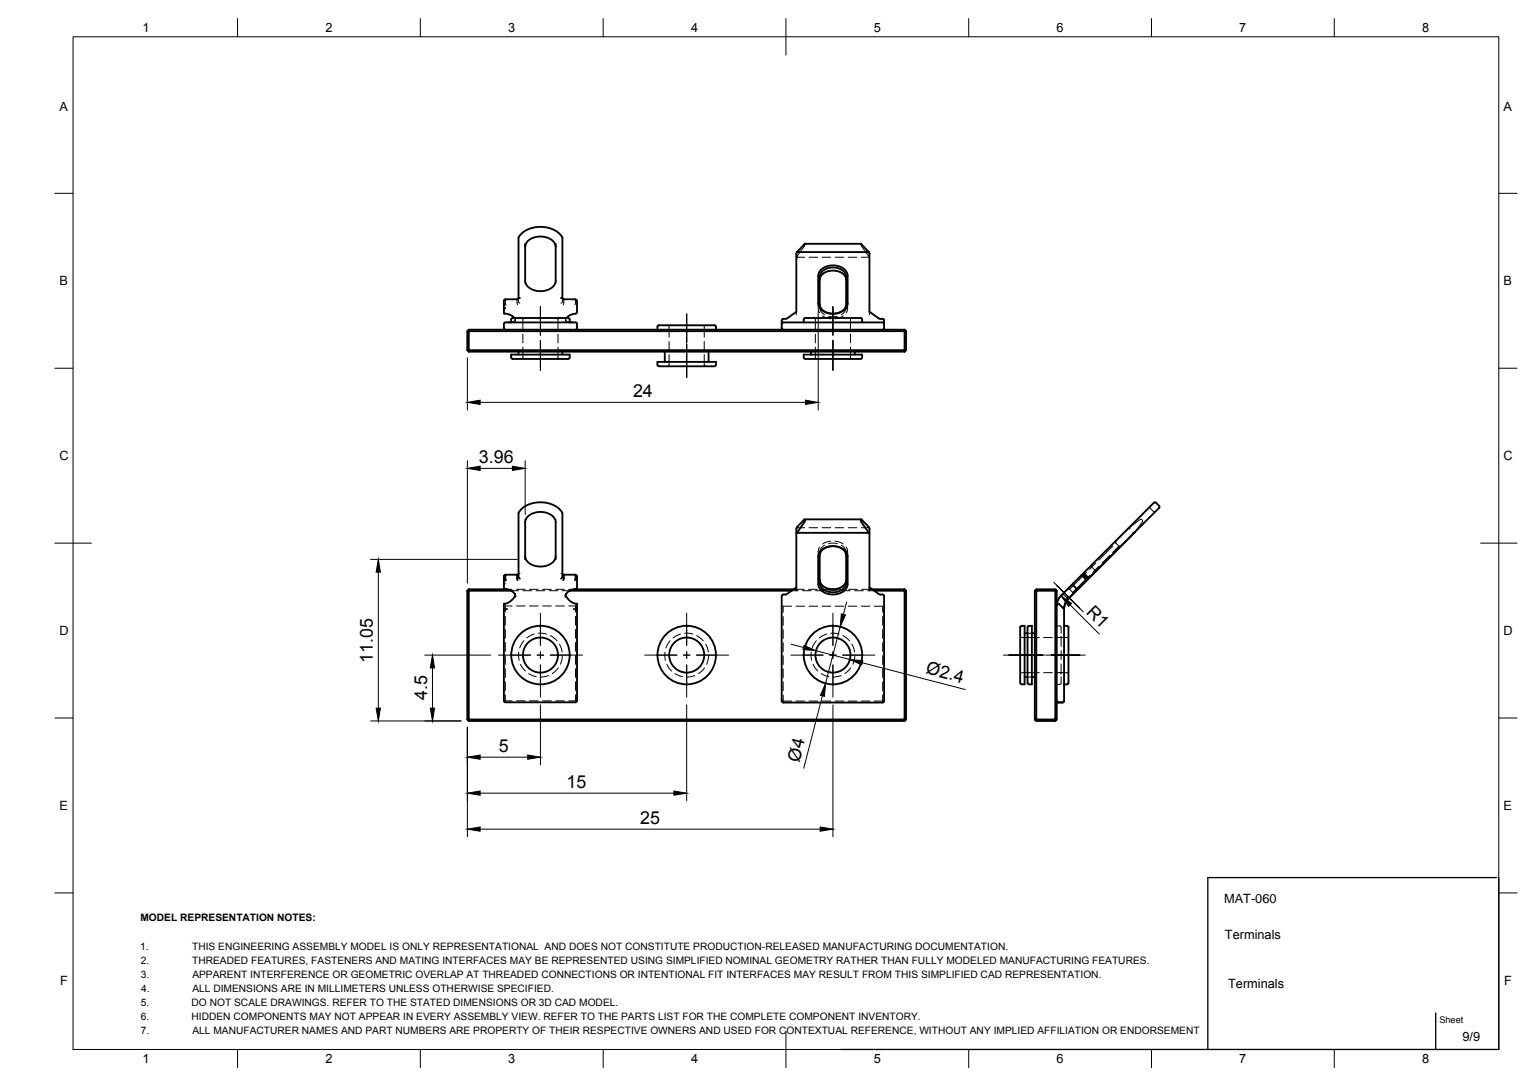
ISO-10303-21;
HEADER;
FILE_DESCRIPTION (('STEP AP214'),
    '1' );
FILE_NAME ('Terminals.step',
    '2026-10-29T23:46:56',
    ( '' ),
    ( '' ),
    'SwSTEP 2.0',
    'SolidWorks 2020',
    '' );
FILE_SCHEMA (( 'AUTOMOTIVE_DESIGN' ));
ENDSEC;

DATA;
#17=AXIS2_PLACEMENT_3D ( 'NONE', #6109, #14151, #26614 ) ;
#19=AXIS2_PLACEMENT_3D ( 'NONE', #29892, #26933, #14470 ) ;
#20=EDGE_LOOP ( 'NONE', ( #20639, #20304, #9074, #30153 ) ) ;
#22=DIRECTION ( 'NONE',  ( 7.588956326749211550E-18, -4.206627182996911684E-18, 1.000000000000000000 ) ) ;
#27=DIRECTION ( 'NONE',  ( 0.9612616959383206705, 0.2756373558169926130, 8.795445018804289444E-19 ) ) ;
#28=FACE_OUTER_BOUND ( 'NONE', #27332, .T. ) ;
#29=CARTESIAN_POINT ( 'NONE',  ( -42.41019933908752648, 14.71530103803245915, 55.14139656020049785 ) ) ;
#36=DIRECTION ( 'NONE',  ( 0.9612616959383191162, 0.2756373558169986082, 8.795445018805098335E-19 ) ) ;
#38=FACE_OUTER_BOUND ( 'NONE', #16032, .T. ) ;
#41=AXIS2_PLACEMENT_3D ( 'NONE', #1077, #13253, #30795 ) ;
#52=EDGE_LOOP ( 'NONE', ( #4319, #21732, #2975, #7082 ) ) ;
#54=CARTESIAN_POINT ( 'NONE',  ( -41.75126335834794133, 15.45321085637654690, 35.55750462089839203 ) ) ;
#56=ORIENTED_EDGE ( 'NONE', *, *, #16072, .T. ) ;
#57=CARTESIAN_POINT ( 'NONE',  ( -40.99628586177130529, 8.927770518203464789, 58.05249952744806308 ) ) ;
#66=ORIENTED_EDGE ( 'NONE', *, *, #7414, .F. ) ;
#68=FACE_OUTER_BOUND ( 'NONE', #23592, .T. ) ;
#69=CARTESIAN_POINT ( 'NONE',  ( -40.69193635511749108, 9.347952559758585522, 39.44930799450052206 ) ) ;
#72=CARTESIAN_POINT ( 'NONE',  ( -40.77849034781615956, 8.435947495041027366, 34.55508635502627612 ) ) ;
#75=CARTESIAN_POINT ( 'NONE',  ( -40.75848109938849717, 9.580021662090986823, 38.54930799450052348 ) ) ;
#76=DIRECTION ( 'NONE',  ( 0.4848096202463429982, 0.8746197071393925215, 9.920727850371698576E-18 ) ) ;
#77=ORIENTED_EDGE ( 'NONE', *, *, #10123, .F. ) ;
#82=CARTESIAN_POINT ( 'NONE',  ( -39.58809650894544774, 2.596771453999702661, 45.04930799450051637 ) ) ;
#90=VERTEX_POINT ( 'NONE', #16171 ) ;
#101=LINE ( 'NONE', #30305, #23466 ) ;
#103=ORIENTED_EDGE ( 'NONE', *, *, #27267, .F. ) ;
#108=DIRECTION ( 'NONE',  ( 0.9612616959383206705, 0.2756373558169926130, 8.795445018804289444E-19 ) ) ;
#110=VERTEX_POINT ( 'NONE', #16495 ) ;
#115=VECTOR ( 'NONE', #2052, 999.9999999999998863 ) ;
#118=SPHERICAL_SURFACE ( 'NONE', #22577, 0.1000000000000000056 ) ;
#123=EDGE_CURVE ( 'NONE', #13895, #2732, #897, .T. ) ;
#136=FACE_OUTER_BOUND ( 'NONE', #14776, .T. ) ;
#137=ORIENTED_EDGE ( 'NONE', *, *, #30547, .F. ) ;
#149=AXIS2_PLACEMENT_3D ( 'NONE', #13743, #23739, #24058 ) ;
#153=ORIENTED_EDGE ( 'NONE', *, *, #20856, .F. ) ;
#155=VERTEX_POINT ( 'NONE', #13728 ) ;
#156=CARTESIAN_POINT ( 'NONE',  ( -40.54018958231235814, 7.005332542891154368, 35.02307665165292150 ) ) ;
#158=CARTESIAN_POINT ( 'NONE',  ( -40.76199410932685652, 8.110698076655893374, 59.50788663826320146 ) ) ;
#168=VECTOR ( 'NONE', #18188, 1000.000000000000114 ) ;
#171=AXIS2_PLACEMENT_3D ( 'NONE', #9638, #108, #19631 ) ;
#175=DIRECTION ( 'NONE',  ( 0.3958453973320085195, 0.7141240004913234074, 0.5773502691896251759 ) ) ;
#179=EDGE_CURVE ( 'NONE', #22338, #15550, #10168, .T. ) ;
#180=VERTEX_POINT ( 'NONE', #22065 ) ;
#184=DIRECTION ( 'NONE',  ( 0.8746197071393858602, -0.4848096202463547666, 0.000000000000000000 ) ) ;
#187=ORIENTED_EDGE ( 'NONE', *, *, #28945, .F. ) ;
#188=AXIS2_PLACEMENT_3D ( 'NONE', #771, #25875, #3057 ) ;
#192=DIRECTION ( 'NONE',  ( -0.9612616959383207815, -0.2756373558169926685, -8.795445018804289444E-19 ) ) ;
#195=CARTESIAN_POINT ( 'NONE',  ( -42.67844523361456766, 15.18734573188464765, 35.55750462089839203 ) ) ;
#196=CIRCLE ( 'NONE', #709, 0.8928932188134561798 ) ;
#197=DIRECTION ( 'NONE',  ( -0.9612616959383183390, -0.2756373558170014948, -8.795445018805493151E-19 ) ) ;
#209=DIRECTION ( 'NONE',  ( 0.2756373558169961657, -0.9612616959383196713, -2.918609477355923238E-15 ) ) ;
#211=CARTESIAN_POINT ( 'NONE',  ( -43.29088418437023478, 1.073429008971243270, 39.44930799450052916 ) ) ;
#218=LINE ( 'NONE', #12381, #10663 ) ;
#225=ORIENTED_EDGE ( 'NONE', *, *, #23042, .T. ) ;
#229=VERTEX_POINT ( 'NONE', #19763 ) ;
#232=CARTESIAN_POINT ( 'NONE',  ( -40.60333149162104860, 7.557375771971046596, 56.04611646155296256 ) ) ;
#240=CARTESIAN_POINT ( 'NONE',  ( -40.59758774925371938, 7.567737757495682338, 34.64930799450051779 ) ) ;
#249=ORIENTED_EDGE ( 'NONE', *, *, #29875, .T. ) ;
#250=DIRECTION ( 'NONE',  ( -0.9612616959383205595, -0.2756373558169929461, 1.660411357259281952E-16 ) ) ;
#261=TOROIDAL_SURFACE ( 'NONE', #15443, 0.2000000000000000111, 0.1000000000000000056 ) ;
#271=DIRECTION ( 'NONE',  ( -0.2756373558170082672, 0.9612616959383162296, 0.000000000000000000 ) ) ;
#280=DIRECTION ( 'NONE',  ( -0.8746197071393927436, 0.4848096202463423876, 1.277302113040827440E-17 ) ) ;
#283=TOROIDAL_SURFACE ( 'NONE', #21230, 1.142135311067127068, 0.1000000000000000056 ) ;
#284=CARTESIAN_POINT ( 'NONE',  ( -40.04869510400508403, 6.988917179839018168, 35.05065200723174001 ) ) ;
#286=VERTEX_POINT ( 'NONE', #26777 ) ;
#289=ORIENTED_EDGE ( 'NONE', *, *, #14454, .T. ) ;
#290=VECTOR ( 'NONE', #23726, 1000.000000000000114 ) ;
#292=PLANE ( 'NONE',  #4320 ) ;
#301=ADVANCED_FACE ( 'NONE', ( #4126 ), #31709, .T. ) ;
#311=ORIENTED_EDGE ( 'NONE', *, *, #27048, .T. ) ;
#317=DIRECTION ( 'NONE',  ( 2.946248497964555786E-19, 3.001156285468303092E-19, 1.000000000000000000 ) ) ;
#318=CARTESIAN_POINT ( 'NONE',  ( -40.58856461370174884, 7.499380836222963254, 53.94930799450052206 ) ) ;
#328=CYLINDRICAL_SURFACE ( 'NONE', #6747, 0.1000000000000020595 ) ;
#342=DIRECTION ( 'NONE',  ( 0.4848096202463636484, 0.8746197071393810862, 0.000000000000000000 ) ) ;
#356=ORIENTED_EDGE ( 'NONE', *, *, #17245, .T. ) ;
#357=CYLINDRICAL_SURFACE ( 'NONE', #3440, 2.000000000000001776 ) ;
#361=LINE ( 'NONE', #25479, #15657 ) ;
#365=FACE_OUTER_BOUND ( 'NONE', #31359, .T. ) ;
#367=ORIENTED_EDGE ( 'NONE', *, *, #20650, .T. ) ;
#372=CYLINDRICAL_SURFACE ( 'NONE', #24107, 0.1000000000000012962 ) ;
#376=ORIENTED_EDGE ( 'NONE', *, *, #20856, .T. ) ;
#382=VERTEX_POINT ( 'NONE', #1667 ) ;
#383=LINE ( 'NONE', #20407, #27548 ) ;
#384=VECTOR ( 'NONE', #5115, 1000.000000000000114 ) ;
#390=ORIENTED_EDGE ( 'NONE', *, *, #15587, .T. ) ;
#395=CARTESIAN_POINT ( 'NONE',  ( -37.58300281841709989, 16.01180101885526597, 37.04930799450052348 ) ) ;
#400=CARTESIAN_POINT ( 'NONE',  ( -40.68422973805265030, 6.807290781432339344, 39.32248954417796227 ) ) ;
#407=EDGE_CURVE ( 'NONE', #2291, #14081, #6151, .T. ) ;
#411=ADVANCED_FACE ( 'NONE', ( #1587 ), #6674, .T. ) ;
#413=CARTESIAN_POINT ( 'NONE',  ( -40.08841711228579641, 7.575633567407562552, 60.54930799450051637 ) ) ;
#423=CARTESIAN_POINT ( 'NONE',  ( -40.11967773290336226, 9.763195579837789850, 38.54930799450052348 ) ) ;
#424=ORIENTED_EDGE ( 'NONE', *, *, #23042, .F. ) ;
#433=DIRECTION ( 'NONE',  ( -0.8746197071393805311, 0.4848096202463645921, 8.676864087101954631E-18 ) ) ;
#437=EDGE_CURVE ( 'NONE', #1880, #13059, #22878, .T. ) ;
#438=LINE ( 'NONE', #30167, #5287 ) ;
#451=CARTESIAN_POINT ( 'NONE',  ( -40.90015969217747482, 8.955334253785164123, 57.04930799450051637 ) ) ;
#452=VECTOR ( 'NONE', #29063, 1000.000000000000000 ) ;
#466=DIRECTION ( 'NONE',  ( 0.000000000000000000, 0.000000000000000000, -1.000000000000000000 ) ) ;
#471=ORIENTED_EDGE ( 'NONE', *, *, #842, .F. ) ;
#472=DIRECTION ( 'NONE',  ( -0.8746197071393926326, 0.4848096202463430537, 8.676864087101709653E-18 ) ) ;
#479=DIRECTION ( 'NONE',  ( -0.9612616959383175619, -0.2756373558170036597, -8.795445018805799373E-19 ) ) ;
#480=ORIENTED_EDGE ( 'NONE', *, *, #9764, .F. ) ;
#482=EDGE_CURVE ( 'NONE', #26626, #155, #15829, .T. ) ;
#491=AXIS2_PLACEMENT_3D ( 'NONE', #9371, #11504, #4285 ) ;
#493=ORIENTED_EDGE ( 'NONE', *, *, #32444, .F. ) ;
#495=ORIENTED_EDGE ( 'NONE', *, *, #28799, .T. ) ;
#497=CIRCLE ( 'NONE', #8889, 0.1000000000000018235 ) ;
#503=DIRECTION ( 'NONE',  ( 0.2756373558169932236, -0.9612616959383206705, 3.214564189377567398E-15 ) ) ;
#504=FACE_OUTER_BOUND ( 'NONE', #24476, .T. ) ;
#507=DIRECTION ( 'NONE',  ( -0.8746197071393926326, 0.4848096202463430537, 8.676864087101709653E-18 ) ) ;
#508=FACE_OUTER_BOUND ( 'NONE', #6579, .T. ) ;
#513=ORIENTED_EDGE ( 'NONE', *, *, #26307, .F. ) ;
#527=CARTESIAN_POINT ( 'NONE',  ( -40.19935072163752210, 7.013056605096603668, 39.22629476879045285 ) ) ;
#534=AXIS2_PLACEMENT_3D ( 'NONE', #12377, #29269, #2022 ) ;
#550=EDGE_CURVE ( 'NONE', #4992, #17225, #25775, .T. ) ;
#551=AXIS2_PLACEMENT_3D ( 'NONE', #843, #30240, #2664 ) ;
#557=CARTESIAN_POINT ( 'NONE',  ( -40.69574609830256406, 6.786514717574567257, 39.44982113259668211 ) ) ;
#560=FACE_OUTER_BOUND ( 'NONE', #13717, .T. ) ;
#561=AXIS2_PLACEMENT_3D ( 'NONE', #7178, #14738, #4059 ) ;
#563=CARTESIAN_POINT ( 'NONE',  ( -40.11286833322907341, 2.887657226147505973, 35.84930799450052064 ) ) ;
#564=DIRECTION ( 'NONE',  ( -2.779292025043186357E-18, 1.288349127009862211E-17, -1.000000000000000000 ) ) ;
#569=CARTESIAN_POINT ( 'NONE',  ( -40.29992972011127961, 7.980862958756435255, 40.07149053519532345 ) ) ;
#577=AXIS2_PLACEMENT_3D ( 'NONE', #24916, #30008, #25240 ) ;
#584=AXIS2_PLACEMENT_3D ( 'NONE', #31750, #4338, #1712 ) ;
#585=ADVANCED_FACE ( 'NONE', ( #17503 ), #25657, .T. ) ;
#586=CARTESIAN_POINT ( 'NONE',  ( -40.39697993529618714, 8.288924485351975235, 59.57859731638185963 ) ) ;
#589=EDGE_CURVE ( 'NONE', #28974, #110, #24896, .T. ) ;
#591=ORIENTED_EDGE ( 'NONE', *, *, #5712, .T. ) ;
#594=EDGE_CURVE ( 'NONE', #3250, #802, #20731, .T. ) ;
#596=CIRCLE ( 'NONE', #27333, 0.1000000000000016709 ) ;
#600=CIRCLE ( 'NONE', #24713, 1.199999999999999734 ) ;
#601=ORIENTED_EDGE ( 'NONE', *, *, #27122, .F. ) ;
#607=VERTEX_POINT ( 'NONE', #27519 ) ;
#614=CARTESIAN_POINT ( 'NONE',  ( -40.46704362897354201, 7.411062716778210380, 35.30013894732506685 ) ) ;
#615=ORIENTED_EDGE ( 'NONE', *, *, #10584, .T. ) ;
#626=EDGE_CURVE ( 'NONE', #32106, #27773, #16758, .T. ) ;
#640=DIRECTION ( 'NONE',  ( -2.779292025043186357E-18, 1.288349127009862211E-17, -1.000000000000000000 ) ) ;
#651=B_SPLINE_CURVE_WITH_KNOTS ( 'NONE', 3,
 ( #1890, #31770, #9282, #29302, #27005, #12076, #21904, #22069 ),
 .UNSPECIFIED., .F., .F.,
 ( 4, 2, 2, 4 ),
 ( 0.000000000000000000, 0.0005021167140330338053, 0.0007531750710495593816, 0.001004233428066084958 ),
 .UNSPECIFIED. ) ;
#652=DIRECTION ( 'NONE',  ( -0.9612616959383221138, -0.2756373558169876170, 0.000000000000000000 ) ) ;
#655=VERTEX_POINT ( 'NONE', #26463 ) ;
#656=DIRECTION ( 'NONE',  ( 7.588956326749211550E-18, -4.206627182996912454E-18, 1.000000000000000000 ) ) ;
#666=DIRECTION ( 'NONE',  ( 0.8746197071393925215, -0.4848096202463429982, -8.676864087101709653E-18 ) ) ;
#683=CARTESIAN_POINT ( 'NONE',  ( -43.64647580959332629, 1.256990871545142774, 53.54930799450051637 ) ) ;
#684=VECTOR ( 'NONE', #2246, 1000.000000000000000 ) ;
#685=CARTESIAN_POINT ( 'NONE',  ( -41.08785830660042393, 9.277514380576530328, 34.69072935073783981 ) ) ;
#688=CARTESIAN_POINT ( 'NONE',  ( -42.38687957179150345, 4.148162238788004608, 55.04930799450051637 ) ) ;
#697=LINE ( 'NONE', #20231, #30952 ) ;
#699=CARTESIAN_POINT ( 'NONE',  ( -43.38408989745150990, 1.111547985471239786, 60.54930799450051637 ) ) ;
#701=EDGE_LOOP ( 'NONE', ( #9890, #30769 ) ) ;
#707=EDGE_CURVE ( 'NONE', #18016, #21157, #8900, .T. ) ;
#709=AXIS2_PLACEMENT_3D ( 'NONE', #18125, #3351, #11077 ) ;
#718=DIRECTION ( 'NONE',  ( -0.1949050434465282311, 0.6797146636928673713, -0.7071067811865470176 ) ) ;
#720=DIRECTION ( 'NONE',  ( 0.000000000000000000, 0.000000000000000000, 1.000000000000000000 ) ) ;
#724=DIRECTION ( 'NONE',  ( -7.588956326749211550E-18, 4.206627182996912454E-18, -1.000000000000000000 ) ) ;
#725=ORIENTED_EDGE ( 'NONE', *, *, #20436, .T. ) ;
#728=DIRECTION ( 'NONE',  ( -0.4848096202463391680, -0.8746197071393946310, 0.000000000000000000 ) ) ;
#731=CARTESIAN_POINT ( 'NONE',  ( -40.56956524039852496, 6.944624558150293225, 39.15224832543683675 ) ) ;
#734=DIRECTION ( 'NONE',  ( -0.9612616959383221138, -0.2756373558169876170, 0.000000000000000000 ) ) ;
#743=EDGE_LOOP ( 'NONE', ( #3761, #27026, #1718, #13814 ) ) ;
#747=EDGE_CURVE ( 'NONE', #17034, #3050, #21468, .T. ) ;
#752=ADVANCED_FACE ( 'NONE', ( #26303 ), #3814, .T. ) ;
#753=AXIS2_PLACEMENT_3D ( 'NONE', #2967, #13000, #25623 ) ;
#754=ORIENTED_EDGE ( 'NONE', *, *, #20425, .F. ) ;
#771=CARTESIAN_POINT ( 'NONE',  ( -40.28779227465695811, 2.984619150196779813, 57.04930799450051637 ) ) ;
#773=FACE_OUTER_BOUND ( 'NONE', #16679, .T. ) ;
#776=EDGE_CURVE ( 'NONE', #22267, #18307, #27310, .T. ) ;
#777=VERTEX_POINT ( 'NONE', #26786 ) ;
#784=ADVANCED_FACE ( 'NONE', ( #24816 ), #9558, .T. ) ;
#786=ORIENTED_EDGE ( 'NONE', *, *, #27395, .F. ) ;
#789=ADVANCED_FACE ( 'NONE', ( #32368 ), #21852, .F. ) ;
#791=VECTOR ( 'NONE', #10665, 1000.000000000000114 ) ;
#793=DIRECTION ( 'NONE',  ( 0.000000000000000000, 0.000000000000000000, -1.000000000000000000 ) ) ;
#799=AXIS2_PLACEMENT_3D ( 'NONE', #9111, #29139, #16645 ) ;
#802=VERTEX_POINT ( 'NONE', #6762 ) ;
#804=CIRCLE ( 'NONE', #9739, 1.199999999999999734 ) ;
#805=CARTESIAN_POINT ( 'NONE',  ( -40.60722745863126448, 9.415333058485025219, 39.54930799450052348 ) ) ;
#809=EDGE_CURVE ( 'NONE', #2831, #29664, #6340, .T. ) ;
#811=CARTESIAN_POINT ( 'NONE',  ( -40.08841711228579641, 7.575633567407562552, 53.64930799450051779 ) ) ;
#813=ADVANCED_FACE ( 'NONE', ( #24319 ), #1838, .T. ) ;
#823=AXIS2_PLACEMENT_3D ( 'NONE', #3985, #9075, #29100 ) ;
#830=VECTOR ( 'NONE', #28891, 1000.000000000000000 ) ;
#831=ORIENTED_EDGE ( 'NONE', *, *, #27020, .F. ) ;
#833=CARTESIAN_POINT ( 'NONE',  ( -42.22510282758591416, 14.66434666503944051, 60.44930799450051495 ) ) ;
#839=DIRECTION ( 'NONE',  ( -0.9612616959383193382, -0.2756373558169973870, -8.795445018804928853E-19 ) ) ;
#841=CARTESIAN_POINT ( 'NONE',  ( -40.60722745863126448, 9.415333058485023443, 38.60788663826321709 ) ) ;
#842=EDGE_CURVE ( 'NONE', #16822, #14722, #27927, .T. ) ;
#843=CARTESIAN_POINT ( 'NONE',  ( -40.50720532202722524, 7.584939507552746818, 54.01510846932454513 ) ) ;
#848=EDGE_CURVE ( 'NONE', #30210, #4768, #22672, .T. ) ;
#854=DIRECTION ( 'NONE',  ( -0.2756373558170082672, 0.9612616959383162296, 0.000000000000000000 ) ) ;
#862=CARTESIAN_POINT ( 'NONE',  ( -39.58809650894544774, 2.596771453999702661, 45.54930799450051637 ) ) ;
#864=DIRECTION ( 'NONE',  ( -0.4848096202463430537, -0.8746197071393926326, -9.920727850371701658E-18 ) ) ;
#871=CARTESIAN_POINT ( 'NONE',  ( -41.07560527903737579, 9.385057823277964673, 38.64930799450052490 ) ) ;
#873=SPHERICAL_SURFACE ( 'NONE', #13622, 0.1000000000000000056 ) ;
#875=ORIENTED_EDGE ( 'NONE', *, *, #31987, .T. ) ;
#876=DIRECTION ( 'NONE',  ( 0.8746197071393926326, -0.4848096202463430537, -8.676864087101709653E-18 ) ) ;
#877=CARTESIAN_POINT ( 'NONE',  ( -39.67555847965937943, 2.645252416024337361, 45.14930799450051779 ) ) ;
#879=CARTESIAN_POINT ( 'NONE',  ( -40.13135354151336998, 6.899777549362540618, 34.56234534340313758 ) ) ;
#882=DIRECTION ( 'NONE',  ( -0.7141240004913198547, 0.3958453973320100738, -0.5773502691896283956 ) ) ;
#885=ORIENTED_EDGE ( 'NONE', *, *, #17568, .F. ) ;
#886=FACE_OUTER_BOUND ( 'NONE', #15333, .T. ) ;
#887=DIRECTION ( 'NONE',  ( 0.6184495258776567805, -0.3428121700606641120, -0.7071067811865474617 ) ) ;
#895=DIRECTION ( 'NONE',  ( -0.8746197071393926326, 0.4848096202463430537, 8.676864087101709653E-18 ) ) ;
#897=CIRCLE ( 'NONE', #5101, 0.09999999999999815981 ) ;
#898=ORIENTED_EDGE ( 'NONE', *, *, #17976, .F. ) ;
#899=AXIS2_PLACEMENT_3D ( 'NONE', #30878, #1312, #5929 ) ;
#907=ORIENTED_EDGE ( 'NONE', *, *, #16677, .T. ) ;
#909=DIRECTION ( 'NONE',  ( 2.779292025043186357E-18, -1.288349127009862211E-17, 1.000000000000000000 ) ) ;
#911=AXIS2_PLACEMENT_3D ( 'NONE', #20744, #10594, #20099 ) ;
#912=CARTESIAN_POINT ( 'NONE',  ( -40.63136629056263160, 9.462201496834364178, 35.46931185928404773 ) ) ;
#915=DIRECTION ( 'NONE',  ( -0.2756373558169954441, 0.9612616959383198934, -1.479773560108263451E-16 ) ) ;
#925=ORIENTED_EDGE ( 'NONE', *, *, #15668, .F. ) ;
#930=CYLINDRICAL_SURFACE ( 'NONE', #149, 0.1000000000000028644 ) ;
#931=EDGE_CURVE ( 'NONE', #23264, #20995, #14972, .T. ) ;
#933=EDGE_CURVE ( 'NONE', #14507, #21242, #22832, .T. ) ;
#937=AXIS2_PLACEMENT_3D ( 'NONE', #13718, #3858, #21243 ) ;
#944=DIRECTION ( 'NONE',  ( -0.3958453973319808195, -0.7141240004913296247, 0.5773502691896363892 ) ) ;
#945=ORIENTED_EDGE ( 'NONE', *, *, #16041, .F. ) ;
#948=CYLINDRICAL_SURFACE ( 'NONE', #21641, 0.1000000000000006301 ) ;
#954=DIRECTION ( 'NONE',  ( 1.188208965918165239E-16, 1.880121038077813132E-16, 1.000000000000000000 ) ) ;
#959=CARTESIAN_POINT ( 'NONE',  ( -43.64073206722599707, 1.267352857069778516, 34.64930799450052490 ) ) ;
#962=AXIS2_PLACEMENT_3D ( 'NONE', #395, #15181, #10105 ) ;
#964=DIRECTION ( 'NONE',  ( 0.9612616959383207815, 0.2756373558169926685, 8.795445018804289444E-19 ) ) ;
#967=FACE_BOUND ( 'NONE', #5368, .T. ) ;
#974=CARTESIAN_POINT ( 'NONE',  ( -41.77464577679392477, 3.808795504615564820, 61.94930799450052206 ) ) ;
#975=CARTESIAN_POINT ( 'NONE',  ( -40.59307404304409772, 7.534955414378393002, 53.83739922958098134 ) ) ;
#978=AXIS2_PLACEMENT_3D ( 'NONE', #23436, #30997, #9473 ) ;
#986=ADVANCED_FACE ( 'NONE', ( #5446, #504 ), #31042, .F. ) ;
#988=EDGE_LOOP ( 'NONE', ( #24346, #13936, #21488, #25413 ) ) ;
#990=DIRECTION ( 'NONE',  ( 0.2756373558169961657, -0.9612616959383196713, 1.479773560108262218E-16 ) ) ;
#993=ORIENTED_EDGE ( 'NONE', *, *, #1703, .F. ) ;
#998=EDGE_CURVE ( 'NONE', #28668, #3984, #20301, .T. ) ;
#1005=DIRECTION ( 'NONE',  ( -0.2756373558169945559, 0.9612616959383202264, 0.000000000000000000 ) ) ;
#1008=VECTOR ( 'NONE', #28478, 1000.000000000000000 ) ;
#1010=EDGE_LOOP ( 'NONE', ( #6505, #21848, #23375, #10940 ) ) ;
#1012=CARTESIAN_POINT ( 'NONE',  ( -40.07989290236489666, 6.890692649785590262, 39.18555621625623075 ) ) ;
#1014=CARTESIAN_POINT ( 'NONE',  ( -40.50792392543508669, 7.569031714560849444, 60.24719206080857958 ) ) ;
#1016=EDGE_CURVE ( 'NONE', #17357, #30739, #19231, .T. ) ;
#1021=ADVANCED_FACE ( 'NONE', ( #1151 ), #13482, .T. ) ;
#1022=CARTESIAN_POINT ( 'NONE',  ( -40.22018024869837660, 7.672350704644241404, 53.87859731638185679 ) ) ;
#1036=EDGE_CURVE ( 'NONE', #1567, #17902, #25780, .T. ) ;
#1041=ORIENTED_EDGE ( 'NONE', *, *, #21183, .F. ) ;
#1042=CIRCLE ( 'NONE', #18832, 1.500000000000001332 ) ;
#1043=CYLINDRICAL_SURFACE ( 'NONE', #25449, 1.199999999999999734 ) ;
#1045=CARTESIAN_POINT ( 'NONE',  ( -40.38481129770396194, 8.639635153120075017, 34.64781247685129273 ) ) ;
#1053=DIRECTION ( 'NONE',  ( 0.000000000000000000, 0.000000000000000000, 1.000000000000000000 ) ) ;
#1063=AXIS2_PLACEMENT_3D ( 'NONE', #8082, #7920, #27934 ) ;
#1067=FACE_OUTER_BOUND ( 'NONE', #17197, .T. ) ;
#1074=EDGE_CURVE ( 'NONE', #15332, #31848, #11178, .T. ) ;
#1077=CARTESIAN_POINT ( 'NONE',  ( -40.98031486389898248, 9.265261353013489298, 39.44930799450052206 ) ) ;
#1078=EDGE_LOOP ( 'NONE', ( #3257, #10108, #20186, #1551 ) ) ;
#1080=ORIENTED_EDGE ( 'NONE', *, *, #16476, .F. ) ;
#1083=EDGE_LOOP ( 'NONE', ( #28239, #21597, #8161, #3992, #26206 ) ) ;
#1085=AXIS2_PLACEMENT_3D ( 'NONE', #29474, #7145, #12406 ) ;
#1086=PLANE ( 'NONE',  #19421 ) ;
#1087=CARTESIAN_POINT ( 'NONE',  ( -41.52218637998914375, 11.15499190493234671, 37.04930799450052348 ) ) ;
#1090=VECTOR ( 'NONE', #2299, 1000.000000000000114 ) ;
#1094=VECTOR ( 'NONE', #21735, 1000.000000000000114 ) ;
#1101=AXIS2_PLACEMENT_3D ( 'NONE', #12283, #32466, #15389 ) ;
#1104=DIRECTION ( 'NONE',  ( -0.4848096202463424431, -0.8746197071393927436, 2.220446049250312588E-16 ) ) ;
#1110=EDGE_CURVE ( 'NONE', #4462, #25249, #21007, .T. ) ;
#1111=( BOUNDED_CURVE ( )  B_SPLINE_CURVE ( 3, ( #18107, #6123, #11062, #15965 ),
 .UNSPECIFIED., .F., .F. ) 
 B_SPLINE_CURVE_WITH_KNOTS ( ( 4, 4 ),
 ( 1.048273564425898918, 1.570796326794896558 ),
 .UNSPECIFIED. ) 
 CURVE ( )  GEOMETRIC_REPRESENTATION_ITEM ( )  RATIONAL_B_SPLINE_CURVE ( ( 1.000000000000000000, 0.9773766218976414066, 0.9773766218976414066, 1.000000000000000000 ) ) 
 REPRESENTATION_ITEM ( '' )  );
#1119=DIRECTION ( 'NONE',  ( -0.8746197071393858602, 0.4848096202463547666, 0.000000000000000000 ) ) ;
#1122=DIRECTION ( 'NONE',  ( -0.4848096202463636484, -0.8746197071393810862, 0.000000000000000000 ) ) ;
#1123=DIRECTION ( 'NONE',  ( -0.9612616959383205595, -0.2756373558169932236, 1.660411357259282445E-16 ) ) ;
#1125=CARTESIAN_POINT ( 'NONE',  ( -40.54828680531407770, 6.846271790121643441, 39.54930799450052348 ) ) ;
#1138=EDGE_CURVE ( 'NONE', #155, #26626, #23818, .T. ) ;
#1142=LINE ( 'NONE', #11172, #830 ) ;
#1150=ORIENTED_EDGE ( 'NONE', *, *, #15975, .T. ) ;
#1151=FACE_OUTER_BOUND ( 'NONE', #1860, .T. ) ;
#1155=CARTESIAN_POINT ( 'NONE',  ( -40.66789130039685318, 6.810915939861079238, 34.59928685681251181 ) ) ;
#1165=CARTESIAN_POINT ( 'NONE',  ( -40.23397449525940317, 6.794506605641760899, 39.54930799450052348 ) ) ;
#1170=CIRCLE ( 'NONE', #24754, 0.1000000000000011019 ) ;
#1179=DIRECTION ( 'NONE',  ( -1.431146867680865853E-17, -2.558717127065790464E-17, -1.000000000000000000 ) ) ;
#1180=ORIENTED_EDGE ( 'NONE', *, *, #4567, .T. ) ;
#1184=DIRECTION ( 'NONE',  ( 0.8746197071393926326, -0.4848096202463430537, -8.676864087101709653E-18 ) ) ;
#1187=VERTEX_POINT ( 'NONE', #1804 ) ;
#1188=DIRECTION ( 'NONE',  ( 0.8746197071393926326, -0.4848096202463430537, -8.676864087101709653E-18 ) ) ;
#1189=DIRECTION ( 'NONE',  ( 0.1949050434465272041, -0.6797146636928682595, 0.7071067811865464625 ) ) ;
#1195=CARTESIAN_POINT ( 'NONE',  ( -40.11708823821336267, 6.803395581744677401, 34.64878293746919979 ) ) ;
#1201=CARTESIAN_POINT ( 'NONE',  ( -40.13606231985500017, 7.635531802539802904, 53.64930799450051779 ) ) ;
#1202=EDGE_CURVE ( 'NONE', #5096, #18712, #24777, .T. ) ;
#1204=CARTESIAN_POINT ( 'NONE',  ( -40.02540636251513462, 2.839176264122873050, 37.04930799450052348 ) ) ;
#1213=TOROIDAL_SURFACE ( 'NONE', #10659, 0.2000000000000000111, 0.1000000000000000056 ) ;
#1216=EDGE_CURVE ( 'NONE', #21033, #23633, #1170, .T. ) ;
#1222=EDGE_LOOP ( 'NONE', ( #3505, #5373, #3575, #27729 ) ) ;
#1234=ORIENTED_EDGE ( 'NONE', *, *, #29026, .F. ) ;
#1236=DIRECTION ( 'NONE',  ( 0.7141240004913222972, -0.3958453973320028019, -0.5773502691896303940 ) ) ;
#1237=DIRECTION ( 'NONE',  ( 0.7936353835927094647, -0.4399192766786362285, -0.4202545751282172337 ) ) ;
#1238=DIRECTION ( 'NONE',  ( -0.9097384655268496711, -0.4151817967359032746, -2.820562191637069417E-18 ) ) ;
#1239=AXIS2_PLACEMENT_3D ( 'NONE', #3672, #18277, #16138 ) ;
#1244=CARTESIAN_POINT ( 'NONE',  ( -40.57119026524449623, 6.941393190192507667, 34.94194090914223949 ) ) ;
#1246=ORIENTED_EDGE ( 'NONE', *, *, #10469, .T. ) ;
#1255=AXIS2_PLACEMENT_3D ( 'NONE', #6118, #23513, #31074 ) ;
#1257=DIRECTION ( 'NONE',  ( 0.9612616959383206705, 0.2756373558169926130, 8.795445018804289444E-19 ) ) ;
#1260=CARTESIAN_POINT ( 'NONE',  ( -40.68422973805265030, 6.807290781432339344, 39.32248954417796227 ) ) ;
#1261=CARTESIAN_POINT ( 'NONE',  ( -40.50737503712689147, 7.561449354142130375, 53.83005649861389941 ) ) ;
#1265=VERTEX_POINT ( 'NONE', #20497 ) ;
#1270=CARTESIAN_POINT ( 'NONE',  ( -40.69571722278731585, 6.786566810383049209, 39.44930799450052206 ) ) ;
#1278=FACE_OUTER_BOUND ( 'NONE', #27742, .T. ) ;
#1279=DIRECTION ( 'NONE',  ( 2.779292025043186357E-18, -1.288349127009862211E-17, 1.000000000000000000 ) ) ;
#1283=AXIS2_PLACEMENT_3D ( 'NONE', #2957, #27434, #10201 ) ;
#1288=EDGE_LOOP ( 'NONE', ( #27758, #29000, #14380, #13174 ) ) ;
#1289=AXIS2_PLACEMENT_3D ( 'NONE', #1498, #12009, #32033 ) ;
#1293=EDGE_CURVE ( 'NONE', #25363, #13517, #18029, .T. ) ;
#1295=EDGE_CURVE ( 'NONE', #19780, #23334, #28946, .T. ) ;
#1298=( BOUNDED_CURVE ( )  B_SPLINE_CURVE ( 3, ( #6678, #1749, #21433, #31949 ),
 .UNSPECIFIED., .F., .F. ) 
 B_SPLINE_CURVE_WITH_KNOTS ( ( 4, 4 ),
 ( 2.001968580199905201, 2.533845118315130041 ),
 .UNSPECIFIED. ) 
 CURVE ( )  GEOMETRIC_REPRESENTATION_ITEM ( )  RATIONAL_B_SPLINE_CURVE ( ( 1.000000000000000000, 0.9765642231641245008, 0.9765642231641245008, 1.000000000000000000 ) ) 
 REPRESENTATION_ITEM ( '' )  );
#1302=CARTESIAN_POINT ( 'NONE',  ( -42.22138300640814634, 14.68176690255379491, 37.04930799450052348 ) ) ;
#1308=DIRECTION ( 'NONE',  ( -0.9612616959383200044, -0.2756373558169954996, 1.660411357259285896E-16 ) ) ;
#1310=CARTESIAN_POINT ( 'NONE',  ( -40.01185171578376298, 7.339011093366010208, 38.76026362135365844 ) ) ;
#1312=DIRECTION ( 'NONE',  ( 0.8746197071393928546, -0.4848096202463424431, -1.277302113040829905E-17 ) ) ;
#1315=CYLINDRICAL_SURFACE ( 'NONE', #22680, 0.1000000000000012962 ) ;
#1316=DIRECTION ( 'NONE',  ( 0.4848096202463429982, 0.8746197071393925215, 9.920727850371698576E-18 ) ) ;
#1317=PRESENTATION_STYLE_ASSIGNMENT (( #30729 ) ) ;
#1326=DIRECTION ( 'NONE',  ( 0.8746197071393925215, -0.4848096202463429982, -8.676864087101708112E-18 ) ) ;
#1328=VERTEX_POINT ( 'NONE', #10013 ) ;
#1329=CARTESIAN_POINT ( 'NONE',  ( -40.50735885958352611, 7.561537692508191633, 60.26824376325151889 ) ) ;
#1336=EDGE_CURVE ( 'NONE', #25136, #28530, #5568, .T. ) ;
#1345=EDGE_LOOP ( 'NONE', ( #24023, #10334, #14732, #11651 ) ) ;
#1346=DIRECTION ( 'NONE',  ( 0.9612616959383194493, 0.2756373558169974980, 8.795445018804946186E-19 ) ) ;
#1350=DIRECTION ( 'NONE',  ( 0.8746197071393926326, -0.4848096202463430537, -8.676864087101709653E-18 ) ) ;
#1351=DIRECTION ( 'NONE',  ( 0.7141240004913222972, -0.3958453973320028019, -0.5773502691896303940 ) ) ;
#1352=DIRECTION ( 'NONE',  ( -0.2756373558169932236, 0.9612616959383204485, -1.479773560108267395E-16 ) ) ;
#1354=DIRECTION ( 'NONE',  ( 0.000000000000000000, 0.000000000000000000, 1.000000000000000000 ) ) ;
#1357=CARTESIAN_POINT ( 'NONE',  ( -39.59792565122570096, 7.943629834091022524, 39.54930799450052348 ) ) ;
#1362=VECTOR ( 'NONE', #6802, 1000.000000000000114 ) ;
#1365=CARTESIAN_POINT ( 'NONE',  ( -41.40774006177731081, 10.72547736613775626, 57.28220823191252720 ) ) ;
#1368=ORIENTED_EDGE ( 'NONE', *, *, #22630, .F. ) ;
#1371=CARTESIAN_POINT ( 'NONE',  ( -40.47970302497625994, 7.463434137431150361, 53.64930799450051779 ) ) ;
#1379=ORIENTED_EDGE ( 'NONE', *, *, #26631, .F. ) ;
#1382=CARTESIAN_POINT ( 'NONE',  ( -40.75848109938849717, 9.580021662090986823, 38.54930799450052348 ) ) ;
#1386=ORIENTED_EDGE ( 'NONE', *, *, #2719, .F. ) ;
#1390=CARTESIAN_POINT ( 'NONE',  ( -40.50726676055796105, 7.559560307024983494, 60.29072935073781991 ) ) ;
#1393=EDGE_CURVE ( 'NONE', #7595, #2858, #1686, .T. ) ;
#1394=SPHERICAL_SURFACE ( 'NONE', #7627, 0.1000000000000000056 ) ;
#1396=DIRECTION ( 'NONE',  ( 0.000000000000000000, 0.000000000000000000, 1.000000000000000000 ) ) ;
#1402=DIRECTION ( 'NONE',  ( -0.8746197071393810862, 0.4848096202463637039, 8.676864087101942305E-18 ) ) ;
#1404=DIRECTION ( 'NONE',  ( -0.9612616959383207815, -0.2756373558169927795, 2.080984688351791594E-17 ) ) ;
#1409=DIRECTION ( 'NONE',  ( 0.000000000000000000, 0.000000000000000000, -1.000000000000000000 ) ) ;
#1422=EDGE_CURVE ( 'NONE', #90, #22267, #8822, .T. ) ;
#1425=DIRECTION ( 'NONE',  ( 0.4848096202463673676, 0.8746197071393789768, 0.000000000000000000 ) ) ;
#1435=CARTESIAN_POINT ( 'NONE',  ( -40.63900869798943205, 6.896661531574880044, 39.10715606024436397 ) ) ;
#1436=CARTESIAN_POINT ( 'NONE',  ( -42.47434154250544225, 4.196643200812637531, 57.04930799450051637 ) ) ;
#1441=ORIENTED_EDGE ( 'NONE', *, *, #179, .F. ) ;
#1443=ADVANCED_FACE ( 'NONE', ( #6369 ), #23288, .T. ) ;
#1446=CIRCLE ( 'NONE', #24577, 0.1000000000000018235 ) ;
#1447=CARTESIAN_POINT ( 'NONE',  ( -40.41647043964083252, 8.356895951721261540, 54.64930799450051069 ) ) ;
#1450=DIRECTION ( 'NONE',  ( 0.000000000000000000, 0.000000000000000000, -1.000000000000000000 ) ) ;
#1452=ORIENTED_EDGE ( 'NONE', *, *, #25684, .F. ) ;
#1453=DIRECTION ( 'NONE',  ( 0.2756373558169932236, -0.9612616959383205595, -1.211836997745615998E-14 ) ) ;
#1454=B_SPLINE_CURVE_WITH_KNOTS ( 'NONE', 3,
 ( #14906, #12614, #22766, #24749, #284, #20140, #30497, #30172 ),
 .UNSPECIFIED., .F., .F.,
 ( 4, 2, 2, 4 ),
 ( 4.148501517905142282E-16, 0.0002713365654423687142, 0.0005426731308843225042, 0.001085346261768216532 ),
 .UNSPECIFIED. ) ;
#1457=ORIENTED_EDGE ( 'NONE', *, *, #28527, .F. ) ;
#1458=ORIENTED_EDGE ( 'NONE', *, *, #25398, .T. ) ;
#1460=TOROIDAL_SURFACE ( 'NONE', #937, 1.299999999999999822, 0.1000000000000000056 ) ;
#1461=DIRECTION ( 'NONE',  ( 0.9612616959383198934, 0.2756373558169956106, 0.000000000000000000 ) ) ;
#1466=FACE_OUTER_BOUND ( 'NONE', #15993, .T. ) ;
#1467=VECTOR ( 'NONE', #28994, 1000.000000000000227 ) ;
#1468=CARTESIAN_POINT ( 'NONE',  ( -43.64073206722599707, 1.267352857069778960, 34.64930799450052490 ) ) ;
#1470=ORIENTED_EDGE ( 'NONE', *, *, #18966, .F. ) ;
#1472=ADVANCED_FACE ( 'NONE', ( #3419 ), #26855, .T. ) ;
#1475=CARTESIAN_POINT ( 'NONE',  ( -37.49824857498671093, 12.70128680827697387, 57.95249952744806166 ) ) ;
#1480=EDGE_LOOP ( 'NONE', ( #25592, #24123, #29450, #23747, #16266, #20918 ) ) ;
#1491=AXIS2_PLACEMENT_3D ( 'NONE', #13784, #18527, #23779 ) ;
#1493=AXIS2_PLACEMENT_3D ( 'NONE', #20507, #7402, #30208 ) ;
#1494=( BOUNDED_CURVE ( )  B_SPLINE_CURVE ( 3, ( #32024, #1823, #2317, #16914 ),
 .UNSPECIFIED., .F., .F. ) 
 B_SPLINE_CURVE_WITH_KNOTS ( ( 4, 4 ),
 ( 4.712388980384723425, 5.497787143782102426 ),
 .UNSPECIFIED. ) 
 CURVE ( )  GEOMETRIC_REPRESENTATION_ITEM ( )  RATIONAL_B_SPLINE_CURVE ( ( 1.000000000000000000, 0.9492530216742000038, 0.9492530216742000038, 1.000000000000000000 ) ) 
 REPRESENTATION_ITEM ( '' )  );
#1498=CARTESIAN_POINT ( 'NONE',  ( -39.64148344771002286, 7.657122216028890982, 61.94930799450052206 ) ) ;
#1500=CARTESIAN_POINT ( 'NONE',  ( -40.67014616567488616, 6.832698218566654269, 34.86215755014509909 ) ) ;
#1512=EDGE_CURVE ( 'NONE', #14722, #4736, #3326, .T. ) ;
#1513=ADVANCED_FACE ( 'NONE', ( #9149 ), #11780, .T. ) ;
#1521=VECTOR ( 'NONE', #32016, 1000.000000000000000 ) ;
#1529=CARTESIAN_POINT ( 'NONE',  ( -40.46271621608484281, 3.081581074246049212, 57.04930799450051637 ) ) ;
#1542=DIRECTION ( 'NONE',  ( 0.8746197071393926326, -0.4848096202463430537, -8.676864087101709653E-18 ) ) ;
#1544=DIRECTION ( 'NONE',  ( 0.4848096202463424431, 0.8746197071393927436, -2.220446049250312588E-16 ) ) ;
#1546=VERTEX_POINT ( 'NONE', #29669 ) ;
#1550=EDGE_CURVE ( 'NONE', #1830, #10311, #6857, .T. ) ;
#1551=ORIENTED_EDGE ( 'NONE', *, *, #30547, .T. ) ;
#1554=CARTESIAN_POINT ( 'NONE',  ( -40.41647043964083252, 8.356895951721259763, 54.44930799450051495 ) ) ;
#1555=( NAMED_UNIT ( * ) PLANE_ANGLE_UNIT ( ) SI_UNIT ( $, .RADIAN. ) );
#1557=AXIS2_PLACEMENT_3D ( 'NONE', #8265, #28289, #5810 ) ;
#1558=ORIENTED_EDGE ( 'NONE', *, *, #7947, .T. ) ;
#1565=CARTESIAN_POINT ( 'NONE',  ( -40.18126594841540822, 7.055686659393786364, 34.94323797956834454 ) ) ;
#1567=VERTEX_POINT ( 'NONE', #7175 ) ;
#1576=AXIS2_PLACEMENT_3D ( 'NONE', #20462, #28021, #8318 ) ;
#1577=TOROIDAL_SURFACE ( 'NONE', #26742, 1.524998423334081643, 0.1000000000000000056 ) ;
#1581=AXIS2_PLACEMENT_3D ( 'NONE', #4798, #14977, #16932 ) ;
#1582=EDGE_CURVE ( 'NONE', #18712, #25136, #9969, .T. ) ;
#1584=CIRCLE ( 'NONE', #16870, 0.09999999999999978351 ) ;
#1586=VERTEX_POINT ( 'NONE', #22759 ) ;
#1587=FACE_OUTER_BOUND ( 'NONE', #8169, .T. ) ;
#1588=CARTESIAN_POINT ( 'NONE',  ( -40.69193635511749108, 9.347952559758583746, 39.44930799450052206 ) ) ;
#1602=CARTESIAN_POINT ( 'NONE',  ( -40.68074350590692490, 6.811995273159344499, 39.41969944873108744 ) ) ;
#1609=DIRECTION ( 'NONE',  ( 0.9612616959383205595, 0.2756373558169931681, -1.660411357259282445E-16 ) ) ;
#1610=DIRECTION ( 'NONE',  ( -0.8746197071393926326, 0.4848096202463430537, 8.676864087101709653E-18 ) ) ;
#1611=VECTOR ( 'NONE', #3459, 1000.000000000000114 ) ;
#1614=CARTESIAN_POINT ( 'NONE',  ( -40.51565501380215295, 9.065589196111961456, 56.04611646155296256 ) ) ;
#1615=ORIENTED_EDGE ( 'NONE', *, *, #25392, .F. ) ;
#1617=EDGE_CURVE ( 'NONE', #26367, #2133, #27487, .T. ) ;
#1622=EDGE_LOOP ( 'NONE', ( #2552, #10221, #21109 ) ) ;
#1626=EDGE_CURVE ( 'NONE', #3661, #31739, #30026, .T. ) ;
#1630=FACE_OUTER_BOUND ( 'NONE', #22733, .T. ) ;
#1631=DIRECTION ( 'NONE',  ( -0.3958453973319808195, -0.7141240004913296247, -0.5773502691896363892 ) ) ;
#1634=CARTESIAN_POINT ( 'NONE',  ( -43.90780810587784089, -0.03953120679776400692, 62.04930799450052348 ) ) ;
#1635=CARTESIAN_POINT ( 'NONE',  ( -40.57861772207635198, 7.624524047285945905, 60.14124254659545699 ) ) ;
#1639=VERTEX_POINT ( 'NONE', #5206 ) ;
#1641=LINE ( 'NONE', #1475, #10773 ) ;
#1643=CIRCLE ( 'NONE', #21059, 0.1000000000000007688 ) ;
#1644=DIRECTION ( 'NONE',  ( 0.9612616959383194493, 0.2756373558169974980, 8.795445018804946186E-19 ) ) ;
#1648=EDGE_LOOP ( 'NONE', ( #4268, #16046, #1915, #601, #20806, #11239, #20230, #2720, #2294, #16738, #10326, #17722, #18135, #11663 ) ) ;
#1651=CYLINDRICAL_SURFACE ( 'NONE', #17206, 1.199999999999999734 ) ;
#1653=ORIENTED_EDGE ( 'NONE', *, *, #13052, .F. ) ;
#1662=EDGE_CURVE ( 'NONE', #14460, #7845, #17435, .T. ) ;
#1666=CIRCLE ( 'NONE', #5885, 0.1000000000000018235 ) ;
#1667=CARTESIAN_POINT ( 'NONE',  ( -41.23380787120766655, 11.23768311167744294, 38.09144330556765112 ) ) ;
#1668=DIRECTION ( 'NONE',  ( -0.6184495258776567805, 0.3428121700606641120, 0.7071067811865474617 ) ) ;
#1669=CARTESIAN_POINT ( 'NONE',  ( -40.61197514715824752, 6.966360136513624290, 35.08795977352291118 ) ) ;
#1673=LINE ( 'NONE', #8899, #26101 ) ;
#1676=DIRECTION ( 'NONE',  ( 0.1949050434465325055, -0.6797146636928671493, 0.7071067811865460184 ) ) ;
#1677=DIRECTION ( 'NONE',  ( 0.8746197071393926326, -0.4848096202463430537, -8.676864087101709653E-18 ) ) ;
#1678=FACE_BOUND ( 'NONE', #7087, .T. ) ;
#1685=DIRECTION ( 'NONE',  ( 0.9612616959383221138, 0.2756373558169876170, 0.000000000000000000 ) ) ;
#1686=CIRCLE ( 'NONE', #17409, 0.09999999999999795164 ) ;
#1688=CARTESIAN_POINT ( 'NONE',  ( -41.07644103349281295, 9.237697617431788188, 34.64930799450051779 ) ) ;
#1693=CARTESIAN_POINT ( 'NONE',  ( -42.22138300640814634, 14.68176690255379313, 36.00717268343339583 ) ) ;
#1698=LINE ( 'NONE', #6468, #5751 ) ;
#1703=EDGE_CURVE ( 'NONE', #22782, #13582, #17947, .T. ) ;
#1710=AXIS2_PLACEMENT_3D ( 'NONE', #9678, #29704, #7209 ) ;
#1712=DIRECTION ( 'NONE',  ( -0.2756373558170082672, 0.9612616959383162296, 0.000000000000000000 ) ) ;
#1715=DIRECTION ( 'NONE',  ( -0.1949050434465267878, 0.6797146636928665941, -0.7071067811865480168 ) ) ;
#1718=ORIENTED_EDGE ( 'NONE', *, *, #12170, .T. ) ;
#1720=ORIENTED_EDGE ( 'NONE', *, *, #11473, .F. ) ;
#1722=CARTESIAN_POINT ( 'NONE',  ( -40.23971823762673239, 6.784144620117122493, 53.54930799450051637 ) ) ;
#1724=DIRECTION ( 'NONE',  ( 0.8746197071393925215, -0.4848096202463429982, -8.676864087101708112E-18 ) ) ;
#1726=( NAMED_UNIT ( * ) SI_UNIT ( $, .STERADIAN. ) SOLID_ANGLE_UNIT ( ) );
#1736=ORIENTED_EDGE ( 'NONE', *, *, #28675, .T. ) ;
#1742=VECTOR ( 'NONE', #28385, 1000.000000000000000 ) ;
#1743=ORIENTED_EDGE ( 'NONE', *, *, #5029, .F. ) ;
#1745=EDGE_CURVE ( 'NONE', #2754, #8819, #23410, .T. ) ;
#1747=TOROIDAL_SURFACE ( 'NONE', #3839, 1.100000000000000089, 0.1000000000000000056 ) ;
#1749=CARTESIAN_POINT ( 'NONE',  ( -41.91799733298572761, 13.87669230940966969, 54.58433102282629079 ) ) ;
#1761=CARTESIAN_POINT ( 'NONE',  ( -42.12525683681430877, 14.70933063813549424, 37.04930799450052348 ) ) ;
#1764=VERTEX_POINT ( 'NONE', #15694 ) ;
#1767=FACE_OUTER_BOUND ( 'NONE', #3133, .T. ) ;
#1774=VERTEX_POINT ( 'NONE', #18309 ) ;
#1777=EDGE_CURVE ( 'NONE', #29734, #15549, #28017, .T. ) ;
#1789=VECTOR ( 'NONE', #16656, 1000.000000000000000 ) ;
#1792=ORIENTED_EDGE ( 'NONE', *, *, #16762, .F. ) ;
#1797=VECTOR ( 'NONE', #18419, 1000.000000000000114 ) ;
#1799=CARTESIAN_POINT ( 'NONE',  ( -43.68921302925062378, 1.179890886355840163, 39.54930799450052348 ) ) ;
#1802=ORIENTED_EDGE ( 'NONE', *, *, #6040, .T. ) ;
#1803=VERTEX_POINT ( 'NONE', #28179 ) ;
#1804=CARTESIAN_POINT ( 'NONE',  ( -40.61178118339597631, 9.038025460530262123, 56.14611646155296398 ) ) ;
#1805=ORIENTED_EDGE ( 'NONE', *, *, #30808, .T. ) ;
#1812=VERTEX_POINT ( 'NONE', #5865 ) ;
#1814=FACE_OUTER_BOUND ( 'NONE', #2795, .T. ) ;
#1823=CARTESIAN_POINT ( 'NONE',  ( -40.61463551858321352, 9.441168033762322054, 39.41901908761455786 ) ) ;
#1824=DIRECTION ( 'NONE',  ( -0.1949050434465283144, 0.6797146636928674823, 0.7071067811865467956 ) ) ;
#1826=AXIS2_PLACEMENT_3D ( 'NONE', #16899, #16723, #19189 ) ;
#1829=AXIS2_PLACEMENT_3D ( 'NONE', #31153, #1104, #26213 ) ;
#1830=VERTEX_POINT ( 'NONE', #15865 ) ;
#1833=CARTESIAN_POINT ( 'NONE',  ( -40.18454328187963398, 7.548069831825862330, 60.44930799450051495 ) ) ;
#1838=PLANE ( 'NONE',  #31511 ) ;
#1843=CARTESIAN_POINT ( 'NONE',  ( -41.13768170161382898, 11.26524684725914227, 37.04930799450052348 ) ) ;
#1853=AXIS2_PLACEMENT_3D ( 'NONE', #9106, #4179, #24201 ) ;
#1854=MANIFOLD_SOLID_BREP ( 'Stock-MAT-060-1', #25227 ) ;
#1855=CARTESIAN_POINT ( 'NONE',  ( -36.76418579970419387, 10.14130568307076352, 57.04930799450051637 ) ) ;
#1858=DIRECTION ( 'NONE',  ( -0.9612616959383200044, -0.2756373558169954996, 1.660411357259285896E-16 ) ) ;
#1860=EDGE_LOOP ( 'NONE', ( #4335, #9255, #17864, #29112 ) ) ;
#1862=DIRECTION ( 'NONE',  ( 0.8746197071393926326, -0.4848096202463430537, -8.676864087101709653E-18 ) ) ;
#1865=CARTESIAN_POINT ( 'NONE',  ( -42.66751614955960292, 15.14923148629343430, 38.44930799450052206 ) ) ;
#1871=CIRCLE ( 'NONE', #823, 1.300000000000002487 ) ;
#1872=CIRCLE ( 'NONE', #30188, 1.003191532947552256 ) ;
#1876=DIRECTION ( 'NONE',  ( -0.2530443915477144645, 0.8824706660164548522, 0.3965022818682404915 ) ) ;
#1879=DIRECTION ( 'NONE',  ( 0.9612616959383221138, 0.2756373558169876170, 0.000000000000000000 ) ) ;
#1880=VERTEX_POINT ( 'NONE', #21406 ) ;
#1883=CARTESIAN_POINT ( 'NONE',  ( -40.66881382964710667, 6.810455744988438198, 39.49839327164657732 ) ) ;
#1884=VERTEX_POINT ( 'NONE', #9113 ) ;
#1889=DIRECTION ( 'NONE',  ( 0.2756373558169954441, -0.9612616959383198934, 1.479773560108263451E-16 ) ) ;
#1890=CARTESIAN_POINT ( 'NONE',  ( -40.16503835899720087, 7.510440877657817538, 35.29832907986742185 ) ) ;
#1895=CARTESIAN_POINT ( 'NONE',  ( -40.23847961986563604, 6.935107571023904960, 34.63435542749680707 ) ) ;
#1897=EDGE_LOOP ( 'NONE', ( #19194, #19505 ) ) ;
#1898=DIRECTION ( 'NONE',  ( -0.8746197071393858602, 0.4848096202463547666, 0.000000000000000000 ) ) ;
#1899=VECTOR ( 'NONE', #10554, 1000.000000000000114 ) ;
#1903=ORIENTED_EDGE ( 'NONE', *, *, #12814, .T. ) ;
#1905=VERTEX_POINT ( 'NONE', #29472 ) ;
#1906=PLANE ( 'NONE',  #19818 ) ;
#1908=ORIENTED_EDGE ( 'NONE', *, *, #6557, .F. ) ;
#1909=ORIENTED_EDGE ( 'NONE', *, *, #24067, .T. ) ;
#1913=PLANE ( 'NONE',  #3302 ) ;
#1915=ORIENTED_EDGE ( 'NONE', *, *, #16110, .T. ) ;
#1925=DIRECTION ( 'NONE',  ( -0.4848096202463645921, -0.8746197071393805311, 0.000000000000000000 ) ) ;
#1926=EDGE_CURVE ( 'NONE', #18455, #2485, #10046, .T. ) ;
#1929=EDGE_CURVE ( 'NONE', #26389, #3234, #9006, .T. ) ;
#1932=EDGE_CURVE ( 'NONE', #24691, #28859, #24532, .T. ) ;
#1936=CARTESIAN_POINT ( 'NONE',  ( -36.59542768321662720, 12.56771722797891400, 37.04930799450052348 ) ) ;
#1943=AXIS2_PLACEMENT_3D ( 'NONE', #31975, #9495, #19493 ) ;
#1944=ORIENTED_EDGE ( 'NONE', *, *, #2599, .T. ) ;
#1950=DIRECTION ( 'NONE',  ( 0.000000000000000000, 0.000000000000000000, -1.000000000000000000 ) ) ;
#1953=VECTOR ( 'NONE', #28095, 999.9999999999998863 ) ;
#1968=EDGE_CURVE ( 'NONE', #4559, #29013, #12874, .T. ) ;
#1970=ORIENTED_EDGE ( 'NONE', *, *, #13537, .F. ) ;
#1973=CARTESIAN_POINT ( 'NONE',  ( -40.90015969217747482, 8.955334253785164123, 57.04930799450051637 ) ) ;
#1974=LINE ( 'NONE', #9699, #15157 ) ;
#1978=ORIENTED_EDGE ( 'NONE', *, *, #18415, .F. ) ;
#1982=ADVANCED_FACE ( 'NONE', ( #11582 ), #9775, .F. ) ;
#1983=CIRCLE ( 'NONE', #27669, 0.1000000000000006301 ) ;
#1988=VECTOR ( 'NONE', #29349, 1000.000000000000114 ) ;
#1990=CARTESIAN_POINT ( 'NONE',  ( -43.86882709718853590, -0.1754741395363378920, 32.14930799450051779 ) ) ;
#1993=EDGE_CURVE ( 'NONE', #12799, #21428, #12734, .T. ) ;
#1994=CIRCLE ( 'NONE', #8809, 0.1000000000000028644 ) ;
#1998=CARTESIAN_POINT ( 'NONE',  ( -43.69495677161796010, 1.169528900831203311, 60.44930799450051495 ) ) ;
#2002=CARTESIAN_POINT ( 'NONE',  ( -43.68921302925062378, 1.179890886355840163, 39.54930799450052348 ) ) ;
#2011=CARTESIAN_POINT ( 'NONE',  ( -40.41702379479729501, 8.543002789739318814, 34.55838508629864947 ) ) ;
#2017=DIRECTION ( 'NONE',  ( 0.4848096202463484938, 0.8746197071393896350, -2.220446049250314067E-16 ) ) ;
#2022=DIRECTION ( 'NONE',  ( 0.000000000000000000, 0.000000000000000000, -1.000000000000000000 ) ) ;
#2024=CARTESIAN_POINT ( 'NONE',  ( -39.58809650894544774, 2.596771453999702661, 47.04930799450051637 ) ) ;
#2030=ADVANCED_FACE ( 'NONE', ( #10267 ), #15024, .T. ) ;
#2033=DIRECTION ( 'NONE',  ( -0.2756373558169947779, 0.9612616959383200044, 0.000000000000000000 ) ) ;
#2034=EDGE_CURVE ( 'NONE', #8765, #30210, #25027, .T. ) ;
#2051=CARTESIAN_POINT ( 'NONE',  ( -41.04685960816998147, 9.497330455345890599, 38.54930799450052348 ) ) ;
#2052=DIRECTION ( 'NONE',  ( -0.9097384655268497822, -0.4151817967359032191, -2.820562191637069417E-18 ) ) ;
#2056=ORIENTED_EDGE ( 'NONE', *, *, #22974, .T. ) ;
#2059=ORIENTED_EDGE ( 'NONE', *, *, #18153, .T. ) ;
#2063=PLANE ( 'NONE',  #31594 ) ;
#2065=ORIENTED_EDGE ( 'NONE', *, *, #19663, .T. ) ;
#2069=AXIS2_PLACEMENT_3D ( 'NONE', #26157, #11550, #15989 ) ;
#2077=CARTESIAN_POINT ( 'NONE',  ( -40.13606231985500017, 7.635531802539802015, 60.54930799450051637 ) ) ;
#2081=CARTESIAN_POINT ( 'NONE',  ( -36.21250238186772208, 8.895094119121829124, 53.80788663826320573 ) ) ;
#2084=ORIENTED_EDGE ( 'NONE', *, *, #28084, .T. ) ;
#2087=DIRECTION ( 'NONE',  ( 0.9612616959383127879, 0.2756373558170205351, 1.210030619774134952E-14 ) ) ;
#2092=DIRECTION ( 'NONE',  ( 0.8746197071393925215, -0.4848096202463429982, -8.676864087101708112E-18 ) ) ;
#2098=CIRCLE ( 'NONE', #24716, 0.1000000000000014905 ) ;
#2099=DIRECTION ( 'NONE',  ( 0.2756373558170082672, -0.9612616959383162296, 0.000000000000000000 ) ) ;
#2102=LINE ( 'NONE', #14423, #15595 ) ;
#2106=ORIENTED_EDGE ( 'NONE', *, *, #1295, .F. ) ;
#2114=ADVANCED_FACE ( 'NONE', ( #560 ), #23211, .F. ) ;
#2116=TOROIDAL_SURFACE ( 'NONE', #10523, 1.524998423334081643, 0.1000000000000000056 ) ;
#2132=CIRCLE ( 'NONE', #31519, 1.042135311067126979 ) ;
#2133=VERTEX_POINT ( 'NONE', #20742 ) ;
#2134=CARTESIAN_POINT ( 'NONE',  ( -40.49360782792987123, 7.147293204394357780, 35.15590551817737008 ) ) ;
#2135=FACE_OUTER_BOUND ( 'NONE', #26216, .T. ) ;
#2143=DIRECTION ( 'NONE',  ( 0.000000000000000000, 0.000000000000000000, -1.000000000000000000 ) ) ;
#2148=CIRCLE ( 'NONE', #28885, 0.1000000000000006301 ) ;
#2153=AXIS2_PLACEMENT_3D ( 'NONE', #11898, #18942, #21895 ) ;
#2160=ORIENTED_EDGE ( 'NONE', *, *, #31987, .F. ) ;
#2161=ADVANCED_FACE ( 'NONE', ( #28145 ), #8119, .T. ) ;
#2170=VECTOR ( 'NONE', #280, 1000.000000000000227 ) ;
#2179=ORIENTED_EDGE ( 'NONE', *, *, #10545, .T. ) ;
#2180=DIRECTION ( 'NONE',  ( 0.000000000000000000, 0.000000000000000000, -1.000000000000000000 ) ) ;
#2181=CARTESIAN_POINT ( 'NONE',  ( -40.40343367063677249, 8.556671693759611230, 34.56793150177820451 ) ) ;
#2185=VERTEX_POINT ( 'NONE', #23370 ) ;
#2191=CARTESIAN_POINT ( 'NONE',  ( -40.11096502192367552, 6.858424625636979854, 39.50614098478442315 ) ) ;
#2202=ADVANCED_FACE ( 'NONE', ( #5648 ), #21568, .T. ) ;
#2209=ORIENTED_EDGE ( 'NONE', *, *, #15227, .F. ) ;
#2212=DIRECTION ( 'NONE',  ( 2.779292025043186357E-18, -1.288349127009862211E-17, 1.000000000000000000 ) ) ;
#2213=AXIS2_PLACEMENT_3D ( 'NONE', #15394, #27549, #23100 ) ;
#2214=EDGE_CURVE ( 'NONE', #31154, #24996, #28410, .T. ) ;
#2216=CARTESIAN_POINT ( 'NONE',  ( -40.68134976037170247, 6.801398876102698665, 39.48202140826487039 ) ) ;
#2220=CARTESIAN_POINT ( 'NONE',  ( -42.21195563036362586, 4.051200314738734320, 57.04930799450051637 ) ) ;
#2230=EDGE_CURVE ( 'NONE', #2858, #3439, #19942, .T. ) ;
#2231=AXIS2_PLACEMENT_3D ( 'NONE', #13331, #839, #8554 ) ;
#2235=AXIS2_PLACEMENT_3D ( 'NONE', #7426, #28093, #26096 ) ;
#2236=AXIS2_PLACEMENT_3D ( 'NONE', #31647, #8988, #24078 ) ;
#2246=DIRECTION ( 'NONE',  ( 0.2756373558169973870, -0.9612616959383193382, -1.315048337272770280E-17 ) ) ;
#2248=EDGE_CURVE ( 'NONE', #4768, #9952, #1584, .T. ) ;
#2255=EDGE_LOOP ( 'NONE', ( #24827, #13187, #8431, #1234 ) ) ;
#2257=DIRECTION ( 'NONE',  ( 1.188208965918165239E-16, 1.880121038077813132E-16, 1.000000000000000000 ) ) ;
#2260=CARTESIAN_POINT ( 'NONE',  ( -40.59783130604490253, 7.538194345349022996, 60.10545738969978657 ) ) ;
#2265=CARTESIAN_POINT ( 'NONE',  ( -41.94956971822180947, 3.905757428664828890, 48.94930799450051495 ) ) ;
#2271=EDGE_CURVE ( 'NONE', #6626, #25934, #27412, .T. ) ;
#2274=ORIENTED_EDGE ( 'NONE', *, *, #22337, .T. ) ;
#2284=CARTESIAN_POINT ( 'NONE',  ( -40.69193635511749108, 9.347952559758585522, 39.44930799450052206 ) ) ;
#2285=DIRECTION ( 'NONE',  ( 0.9612616959383207815, 0.2756373558169926685, 8.795445018804289444E-19 ) ) ;
#2291=VERTEX_POINT ( 'NONE', #15100 ) ;
#2294=ORIENTED_EDGE ( 'NONE', *, *, #13052, .T. ) ;
#2295=CARTESIAN_POINT ( 'NONE',  ( -40.50410981870283678, 7.604537000166496696, 35.33853321918559232 ) ) ;
#2296=DIRECTION ( 'NONE',  ( -0.2756373558169973870, 0.9612616959383193382, 1.315048337272770435E-17 ) ) ;
#2297=CARTESIAN_POINT ( 'NONE',  ( -40.69423955692155204, 6.789232590171223158, 34.67341590623290415 ) ) ;
#2299=DIRECTION ( 'NONE',  ( -0.9612616959383205595, -0.2756373558169931681, 1.660411357259282445E-16 ) ) ;
#2304=CARTESIAN_POINT ( 'NONE',  ( -42.33363892739273382, 14.73725438281773847, 58.96402370174222085 ) ) ;
#2305=LINE ( 'NONE', #9697, #452 ) ;
#2310=EDGE_CURVE ( 'NONE', #12604, #19419, #3241, .T. ) ;
#2317=CARTESIAN_POINT ( 'NONE',  ( -40.63136629056263160, 9.462201496834369507, 39.42930412971698217 ) ) ;
#2319=VERTEX_POINT ( 'NONE', #5069 ) ;
#2323=CARTESIAN_POINT ( 'NONE',  ( -41.08785830660042393, 9.277514380576530328, 34.69072935073783981 ) ) ;
#2327=VECTOR ( 'NONE', #6599, 1000.000000000000114 ) ;
#2331=ADVANCED_FACE ( 'NONE', ( #5088 ), #8204, .T. ) ;
#2332=CARTESIAN_POINT ( 'NONE',  ( -42.73182147790732444, -0.8057266458565844891, 61.94930799450052206 ) ) ;
#2333=DIRECTION ( 'NONE',  ( -0.4848096202463673121, -0.8746197071393789768, 0.000000000000000000 ) ) ;
#2335=DIRECTION ( 'NONE',  ( -0.9097384655268497822, -0.4151817967359032191, -2.820562191637069803E-18 ) ) ;
#2339=CARTESIAN_POINT ( 'NONE',  ( -40.58388821705207761, 6.836049376365832764, 39.54676951983897482 ) ) ;
#2341=EDGE_LOOP ( 'NONE', ( #4125, #591, #7956, #5863 ) ) ;
#2352=DIRECTION ( 'NONE',  ( -0.4848096202463432203, -0.8746197071393924105, -9.920727850371698576E-18 ) ) ;
#2356=DIRECTION ( 'NONE',  ( 0.8746197071393925215, -0.4848096202463429982, -8.676864087101708112E-18 ) ) ;
#2358=EDGE_CURVE ( 'NONE', #19852, #10175, #31112, .T. ) ;
#2361=AXIS2_PLACEMENT_3D ( 'NONE', #2640, #32194, #175 ) ;
#2364=CIRCLE ( 'NONE', #2885, 0.09999999999999795164 ) ;
#2368=DIRECTION ( 'NONE',  ( 0.2756373558169961102, -0.9612616959383197823, 0.000000000000000000 ) ) ;
#2369=ORIENTED_EDGE ( 'NONE', *, *, #31211, .T. ) ;
#2371=( BOUNDED_CURVE ( )  B_SPLINE_CURVE ( 3, ( #7988, #13550, #13400, #3525 ),
 .UNSPECIFIED., .F., .F. ) 
 B_SPLINE_CURVE_WITH_KNOTS ( ( 4, 4 ),
 ( 4.712388980384693227, 6.283185307179583567 ),
 .UNSPECIFIED. ) 
 CURVE ( )  GEOMETRIC_REPRESENTATION_ITEM ( )  RATIONAL_B_SPLINE_CURVE ( ( 1.000000000000000000, 0.8047378541243658256, 0.8047378541243658256, 1.000000000000000000 ) ) 
 REPRESENTATION_ITEM ( '' )  );
#2373=DIRECTION ( 'NONE',  ( 0.9612616959383198934, 0.2756373558169958327, 1.367252280957423978E-15 ) ) ;
#2374=CIRCLE ( 'NONE', #7609, 1.142135311067127512 ) ;
#2375=ADVANCED_FACE ( 'NONE', ( #3584 ), #9623, .T. ) ;
#2376=AXIS2_PLACEMENT_3D ( 'NONE', #32094, #11579, #21574 ) ;
#2378=CIRCLE ( 'NONE', #28592, 1.199999999999999734 ) ;
#2379=EDGE_LOOP ( 'NONE', ( #32400, #27308 ) ) ;
#2380=CARTESIAN_POINT ( 'NONE',  ( -40.74365851677129768, 8.439942589813739460, 34.54930799450052348 ) ) ;
#2391=ORIENTED_EDGE ( 'NONE', *, *, #4341, .T. ) ;
#2405=AXIS2_PLACEMENT_3D ( 'NONE', #30954, #8619, #21237 ) ;
#2408=EDGE_CURVE ( 'NONE', #23152, #30572, #16379, .T. ) ;
#2410=VERTEX_POINT ( 'NONE', #31491 ) ;
#2412=LINE ( 'NONE', #12429, #29320 ) ;
#2414=LINE ( 'NONE', #22260, #684 ) ;
#2417=DIRECTION ( 'NONE',  ( -0.9612616959383194493, -0.2756373558169974980, -8.795445018804946186E-19 ) ) ;
#2421=DIRECTION ( 'NONE',  ( 0.1949050434465355863, -0.6797146636928657060, 0.7071067811865464625 ) ) ;
#2422=PRODUCT_DEFINITION_FORMATION_WITH_SPECIFIED_SOURCE ( 'ANY', '', #14546, .NOT_KNOWN. ) ;
#2423=ORIENTED_EDGE ( 'NONE', *, *, #7011, .F. ) ;
#2425=DIRECTION ( 'NONE',  ( 0.1949050434465264547, -0.6797146636928678154, 0.7071067811865470176 ) ) ;
#2431=VERTEX_POINT ( 'NONE', #1125 ) ;
#2442=EDGE_CURVE ( 'NONE', #22267, #8364, #13818, .T. ) ;
#2451=VERTEX_POINT ( 'NONE', #23452 ) ;
#2454=LINE ( 'NONE', #32490, #18082 ) ;
#2456=ORIENTED_EDGE ( 'NONE', *, *, #11933, .T. ) ;
#2464=DIRECTION ( 'NONE',  ( 0.2756373558170082672, -0.9612616959383162296, 0.000000000000000000 ) ) ;
#2471=CARTESIAN_POINT ( 'NONE',  ( -41.93344242462055149, 13.82826554927147988, 59.53596428539564300 ) ) ;
#2477=CYLINDRICAL_SURFACE ( 'NONE', #20687, 0.1000000000000008243 ) ;
#2478=ORIENTED_EDGE ( 'NONE', *, *, #16762, .T. ) ;
#2479=VERTEX_POINT ( 'NONE', #18513 ) ;
#2485=VERTEX_POINT ( 'NONE', #18673 ) ;
#2487=CIRCLE ( 'NONE', #911, 1.300000000000002487 ) ;
#2488=DIRECTION ( 'NONE',  ( 0.8746197071393926326, -0.4848096202463430537, -8.676864087101709653E-18 ) ) ;
#2492=CARTESIAN_POINT ( 'NONE',  ( -42.60588768478345401, 14.57151196022700113, 37.04930799450052348 ) ) ;
#2493=CYLINDRICAL_SURFACE ( 'NONE', #10685, 0.1000000000000018235 ) ;
#2499=VERTEX_POINT ( 'NONE', #11306 ) ;
#2502=DIRECTION ( 'NONE',  ( 0.3428121700606596156, 0.6184495258776487869, 0.7071067811865566766 ) ) ;
#2503=CARTESIAN_POINT ( 'NONE',  ( -43.90780810587784089, -0.03953120679776574165, 32.14930799450051779 ) ) ;
#2517=AXIS2_PLACEMENT_3D ( 'NONE', #16868, #29187, #24258 ) ;
#2529=AXIS2_PLACEMENT_3D ( 'NONE', #19130, #19467, #9299 ) ;
#2544=ORIENTED_EDGE ( 'NONE', *, *, #17977, .F. ) ;
#2552=ORIENTED_EDGE ( 'NONE', *, *, #25358, .T. ) ;
#2555=VECTOR ( 'NONE', #21564, 1000.000000000000114 ) ;
#2558=CIRCLE ( 'NONE', #16691, 1.899999999999999023 ) ;
#2562=ADVANCED_FACE ( 'NONE', ( #24090 ), #6868, .F. ) ;
#2572=EDGE_LOOP ( 'NONE', ( #24176, #17970, #898, #18395 ) ) ;
#2574=DIRECTION ( 'NONE',  ( -0.8746197071393926326, 0.4848096202463430537, 8.676864087101709653E-18 ) ) ;
#2575=VECTOR ( 'NONE', #21813, 1000.000000000000227 ) ;
#2576=EDGE_LOOP ( 'NONE', ( #56, #9669, #26047, #25845 ) ) ;
#2577=CARTESIAN_POINT ( 'NONE',  ( -41.01929587258828747, 9.401204285752058354, 35.44930799450052206 ) ) ;
#2582=CARTESIAN_POINT ( 'NONE',  ( -40.90015969217747482, 8.955334253785162346, 57.95249952744806166 ) ) ;
#2584=DIRECTION ( 'NONE',  ( -0.8746197071393925215, 0.4848096202463429982, 1.121857559391816958E-19 ) ) ;
#2585=CARTESIAN_POINT ( 'NONE',  ( -40.64500813507293486, 6.819128862114092193, 39.51928662074344345 ) ) ;
#2586=EDGE_CURVE ( 'NONE', #655, #6754, #17979, .T. ) ;
#2587=ORIENTED_EDGE ( 'NONE', *, *, #29280, .T. ) ;
#2590=ORIENTED_EDGE ( 'NONE', *, *, #22060, .T. ) ;
#2597=DIRECTION ( 'NONE',  ( -0.4848096202463430537, -0.8746197071393926326, -9.920727850371701658E-18 ) ) ;
#2599=EDGE_CURVE ( 'NONE', #17105, #11324, #6696, .T. ) ;
#2606=AXIS2_PLACEMENT_3D ( 'NONE', #26812, #21379, #26644 ) ;
#2620=CARTESIAN_POINT ( 'NONE',  ( -39.50554051497144314, 7.696103224718195968, 62.04930799450052348 ) ) ;
#2624=SHAPE_DEFINITION_REPRESENTATION ( #25040, #28161 ) ;
#2627=CARTESIAN_POINT ( 'NONE',  ( -42.70758099689500398, -0.7619956604996156457, 32.09930799450052064 ) ) ;
#2640=CARTESIAN_POINT ( 'NONE',  ( -36.18493864628602807, 8.798967949527998655, 53.84930799450051353 ) ) ;
#2641=EDGE_CURVE ( 'NONE', #13496, #21395, #7024, .T. ) ;
#2642=CIRCLE ( 'NONE', #23062, 1.000000000000002220 ) ;
#2643=CIRCLE ( 'NONE', #17, 1.300000000000002487 ) ;
#2645=VERTEX_POINT ( 'NONE', #32144 ) ;
#2648=CARTESIAN_POINT ( 'NONE',  ( -41.74033427429298371, 15.41509661078533355, 38.54930799450052348 ) ) ;
#2659=CYLINDRICAL_SURFACE ( 'NONE', #29429, 0.1000000000000028644 ) ;
#2661=AXIS2_PLACEMENT_3D ( 'NONE', #11338, #26104, #23330 ) ;
#2663=EDGE_CURVE ( 'NONE', #1880, #18016, #6540, .T. ) ;
#2664=DIRECTION ( 'NONE',  ( -0.7141240004913222972, 0.3958453973320028019, -0.5773502691896303940 ) ) ;
#2668=DIRECTION ( 'NONE',  ( 0.000000000000000000, 0.000000000000000000, -1.000000000000000000 ) ) ;
#2669=CIRCLE ( 'NONE', #23099, 0.1000000000000018235 ) ;
#2678=ORIENTED_EDGE ( 'NONE', *, *, #2248, .F. ) ;
#2679=CARTESIAN_POINT ( 'NONE',  ( -40.65762574042817334, 9.591092754368338191, 35.59072935073783128 ) ) ;
#2682=FACE_OUTER_BOUND ( 'NONE', #28319, .T. ) ;
#2687=CIRCLE ( 'NONE', #21013, 0.9999999999999978906 ) ;
#2692=LINE ( 'NONE', #10251, #6619 ) ;
#2693=CARTESIAN_POINT ( 'NONE',  ( -42.50976151518962354, 14.59907569580870224, 38.19144330556764544 ) ) ;
#2694=AXIS2_PLACEMENT_3D ( 'NONE', #20538, #32372, #7590 ) ;
#2695=ORIENTED_EDGE ( 'NONE', *, *, #16677, .F. ) ;
#2696=CARTESIAN_POINT ( 'NONE',  ( -40.80566404189690388, 8.441333990788717045, 34.56793150177820451 ) ) ;
#2697=VERTEX_POINT ( 'NONE', #2585 ) ;
#2700=CARTESIAN_POINT ( 'NONE',  ( -39.52978099598376360, 7.652372239361226569, 32.09930799450052064 ) ) ;
#2701=CARTESIAN_POINT ( 'NONE',  ( -39.67555847965937943, 2.645252416024337361, 47.04930799450051637 ) ) ;
#2704=DIRECTION ( 'NONE',  ( 0.2072038891212098777, -0.4540212254542328463, -0.8665629089512670857 ) ) ;
#2719=EDGE_CURVE ( 'NONE', #26808, #16648, #7355, .T. ) ;
#2720=ORIENTED_EDGE ( 'NONE', *, *, #10034, .F. ) ;
#2722=CARTESIAN_POINT ( 'NONE',  ( -40.46271621608484281, 3.081581074246044327, 32.14930799450051779 ) ) ;
#2723=ORIENTED_EDGE ( 'NONE', *, *, #27198, .F. ) ;
#2725=CIRCLE ( 'NONE', #15306, 0.1000000000000014905 ) ;
#2729=DIRECTION ( 'NONE',  ( -0.4848096202463430537, -0.8746197071393926326, -9.920727850371701658E-18 ) ) ;
#2731=ORIENTED_EDGE ( 'NONE', *, *, #27073, .F. ) ;
#2732=VERTEX_POINT ( 'NONE', #19810 ) ;
#2740=ORIENTED_EDGE ( 'NONE', *, *, #4168, .F. ) ;
#2746=DIRECTION ( 'NONE',  ( -0.2743622330404226206, 0.9568148143496237878, 0.09607692814702083195 ) ) ;
#2748=CARTESIAN_POINT ( 'NONE',  ( -40.52669582637187773, 7.652910973922034010, 53.94439779120588696 ) ) ;
#2753=CARTESIAN_POINT ( 'NONE',  ( -40.13606231985500017, 7.635531802539801127, 60.29072935073781991 ) ) ;
#2754=VERTEX_POINT ( 'NONE', #2753 ) ;
#2758=CARTESIAN_POINT ( 'NONE',  ( -40.80097511801616150, 8.246641009394465982, 59.64930799450051779 ) ) ;
#2762=ORIENTED_EDGE ( 'NONE', *, *, #1929, .F. ) ;
#2770=EDGE_CURVE ( 'NONE', #7874, #11316, #29009, .T. ) ;
#2771=ORIENTED_EDGE ( 'NONE', *, *, #6793, .F. ) ;
#2777=ADVANCED_FACE ( 'NONE', ( #12782 ), #28025, .T. ) ;
#2781=ORIENTED_EDGE ( 'NONE', *, *, #809, .F. ) ;
#2788=ORIENTED_EDGE ( 'NONE', *, *, #19743, .T. ) ;
#2789=VERTEX_POINT ( 'NONE', #27696 ) ;
#2795=EDGE_LOOP ( 'NONE', ( #424, #16242, #2877, #20423 ) ) ;
#2796=FACE_OUTER_BOUND ( 'NONE', #7289, .T. ) ;
#2798=DIRECTION ( 'NONE',  ( 0.9612616959383193382, 0.2756373558169973870, 8.795445018804928853E-19 ) ) ;
#2804=FACE_OUTER_BOUND ( 'NONE', #22909, .T. ) ;
#2805=CARTESIAN_POINT ( 'NONE',  ( -42.47434154250543514, 4.196643200812633978, 35.14930799450051779 ) ) ;
#2807=ORIENTED_EDGE ( 'NONE', *, *, #22162, .F. ) ;
#2808=DIRECTION ( 'NONE',  ( -0.2756373558169956106, 0.9612616959383197823, 0.000000000000000000 ) ) ;
#2809=FACE_OUTER_BOUND ( 'NONE', #30576, .T. ) ;
#2810=CARTESIAN_POINT ( 'NONE',  ( -41.96544240928614755, 13.75880317176705603, 54.54930799450051637 ) ) ;
#2819=VECTOR ( 'NONE', #3476, 1000.000000000000000 ) ;
#2820=DIRECTION ( 'NONE',  ( -2.779292025043186357E-18, 1.288349127009862211E-17, -1.000000000000000000 ) ) ;
#2828=CARTESIAN_POINT ( 'NONE',  ( -39.67555847965937943, 2.645252416024337361, 47.04930799450051637 ) ) ;
#2831=VERTEX_POINT ( 'NONE', #22605 ) ;
#2832=CARTESIAN_POINT ( 'NONE',  ( -42.38263560350583248, 14.61917486843862868, 53.54930799450051637 ) ) ;
#2835=DIRECTION ( 'NONE',  ( -2.779292025043186357E-18, 1.288349127009862211E-17, -1.000000000000000000 ) ) ;
#2842=ADVANCED_FACE ( 'NONE', ( #8323 ), #11567, .T. ) ;
#2844=DIRECTION ( 'NONE',  ( 2.779292025043186357E-18, -1.288349127009862057E-17, 1.000000000000000000 ) ) ;
#2845=DIRECTION ( 'NONE',  ( -0.2756373558169932236, 0.9612616959383205595, -1.479773560108267395E-16 ) ) ;
#2847=EDGE_LOOP ( 'NONE', ( #18759, #30686 ) ) ;
#2848=CARTESIAN_POINT ( 'NONE',  ( -40.85259535153578270, 8.476421318711492958, 34.61707255558062002 ) ) ;
#2850=EDGE_CURVE ( 'NONE', #1764, #2499, #23259, .T. ) ;
#2852=DIRECTION ( 'NONE',  ( 0.000000000000000000, 0.000000000000000000, -1.000000000000000000 ) ) ;
#2858=VERTEX_POINT ( 'NONE', #5699 ) ;
#2862=AXIS2_PLACEMENT_3D ( 'NONE', #4608, #7241, #12334 ) ;
#2864=CARTESIAN_POINT ( 'NONE',  ( -40.47970302497625994, 7.463434137431151250, 53.54930799450051637 ) ) ;
#2865=VECTOR ( 'NONE', #14637, 1000.000000000000114 ) ;
#2866=DIRECTION ( 'NONE',  ( -0.8746197071393926326, 0.4848096202463430537, 8.676864087101709653E-18 ) ) ;
#2869=FACE_OUTER_BOUND ( 'NONE', #1078, .T. ) ;
#2877=ORIENTED_EDGE ( 'NONE', *, *, #19461, .F. ) ;
#2885=AXIS2_PLACEMENT_3D ( 'NONE', #29205, #24766, #14765 ) ;
#2889=VERTEX_POINT ( 'NONE', #23261 ) ;
#2891=ADVANCED_FACE ( 'NONE', ( #773 ), #3548, .T. ) ;
#2896=EDGE_LOOP ( 'NONE', ( #10191, #14250, #4824, #25229 ) ) ;
#2900=CARTESIAN_POINT ( 'NONE',  ( -41.13156850465621517, 9.429949956619452678, 35.64930799450052490 ) ) ;
#2901=EDGE_LOOP ( 'NONE', ( #29208, #11999, #12158, #28052 ) ) ;
#2904=DIRECTION ( 'NONE',  ( -2.779292025043186357E-18, 1.288349127009862211E-17, -1.000000000000000000 ) ) ;
#2906=AXIS2_PLACEMENT_3D ( 'NONE', #9143, #13758, #18812 ) ;
#2907=CARTESIAN_POINT ( 'NONE',  ( -40.06561427811386267, 7.496110634155836117, 54.64930799450051779 ) ) ;
#2914=DIRECTION ( 'NONE',  ( -0.2756373558170082672, 0.9612616959383162296, 0.000000000000000000 ) ) ;
#2916=ORIENTED_EDGE ( 'NONE', *, *, #5389, .T. ) ;
#2921=CARTESIAN_POINT ( 'NONE',  ( -38.41701585771487260, 6.978388747684010518, 62.04930799450052348 ) ) ;
#2922=AXIS2_PLACEMENT_3D ( 'NONE', #22353, #24663, #2180 ) ;
#2944=DIRECTION ( 'NONE',  ( 0.1949050434465264547, -0.6797146636928678154, 0.7071067811865470176 ) ) ;
#2947=EDGE_LOOP ( 'NONE', ( #22043, #26815, #24946, #6905 ) ) ;
#2948=CARTESIAN_POINT ( 'NONE',  ( -40.20068974435373121, 7.604379238274955100, 53.94930799450051495 ) ) ;
#2951=ORIENTED_EDGE ( 'NONE', *, *, #24151, .F. ) ;
#2955=ORIENTED_EDGE ( 'NONE', *, *, #21589, .F. ) ;
#2957=CARTESIAN_POINT ( 'NONE',  ( -42.38687957179150345, 4.148162238788003719, 57.04930799450051637 ) ) ;
#2963=DIRECTION ( 'NONE',  ( -0.9612616959383205595, -0.2756373558169931681, 1.660411357259282445E-16 ) ) ;
#2965=VECTOR ( 'NONE', #31329, 1000.000000000000000 ) ;
#2967=CARTESIAN_POINT ( 'NONE',  ( -40.70484894842233103, 8.274204744976163539, 54.44930799450051495 ) ) ;
#2968=DIRECTION ( 'NONE',  ( 0.000000000000000000, 1.517883041479704827E-15, -1.000000000000000000 ) ) ;
#2969=CARTESIAN_POINT ( 'NONE',  ( -40.57832943677391313, 7.446916543903029151, 60.23803160207061325 ) ) ;
#2971=CARTESIAN_POINT ( 'NONE',  ( -39.59300248568538194, 7.744584186742829779, 32.04930799450052348 ) ) ;
#2973=CARTESIAN_POINT ( 'NONE',  ( -42.37913764077812573, 15.23192269303853053, 38.44930799450052206 ) ) ;
#2975=ORIENTED_EDGE ( 'NONE', *, *, #14761, .F. ) ;
#2976=LINE ( 'NONE', #11187, #1899 ) ;
#2981=CARTESIAN_POINT ( 'NONE',  ( -41.23380787120766655, 11.23768311167744294, 35.90717268343339441 ) ) ;
#2983=CARTESIAN_POINT ( 'NONE',  ( -40.00476266209339116, 7.314288625133150035, 38.76830122587732319 ) ) ;
#2990=EDGE_CURVE ( 'NONE', #4508, #8640, #27007, .T. ) ;
#3002=ADVANCED_FACE ( 'NONE', ( #32105 ), #6663, .T. ) ;
#3004=DIRECTION ( 'NONE',  ( -0.8746197071393926326, 0.4848096202463430537, 8.676864087101709653E-18 ) ) ;
#3031=EDGE_CURVE ( 'NONE', #16525, #8364, #3873, .T. ) ;
#3033=EDGE_CURVE ( 'NONE', #23532, #9452, #20647, .T. ) ;
#3034=VECTOR ( 'NONE', #6705, 1000.000000000000114 ) ;
#3039=DIRECTION ( 'NONE',  ( 0.4848096202463430537, 0.8746197071393926326, 9.920727850371700117E-18 ) ) ;
#3050=VERTEX_POINT ( 'NONE', #8962 ) ;
#3054=CARTESIAN_POINT ( 'NONE',  ( -40.18454328187963398, 7.548069831825862330, 53.64930799450051779 ) ) ;
#3056=CARTESIAN_POINT ( 'NONE',  ( -44.16550389150962985, 1.558238629217584492, 34.54930799450052348 ) ) ;
#3057=DIRECTION ( 'NONE',  ( 0.000000000000000000, 0.000000000000000000, -1.000000000000000000 ) ) ;
#3062=CARTESIAN_POINT ( 'NONE',  ( -40.90015969217747482, 8.955334253785164123, 57.04930799450051637 ) ) ;
#3071=CIRCLE ( 'NONE', #6753, 1.300000000000002487 ) ;
#3072=ORIENTED_EDGE ( 'NONE', *, *, #16965, .F. ) ;
#3073=EDGE_CURVE ( 'NONE', #9700, #17034, #4934, .T. ) ;
#3079=AXIS2_PLACEMENT_3D ( 'NONE', #16869, #3916, #19495 ) ;
#3081=CYLINDRICAL_SURFACE ( 'NONE', #23837, 1.500000000000001332 ) ;
#3082=FACE_OUTER_BOUND ( 'NONE', #52, .T. ) ;
#3093=DIRECTION ( 'NONE',  ( 0.2756373558170013283, -0.9612616959383183390, 0.000000000000000000 ) ) ;
#3095=ORIENTED_EDGE ( 'NONE', *, *, #26603, .T. ) ;
#3098=CARTESIAN_POINT ( 'NONE',  ( -37.42114908093812176, 11.86897798031838391, 60.54930799450051637 ) ) ;
#3103=AXIS2_PLACEMENT_3D ( 'NONE', #14838, #26969, #4490 ) ;
#3104=EDGE_CURVE ( 'NONE', #7358, #18405, #20104, .T. ) ;
#3106=VERTEX_POINT ( 'NONE', #5347 ) ;
#3116=VECTOR ( 'NONE', #20424, 1000.000000000000114 ) ;
#3121=CARTESIAN_POINT ( 'NONE',  ( -40.73091736380679606, 9.483895492497158131, 39.44930799450052206 ) ) ;
#3127=DIRECTION ( 'NONE',  ( 1.431146867680865853E-17, 2.558717127065790464E-17, 1.000000000000000000 ) ) ;
#3130=PLANE ( 'NONE',  #9431 ) ;
#3132=ORIENTED_EDGE ( 'NONE', *, *, #13461, .T. ) ;
#3133=EDGE_LOOP ( 'NONE', ( #16009, #187, #22875, #25955 ) ) ;
#3141=CARTESIAN_POINT ( 'NONE',  ( -40.02667234278160890, 7.000595883235202876, 39.42620813939996793 ) ) ;
#3151=ADVANCED_FACE ( 'NONE', ( #27335 ), #21146, .T. ) ;
#3153=ORIENTED_EDGE ( 'NONE', *, *, #29232, .T. ) ;
#3156=AXIS2_PLACEMENT_3D ( 'NONE', #31133, #8483, #18478 ) ;
#3157=AXIS2_PLACEMENT_3D ( 'NONE', #31995, #2729, #25374 ) ;
#3159=AXIS2_PLACEMENT_3D ( 'NONE', #32179, #14457, #32009 ) ;
#3163=DIRECTION ( 'NONE',  ( -0.7141240004913222972, 0.3958453973320028019, 0.5773502691896303940 ) ) ;
#3165=ADVANCED_FACE ( 'NONE', ( #2869 ), #29802, .F. ) ;
#3171=ORIENTED_EDGE ( 'NONE', *, *, #28400, .T. ) ;
#3173=CARTESIAN_POINT ( 'NONE',  ( -37.58300281841709989, 16.01180101885526597, 38.09144330556765112 ) ) ;
#3179=ORIENTED_EDGE ( 'NONE', *, *, #18966, .T. ) ;
#3180=DIRECTION ( 'NONE',  ( -0.9612616959383205595, -0.2756373558169932236, 1.660411357259282445E-16 ) ) ;
#3182=FACE_OUTER_BOUND ( 'NONE', #27297, .T. ) ;
#3183=EDGE_LOOP ( 'NONE', ( #25096, #32071, #16042, #7853 ) ) ;
#3193=ORIENTED_EDGE ( 'NONE', *, *, #14864, .T. ) ;
#3204=EDGE_CURVE ( 'NONE', #14460, #10889, #6476, .T. ) ;
#3208=AXIS2_PLACEMENT_3D ( 'NONE', #29141, #31767, #3868 ) ;
#3234=VERTEX_POINT ( 'NONE', #20907 ) ;
#3236=CARTESIAN_POINT ( 'NONE',  ( -40.20380355051744914, 8.008426694338135476, 40.07149053519532345 ) ) ;
#3237=ORIENTED_EDGE ( 'NONE', *, *, #20116, .T. ) ;
#3241=CIRCLE ( 'NONE', #15827, 2.000000000000001776 ) ;
#3246=ADVANCED_FACE ( 'NONE', ( #3182 ), #13226, .F. ) ;
#3247=CARTESIAN_POINT ( 'NONE',  ( -40.59758774925371938, 7.567737757495683226, 39.54930799450052348 ) ) ;
#3250=VERTEX_POINT ( 'NONE', #1201 ) ;
#3251=AXIS2_PLACEMENT_3D ( 'NONE', #32371, #36, #14975 ) ;
#3256=EDGE_LOOP ( 'NONE', ( #10233, #3596, #9853, #1908 ) ) ;
#3257=ORIENTED_EDGE ( 'NONE', *, *, #933, .F. ) ;
#3264=CARTESIAN_POINT ( 'NONE',  ( -40.15599670534037102, 7.478908884098773413, 38.70582007960419446 ) ) ;
#3269=ORIENTED_EDGE ( 'NONE', *, *, #2230, .T. ) ;
#3280=AXIS2_PLACEMENT_3D ( 'NONE', #27857, #20132, #12438 ) ;
#3282=VECTOR ( 'NONE', #14060, 1000.000000000000114 ) ;
#3284=DIRECTION ( 'NONE',  ( -0.8746197071393858602, 0.4848096202463547666, 0.000000000000000000 ) ) ;
#3287=VERTEX_POINT ( 'NONE', #5828 ) ;
#3298=EDGE_CURVE ( 'NONE', #26367, #19002, #23535, .T. ) ;
#3302=AXIS2_PLACEMENT_3D ( 'NONE', #32289, #11932, #29504 ) ;
#3305=ORIENTED_EDGE ( 'NONE', *, *, #32444, .T. ) ;
#3307=FACE_OUTER_BOUND ( 'NONE', #6013, .T. ) ;
#3314=CARTESIAN_POINT ( 'NONE',  ( -40.75848109938849717, 9.580021662090986823, 35.54930799450052348 ) ) ;
#3322=EDGE_CURVE ( 'NONE', #21428, #30206, #196, .T. ) ;
#3324=EDGE_LOOP ( 'NONE', ( #390, #19888, #25132, #6051 ) ) ;
#3326=CIRCLE ( 'NONE', #11684, 0.1000000000000006301 ) ;
#3331=CARTESIAN_POINT ( 'NONE',  ( -40.76967387488526384, 8.530668925462080665, 39.44930799450052206 ) ) ;
#3332=ORIENTED_EDGE ( 'NONE', *, *, #6264, .T. ) ;
#3334=CARTESIAN_POINT ( 'NONE',  ( -40.59783212598352264, 7.538197204814764518, 53.99316187147203294 ) ) ;
#3337=EDGE_CURVE ( 'NONE', #25278, #286, #24298, .T. ) ;
#3346=CARTESIAN_POINT ( 'NONE',  ( -40.11669538345027064, 6.804256812083823824, 34.64773285490134214 ) ) ;
#3348=ORIENTED_EDGE ( 'NONE', *, *, #30107, .F. ) ;
#3351=DIRECTION ( 'NONE',  ( 0.9612616959383205595, 0.2756373558169932236, -1.660411357259282445E-16 ) ) ;
#3353=DIRECTION ( 'NONE',  ( 0.4848096202463430537, 0.8746197071393926326, 9.920727850371700117E-18 ) ) ;
#3355=CARTESIAN_POINT ( 'NONE',  ( -43.64073206722599707, 1.267352857069780736, 39.54930799450052348 ) ) ;
#3359=ORIENTED_EDGE ( 'NONE', *, *, #32430, .T. ) ;
#3362=EDGE_CURVE ( 'NONE', #777, #16797, #18442, .T. ) ;
#3363=AXIS2_PLACEMENT_3D ( 'NONE', #26945, #4463, #9061 ) ;
#3364=CARTESIAN_POINT ( 'NONE',  ( -36.76418579970419387, 10.14130568307076352, 56.14611646155296398 ) ) ;
#3368=AXIS2_PLACEMENT_3D ( 'NONE', #21853, #6447, #16448 ) ;
#3371=CIRCLE ( 'NONE', #19084, 0.09999999999999795164 ) ;
#3375=ADVANCED_FACE ( 'NONE', ( #23378 ), #25677, .T. ) ;
#3377=CARTESIAN_POINT ( 'NONE',  ( -40.45528000798979917, 8.522633796558835684, 34.54930799450052348 ) ) ;
#3384=CARTESIAN_POINT ( 'NONE',  ( -43.95628906790246759, -0.1269931775117038586, 32.04930799450052348 ) ) ;
#3387=VERTEX_POINT ( 'NONE', #11229 ) ;
#3392=VERTEX_POINT ( 'NONE', #5503 ) ;
#3397=VECTOR ( 'NONE', #7915, 1000.000000000000000 ) ;
#3398=AXIS2_PLACEMENT_3D ( 'NONE', #26704, #11778, #9309 ) ;
#3401=AXIS2_PLACEMENT_3D ( 'NONE', #3445, #13629, #5759 ) ;
#3402=ORIENTED_EDGE ( 'NONE', *, *, #8220, .T. ) ;
#3404=EDGE_CURVE ( 'NONE', #6754, #6409, #29438, .T. ) ;
#3411=( BOUNDED_CURVE ( )  B_SPLINE_CURVE ( 3, ( #31654, #4238, #26715, #9317 ),
 .UNSPECIFIED., .F., .F. ) 
 B_SPLINE_CURVE_WITH_KNOTS ( ( 4, 4 ),
 ( 1.570796326794888342, 1.630650672327995210 ),
 .UNSPECIFIED. ) 
 CURVE ( )  GEOMETRIC_REPRESENTATION_ITEM ( )  RATIONAL_B_SPLINE_CURVE ( ( 1.000000000000000000, 0.9997014770583808607, 0.9997014770583808607, 1.000000000000000000 ) ) 
 REPRESENTATION_ITEM ( '' )  );
#3412=DIRECTION ( 'NONE',  ( 0.9612616959383205595, 0.2756373558169932236, -1.660411357259282445E-16 ) ) ;
#3417=ORIENTED_EDGE ( 'NONE', *, *, #24032, .T. ) ;
#3418=ORIENTED_EDGE ( 'NONE', *, *, #4412, .T. ) ;
#3419=FACE_OUTER_BOUND ( 'NONE', #19613, .T. ) ;
#3422=CARTESIAN_POINT ( 'NONE',  ( -43.37834615508418068, 1.121909970995877082, 39.44930799450052916 ) ) ;
#3434=ORIENTED_EDGE ( 'NONE', *, *, #5360, .T. ) ;
#3435=FACE_OUTER_BOUND ( 'NONE', #7203, .T. ) ;
#3436=CARTESIAN_POINT ( 'NONE',  ( -40.50726676055793973, 7.559560307024990600, 53.80788663826320573 ) ) ;
#3439=VERTEX_POINT ( 'NONE', #31738 ) ;
#3440=AXIS2_PLACEMENT_3D ( 'NONE', #29927, #10380, #12364 ) ;
#3442=EDGE_CURVE ( 'NONE', #3984, #15332, #16746, .T. ) ;
#3445=CARTESIAN_POINT ( 'NONE',  ( -40.41018466243807694, 8.365367637131765122, 40.47149053519531492 ) ) ;
#3448=CIRCLE ( 'NONE', #12899, 0.1000000000000004774 ) ;
#3456=CARTESIAN_POINT ( 'NONE',  ( -43.29088418437023478, 1.073429008971242382, 34.64930799450052490 ) ) ;
#3459=DIRECTION ( 'NONE',  ( 0.2756373558169932236, -0.9612616959383204485, 1.479773560108267395E-16 ) ) ;
#3461=FILL_AREA_STYLE_COLOUR ( '', #24962 ) ;
#3462=EDGE_LOOP ( 'NONE', ( #11825, #22006, #19417, #25704 ) ) ;
#3470=CARTESIAN_POINT ( 'NONE',  ( -42.12525683681430877, 14.70933063813549424, 35.90717268343339441 ) ) ;
#3473=LINE ( 'NONE', #13344, #15733 ) ;
#3475=AXIS2_PLACEMENT_3D ( 'NONE', #22053, #1542, #21886 ) ;
#3476=DIRECTION ( 'NONE',  ( -0.6184495258776654403, 0.3428121700606547861, -0.7071067811865443531 ) ) ;
#3477=EDGE_CURVE ( 'NONE', #18541, #2754, #20404, .T. ) ;
#3485=CARTESIAN_POINT ( 'NONE',  ( -41.94956971822180947, 3.905757428664828890, 47.04930799450051637 ) ) ;
#3490=CARTESIAN_POINT ( 'NONE',  ( -42.28301147118429526, 15.25948642862022986, 38.44930799450052206 ) ) ;
#3498=CARTESIAN_POINT ( 'NONE',  ( -40.38492706200820948, 8.640065911210484728, 34.64831079233957212 ) ) ;
#3499=FACE_OUTER_BOUND ( 'NONE', #11549, .T. ) ;
#3505=ORIENTED_EDGE ( 'NONE', *, *, #24683, .T. ) ;
#3506=DIRECTION ( 'NONE',  ( 0.8746197071393926326, -0.4848096202463430537, -8.676864087101709653E-18 ) ) ;
#3507=DIRECTION ( 'NONE',  ( 0.9612616959383205595, 0.2756373558169932236, -1.660411357259282445E-16 ) ) ;
#3509=LINE ( 'NONE', #23539, #16210 ) ;
#3512=CARTESIAN_POINT ( 'NONE',  ( -40.58856461370174173, 7.499380836222960589, 60.14930799450051779 ) ) ;
#3514=B_SPLINE_CURVE_WITH_KNOTS ( 'NONE', 3,
 ( #400, #8604, #28151, #10600, #30616, #31095, #8128, #10759 ),
 .UNSPECIFIED., .F., .F.,
 ( 4, 2, 2, 4 ),
 ( 0.000000000000000000, 0.0002680696438040274616, 0.0005361392876080549232, 0.001072278575216109846 ),
 .UNSPECIFIED. ) ;
#3519=EDGE_CURVE ( 'NONE', #13529, #23253, #4154, .T. ) ;
#3521=VECTOR ( 'NONE', #18862, 1000.000000000000114 ) ;
#3525=CARTESIAN_POINT ( 'NONE',  ( -40.70335362822509495, 9.387769322903324110, 34.54930799450052348 ) ) ;
#3526=VECTOR ( 'NONE', #1326, 1000.000000000000114 ) ;
#3528=CARTESIAN_POINT ( 'NONE',  ( -43.29088418437023478, 1.073429008971243492, 39.54930799450052348 ) ) ;
#3538=CARTESIAN_POINT ( 'NONE',  ( -43.38408989745150990, 1.111547985471239786, 60.44930799450051495 ) ) ;
#3541=CARTESIAN_POINT ( 'NONE',  ( -42.38687957179149635, 4.148162238787999279, 38.94930799450052206 ) ) ;
#3542=DIRECTION ( 'NONE',  ( 0.9612616959383164517, 0.2756373558170082116, -1.660411357259305371E-16 ) ) ;
#3548=CYLINDRICAL_SURFACE ( 'NONE', #13332, 0.1000000000000018235 ) ;
#3549=VERTEX_POINT ( 'NONE', #22696 ) ;
#3558=CIRCLE ( 'NONE', #21366, 0.09999999999999939493 ) ;
#3560=AXIS2_PLACEMENT_3D ( 'NONE', #9657, #24583, #9496 ) ;
#3562=CIRCLE ( 'NONE', #29798, 0.1000000000000027811 ) ;
#3574=DIRECTION ( 'NONE',  ( 0.4848096202463427762, 0.8746197071393925215, -2.220446049250312588E-16 ) ) ;
#3575=ORIENTED_EDGE ( 'NONE', *, *, #17900, .F. ) ;
#3576=EDGE_CURVE ( 'NONE', #286, #16387, #9579, .T. ) ;
#3578=CARTESIAN_POINT ( 'NONE',  ( -40.56500720768295309, 7.149487417332511363, 38.92324275860853078 ) ) ;
#3579=CARTESIAN_POINT ( 'NONE',  ( -40.68422973805265030, 6.807290781432339344, 39.32248954417796227 ) ) ;
#3584=FACE_OUTER_BOUND ( 'NONE', #23361, .T. ) ;
#3590=LINE ( 'NONE', #6218, #24504 ) ;
#3596=ORIENTED_EDGE ( 'NONE', *, *, #25354, .T. ) ;
#3600=EDGE_CURVE ( 'NONE', #28668, #15332, #31965, .T. ) ;
#3601=AXIS2_PLACEMENT_3D ( 'NONE', #32164, #24117, #9676 ) ;
#3606=CYLINDRICAL_SURFACE ( 'NONE', #7617, 0.1000000000000006301 ) ;
#3610=ORIENTED_EDGE ( 'NONE', *, *, #1336, .F. ) ;
#3614=EDGE_CURVE ( 'NONE', #7068, #14556, #5138, .T. ) ;
#3619=CARTESIAN_POINT ( 'NONE',  ( -39.58809650894544774, 2.596771453999702661, 48.94930799450051495 ) ) ;
#3621=DIRECTION ( 'NONE',  ( 0.000000000000000000, 0.000000000000000000, -1.000000000000000000 ) ) ;
#3622=SPHERICAL_SURFACE ( 'NONE', #17842, 0.1000000000000000056 ) ;
#3625=APPLICATION_CONTEXT ( 'automotive_design' ) ;
#3630=AXIS2_PLACEMENT_3D ( 'NONE', #19080, #3507, #13857 ) ;
#3631=EDGE_CURVE ( 'NONE', #13895, #27622, #17605, .T. ) ;
#3637=CARTESIAN_POINT ( 'NONE',  ( -40.61463551858322063, 9.441168033762318501, 34.67959690138647488 ) ) ;
#3644=SPHERICAL_SURFACE ( 'NONE', #7897, 0.1000000000000000056 ) ;
#3652=TOROIDAL_SURFACE ( 'NONE', #15709, 1.299999999999999822, 0.1000000000000000056 ) ;
#3661=VERTEX_POINT ( 'NONE', #22361 ) ;
#3667=CARTESIAN_POINT ( 'NONE',  ( -40.28779227465695101, 2.984619150196775372, 35.04930799450051637 ) ) ;
#3668=DIRECTION ( 'NONE',  ( 0.8746197071393926326, -0.4848096202463430537, -8.676864087101709653E-18 ) ) ;
#3670=CYLINDRICAL_SURFACE ( 'NONE', #10858, 0.1000000000000028644 ) ;
#3672=CARTESIAN_POINT ( 'NONE',  ( -41.74593813222361405, 15.43463958587387808, 35.54930799450051637 ) ) ;
#3674=DIRECTION ( 'NONE',  ( 0.2756373558170093774, -0.9612616959383158965, 3.469446951953606616E-14 ) ) ;
#3676=LINE ( 'NONE', #3355, #31966 ) ;
#3678=ORIENTED_EDGE ( 'NONE', *, *, #30035, .T. ) ;
#3679=VERTEX_POINT ( 'NONE', #23179 ) ;
#3682=VERTEX_POINT ( 'NONE', #23340 ) ;
#3685=AXIS2_PLACEMENT_3D ( 'NONE', #26675, #26190, #1237 ) ;
#3693=LINE ( 'NONE', #3528, #6700 ) ;
#3700=CARTESIAN_POINT ( 'NONE',  ( -39.81647664150466426, 8.705807714305638711, 34.54930799450052348 ) ) ;
#3701=CARTESIAN_POINT ( 'NONE',  ( -40.13606231985500017, 7.635531802539802015, 60.54930799450051637 ) ) ;
#3702=ORIENTED_EDGE ( 'NONE', *, *, #29908, .T. ) ;
#3704=ADVANCED_FACE ( 'NONE', ( #15619 ), #3652, .T. ) ;
#3713=ORIENTED_EDGE ( 'NONE', *, *, #8139, .F. ) ;
#3722=DIRECTION ( 'NONE',  ( 2.779292025043186357E-18, -1.288349127009862211E-17, 1.000000000000000000 ) ) ;
#3728=ORIENTED_EDGE ( 'NONE', *, *, #31274, .F. ) ;
#3730=FACE_OUTER_BOUND ( 'NONE', #28754, .T. ) ;
#3739=DIRECTION ( 'NONE',  ( 0.4848096202463430537, 0.8746197071393926326, -1.125439520643636483E-16 ) ) ;
#3741=ORIENTED_EDGE ( 'NONE', *, *, #18376, .T. ) ;
#3742=CARTESIAN_POINT ( 'NONE',  ( -41.01929587258828036, 9.401204285752060130, 34.64930799450051779 ) ) ;
#3743=CARTESIAN_POINT ( 'NONE',  ( -40.57119026524328831, 6.941393190194602880, 39.15667507985590845 ) ) ;
#3744=LINE ( 'NONE', #23763, #27015 ) ;
#3747=ADVANCED_FACE ( 'NONE', ( #365 ), #12829, .T. ) ;
#3750=ADVANCED_FACE ( 'NONE', ( #11839 ), #8723, .T. ) ;
#3754=DIRECTION ( 'NONE',  ( -0.2756373558169954441, 0.9612616959383198934, -1.479773560108263204E-16 ) ) ;
#3755=VECTOR ( 'NONE', #19603, 1000.000000000000114 ) ;
#3759=CARTESIAN_POINT ( 'NONE',  ( -40.02540636251513462, 2.839176264122873050, 37.04930799450052348 ) ) ;
#3761=ORIENTED_EDGE ( 'NONE', *, *, #13645, .T. ) ;
#3764=VERTEX_POINT ( 'NONE', #16910 ) ;
#3767=ADVANCED_FACE ( 'NONE', ( #26930 ), #18710, .F. ) ;
#3779=CARTESIAN_POINT ( 'NONE',  ( -40.17244512953781310, 6.931285263614340053, 34.54930799450052348 ) ) ;
#3781=CARTESIAN_POINT ( 'NONE',  ( -40.41647043964083252, 8.356895951721259763, 59.64930799450051779 ) ) ;
#3783=FILL_AREA_STYLE ('',( #3461 ) ) ;
#3786=DIRECTION ( 'NONE',  ( 0.8746197071393925215, -0.4848096202463429982, -8.676864087101708112E-18 ) ) ;
#3789=TOROIDAL_SURFACE ( 'NONE', #16359, 0.2000000000000000111, 0.1000000000000000056 ) ;
#3790=ORIENTED_EDGE ( 'NONE', *, *, #5673, .F. ) ;
#3794=CARTESIAN_POINT ( 'NONE',  ( -36.38930206846553261, 9.511667899829566508, 59.64930799450051779 ) ) ;
#3801=ORIENTED_EDGE ( 'NONE', *, *, #29455, .F. ) ;
#3804=EDGE_CURVE ( 'NONE', #27622, #26389, #6424, .T. ) ;
#3814=SPHERICAL_SURFACE ( 'NONE', #25683, 0.1000000000000000056 ) ;
#3817=CARTESIAN_POINT ( 'NONE',  ( -40.58856461370174173, 7.499380836222961477, 53.94930799450051495 ) ) ;
#3830=EDGE_LOOP ( 'NONE', ( #3332, #16596, #29855, #32387, #24060, #13101 ) ) ;
#3832=CARTESIAN_POINT ( 'NONE',  ( -40.38516919650994197, 8.640923867788874446, 34.64930799450051779 ) ) ;
#3834=ORIENTED_EDGE ( 'NONE', *, *, #14912, .T. ) ;
#3837=DIRECTION ( 'NONE',  ( -0.8746197071393790878, 0.4848096202463673676, 1.277302113040196197E-17 ) ) ;
#3839=AXIS2_PLACEMENT_3D ( 'NONE', #30325, #2904, #12934 ) ;
#3847=ORIENTED_EDGE ( 'NONE', *, *, #6040, .F. ) ;
#3853=DIRECTION ( 'NONE',  ( 0.8746197071393926326, -0.4848096202463430537, -8.676864087101709653E-18 ) ) ;
#3858=DIRECTION ( 'NONE',  ( 0.8746197071393926326, -0.4848096202463430537, -8.676864087101709653E-18 ) ) ;
#3862=CARTESIAN_POINT ( 'NONE',  ( -40.54828680531408480, 6.846271790121642553, 34.54930799450052348 ) ) ;
#3868=DIRECTION ( 'NONE',  ( -0.9612616959383198934, -0.2756373558169956106, 0.000000000000000000 ) ) ;
#3873=CIRCLE ( 'NONE', #22212, 1.899999999999999023 ) ;
#3874=CARTESIAN_POINT ( 'NONE',  ( -42.36334586133935431, 13.70277685985800709, 54.62588685591540383 ) ) ;
#3876=CARTESIAN_POINT ( 'NONE',  ( -40.02353495526242710, 6.996741961792352527, 34.54930799450051637 ) ) ;
#3877=CARTESIAN_POINT ( 'NONE',  ( -40.56083369918835047, 7.405617721157512712, 35.30738027510436439 ) ) ;
#3885=CIRCLE ( 'NONE', #22223, 0.09999999999999774347 ) ;
#3888=AXIS2_PLACEMENT_3D ( 'NONE', #4950, #30225, #27593 ) ;
#3889=EDGE_CURVE ( 'NONE', #6416, #13529, #21989, .T. ) ;
#3890=ORIENTED_EDGE ( 'NONE', *, *, #848, .F. ) ;
#3893=DIRECTION ( 'NONE',  ( 0.000000000000000000, 1.517883041479704827E-15, -1.000000000000000000 ) ) ;
#3895=DIRECTION ( 'NONE',  ( 0.9612616959383206705, 0.2756373558169927240, 2.454997878969170293E-14 ) ) ;
#3896=DIRECTION ( 'NONE',  ( 0.1949050434465267878, -0.6797146636928667052, 0.7071067811865480168 ) ) ;
#3898=ORIENTED_EDGE ( 'NONE', *, *, #19488, .T. ) ;
#3899=ORIENTED_EDGE ( 'NONE', *, *, #18068, .T. ) ;
#3903=CARTESIAN_POINT ( 'NONE',  ( -40.59758774925372649, 7.567737757495682338, 38.66054537865625917 ) ) ;
#3907=AXIS2_PLACEMENT_3D ( 'NONE', #833, #30875, #17909 ) ;
#3909=FACE_OUTER_BOUND ( 'NONE', #20286, .T. ) ;
#3910=DIRECTION ( 'NONE',  ( 0.8746197071393926326, -0.4848096202463430537, -8.676864087101709653E-18 ) ) ;
#3914=FACE_BOUND ( 'NONE', #701, .T. ) ;
#3916=DIRECTION ( 'NONE',  ( 0.9612616959383205595, 0.2756373558169932236, -1.660411357259282445E-16 ) ) ;
#3923=ORIENTED_EDGE ( 'NONE', *, *, #32133, .F. ) ;
#3929=ADVANCED_FACE ( 'NONE', ( #15570 ), #17880, .T. ) ;
#3932=ORIENTED_EDGE ( 'NONE', *, *, #25696, .F. ) ;
#3933=EDGE_CURVE ( 'NONE', #17034, #31739, #10335, .T. ) ;
#3934=CIRCLE ( 'NONE', #21203, 0.09999999999999795164 ) ;
#3935=EDGE_CURVE ( 'NONE', #27622, #30194, #9457, .T. ) ;
#3948=ORIENTED_EDGE ( 'NONE', *, *, #29480, .F. ) ;
#3956=VECTOR ( 'NONE', #9637, 1000.000000000000114 ) ;
#3957=ORIENTED_EDGE ( 'NONE', *, *, #19251, .F. ) ;
#3961=CARTESIAN_POINT ( 'NONE',  ( -40.50726676055796105, 7.559560307024983494, 60.27956441091988182 ) ) ;
#3963=EDGE_CURVE ( 'NONE', #4744, #17141, #18339, .T. ) ;
#3971=DIRECTION ( 'NONE',  ( -0.7848668881104262640, -0.2250569586005336520, -0.5773502691896258421 ) ) ;
#3975=DIRECTION ( 'NONE',  ( 0.000000000000000000, 0.000000000000000000, 1.000000000000000000 ) ) ;
#3977=VECTOR ( 'NONE', #3786, 1000.000000000000114 ) ;
#3984=VERTEX_POINT ( 'NONE', #7878 ) ;
#3985=CARTESIAN_POINT ( 'NONE',  ( -39.58809650894544774, 2.596771453999702661, 47.04930799450051637 ) ) ;
#3992=ORIENTED_EDGE ( 'NONE', *, *, #3477, .T. ) ;
#3994=CARTESIAN_POINT ( 'NONE',  ( -40.23847960489091236, 6.935107575317838169, 39.54930799450052348 ) ) ;
#4004=CARTESIAN_POINT ( 'NONE',  ( -40.60330327974818232, 7.565477138576673255, 60.21714911875709220 ) ) ;
#4005=ORIENTED_EDGE ( 'NONE', *, *, #24067, .F. ) ;
#4006=AXIS2_PLACEMENT_3D ( 'NONE', #5579, #20826, #5740 ) ;
#4008=ORIENTED_EDGE ( 'NONE', *, *, #32492, .T. ) ;
#4016=ORIENTED_EDGE ( 'NONE', *, *, #3073, .T. ) ;
#4024=AXIS2_PLACEMENT_3D ( 'NONE', #24331, #19573, #11545 ) ;
#4026=ORIENTED_EDGE ( 'NONE', *, *, #14312, .F. ) ;
#4030=CARTESIAN_POINT ( 'NONE',  ( -40.69193635511749108, 9.347952559758585522, 39.54930799450052348 ) ) ;
#4039=FACE_OUTER_BOUND ( 'NONE', #9124, .T. ) ;
#4046=CARTESIAN_POINT ( 'NONE',  ( -40.91899271407989858, 10.13979218557001616, 37.04930799450052348 ) ) ;
#4051=DIRECTION ( 'NONE',  ( -0.9612616959383194493, -0.2756373558169974980, -8.795445018804946186E-19 ) ) ;
#4052=ADVANCED_FACE ( 'NONE', ( #14253 ), #21292, .T. ) ;
#4055=ORIENTED_EDGE ( 'NONE', *, *, #10445, .T. ) ;
#4059=DIRECTION ( 'NONE',  ( 0.000000000000000000, 0.000000000000000000, -1.000000000000000000 ) ) ;
#4060=DIRECTION ( 'NONE',  ( -2.779292025043186357E-18, 1.288349127009862211E-17, -1.000000000000000000 ) ) ;
#4066=ORIENTED_EDGE ( 'NONE', *, *, #26002, .F. ) ;
#4068=CARTESIAN_POINT ( 'NONE',  ( -43.64647580959332629, 1.256990871545142330, 60.44930799450051495 ) ) ;
#4069=AXIS2_PLACEMENT_3D ( 'NONE', #11640, #31502, #6552 ) ;
#4070=CARTESIAN_POINT ( 'NONE',  ( -40.11286833322908052, 2.887657226147511302, 57.04930799450051637 ) ) ;
#4071=AXIS2_PLACEMENT_3D ( 'NONE', #21137, #25916, #31175 ) ;
#4078=ORIENTED_EDGE ( 'NONE', *, *, #1662, .F. ) ;
#4087=CARTESIAN_POINT ( 'NONE',  ( -40.61685141166179136, 7.997713659873190828, 39.96793714460204683 ) ) ;
#4089=ORIENTED_EDGE ( 'NONE', *, *, #10087, .F. ) ;
#4091=LINE ( 'NONE', #9351, #15643 ) ;
#4094=ORIENTED_EDGE ( 'NONE', *, *, #14875, .F. ) ;
#4103=ORIENTED_EDGE ( 'NONE', *, *, #30107, .T. ) ;
#4105=DIRECTION ( 'NONE',  ( 0.8746197071393925215, -0.4848096202463429982, -8.676864087101708112E-18 ) ) ;
#4111=VERTEX_POINT ( 'NONE', #26713 ) ;
#4114=ADVANCED_FACE ( 'NONE', ( #6534 ), #23065, .T. ) ;
#4117=EDGE_CURVE ( 'NONE', #18405, #4732, #25187, .T. ) ;
#4123=AXIS2_PLACEMENT_3D ( 'NONE', #22239, #9455, #21910 ) ;
#4125=ORIENTED_EDGE ( 'NONE', *, *, #29280, .F. ) ;
#4126=FACE_OUTER_BOUND ( 'NONE', #31906, .T. ) ;
#4127=DIRECTION ( 'NONE',  ( 0.9612616959383145643, 0.2756373558170139848, 8.795445018807193747E-19 ) ) ;
#4128=DIRECTION ( 'NONE',  ( 0.8746197071393926326, -0.4848096202463430537, -8.676864087101709653E-18 ) ) ;
#4134=CARTESIAN_POINT ( 'NONE',  ( -40.18454328187963398, 7.548069831825862330, 53.64930799450051779 ) ) ;
#4139=LINE ( 'NONE', #27768, #25246 ) ;
#4140=DIRECTION ( 'NONE',  ( -0.8746197071393925215, 0.4848096202463429982, 8.676864087101708112E-18 ) ) ;
#4150=ORIENTED_EDGE ( 'NONE', *, *, #18011, .F. ) ;
#4154=LINE ( 'NONE', #7764, #6798 ) ;
#4155=ORIENTED_EDGE ( 'NONE', *, *, #11166, .F. ) ;
#4166=ORIENTED_EDGE ( 'NONE', *, *, #27096, .T. ) ;
#4168=EDGE_CURVE ( 'NONE', #10736, #16068, #7347, .T. ) ;
#4170=AXIS2_PLACEMENT_3D ( 'NONE', #1371, #11553, #9088 ) ;
#4179=DIRECTION ( 'NONE',  ( 0.2756373558170404081, -0.9612616959383071258, 1.479773560108186044E-16 ) ) ;
#4189=B_SPLINE_CURVE_WITH_KNOTS ( 'NONE', 3,
 ( #1270, #23925, #18670, #16057, #8681, #11453, #18823, #4237, #31806, #23609, #9316, #26714, #3579 ),
 .UNSPECIFIED., .F., .F.,
 ( 4, 3, 3, 3, 4 ),
 ( 0.000000000000000000, 3.644429809543512820E-05, 7.713354915361920658E-05, 0.0001101572536102696351, 0.0001291034991527052127 ),
 .UNSPECIFIED. ) ;
#4192=ORIENTED_EDGE ( 'NONE', *, *, #12171, .T. ) ;
#4193=CARTESIAN_POINT ( 'NONE',  ( -40.99628586177130529, 8.927770518203464789, 57.04930799450051637 ) ) ;
#4195=DIRECTION ( 'NONE',  ( 2.946248497964555786E-19, 3.001156285468303092E-19, 1.000000000000000000 ) ) ;
#4199=FACE_OUTER_BOUND ( 'NONE', #17319, .T. ) ;
#4200=DIRECTION ( 'NONE',  ( 0.9612616959383221138, 0.2756373558169876170, 0.000000000000000000 ) ) ;
#4204=AXIS2_PLACEMENT_3D ( 'NONE', #11785, #4060, #1122 ) ;
#4205=CIRCLE ( 'NONE', #26199, 0.1000000000000014905 ) ;
#4212=ORIENTED_EDGE ( 'NONE', *, *, #21642, .T. ) ;
#4216=CYLINDRICAL_SURFACE ( 'NONE', #2529, 0.1000000000000014905 ) ;
#4218=CIRCLE ( 'NONE', #15242, 0.1000000000000006301 ) ;
#4227=AXIS2_PLACEMENT_3D ( 'NONE', #5372, #15374, #7995 ) ;
#4230=DIRECTION ( 'NONE',  ( 0.2756373558169959437, -0.9612616959383197823, 0.000000000000000000 ) ) ;
#4237=CARTESIAN_POINT ( 'NONE',  ( -40.68879370032178144, 6.799057175545572207, 39.36235710484030648 ) ) ;
#4238=CARTESIAN_POINT ( 'NONE',  ( -40.52064562223811350, 7.631811404637807605, 60.17616806781843763 ) ) ;
#4247=DIRECTION ( 'NONE',  ( 2.779292025043186357E-18, -1.288349127009862211E-17, 1.000000000000000000 ) ) ;
#4249=FACE_OUTER_BOUND ( 'NONE', #4675, .T. ) ;
#4255=CIRCLE ( 'NONE', #6355, 0.09999999999999795164 ) ;
#4257=ADVANCED_FACE ( 'NONE', ( #9811 ), #19805, .F. ) ;
#4266=CARTESIAN_POINT ( 'NONE',  ( -38.41701585771487260, 6.978388747684010518, 62.04930799450052348 ) ) ;
#4268=ORIENTED_EDGE ( 'NONE', *, *, #7759, .T. ) ;
#4281=CARTESIAN_POINT ( 'NONE',  ( -42.38687957179150345, 4.148162238788003719, 58.94930799450051495 ) ) ;
#4285=DIRECTION ( 'NONE',  ( 0.4848096202463637039, 0.8746197071393810862, 0.000000000000000000 ) ) ;
#4289=VECTOR ( 'NONE', #25715, 1000.000000000000114 ) ;
#4290=DIRECTION ( 'NONE',  ( -0.2756373558169974980, 0.9612616959383193382, 1.315048337272770589E-17 ) ) ;
#4292=AXIS2_PLACEMENT_3D ( 'NONE', #30765, #18115, #27978 ) ;
#4296=CARTESIAN_POINT ( 'NONE',  ( -40.65065394966018175, 6.870367549600009838, 34.94083608680406172 ) ) ;
#4309=DIRECTION ( 'NONE',  ( 0.2756373558169973870, -0.9612616959383193382, -1.315048337272770280E-17 ) ) ;
#4311=CARTESIAN_POINT ( 'NONE',  ( -40.56598700578888383, 6.841196339308488028, 39.54930799450052348 ) ) ;
#4317=CARTESIAN_POINT ( 'NONE',  ( -40.15611298324447631, 6.923081382651430360, 34.55058768090939481 ) ) ;
#4319=ORIENTED_EDGE ( 'NONE', *, *, #13621, .T. ) ;
#4320=AXIS2_PLACEMENT_3D ( 'NONE', #30014, #25080, #22611 ) ;
#4323=DIRECTION ( 'NONE',  ( -0.4848096202463636484, -0.8746197071393810862, 0.000000000000000000 ) ) ;
#4324=ORIENTED_EDGE ( 'NONE', *, *, #14231, .F. ) ;
#4326=CARTESIAN_POINT ( 'NONE',  ( -40.11708823821248160, 6.803395581744264398, 39.44983305153184716 ) ) ;
#4330=DIRECTION ( 'NONE',  ( -0.9612616959383194493, -0.2756373558169972759, -8.795445018804905742E-19 ) ) ;
#4335=ORIENTED_EDGE ( 'NONE', *, *, #14948, .T. ) ;
#4338=DIRECTION ( 'NONE',  ( 0.9612616959383167847, 0.2756373558170070459, -6.299214802459322763E-15 ) ) ;
#4341=EDGE_CURVE ( 'NONE', #2499, #28788, #438, .T. ) ;
#4343=CYLINDRICAL_SURFACE ( 'NONE', #3475, 1.199999999999999734 ) ;
#4348=FACE_OUTER_BOUND ( 'NONE', #22661, .T. ) ;
#4349=VERTEX_POINT ( 'NONE', #5379 ) ;
#4352=CARTESIAN_POINT ( 'NONE',  ( -41.01929587258828747, 9.401204285752060130, 39.44930799450052206 ) ) ;
#4359=VECTOR ( 'NONE', #6059, 1000.000000000000114 ) ;
#4363=CIRCLE ( 'NONE', #8557, 0.09999999999999815981 ) ;
#4374=DIRECTION ( 'NONE',  ( 0.2756373558169926685, -0.9612616959383207815, -1.315048337272770743E-17 ) ) ;
#4376=ORIENTED_EDGE ( 'NONE', *, *, #29908, .F. ) ;
#4379=CARTESIAN_POINT ( 'NONE',  ( -39.67555847965937943, 2.645252416024336028, 45.84930799450051353 ) ) ;
#4380=CIRCLE ( 'NONE', #19038, 0.1000000000000018235 ) ;
#4382=DIRECTION ( 'NONE',  ( 0.000000000000000000, 0.000000000000000000, -1.000000000000000000 ) ) ;
#4385=CARTESIAN_POINT ( 'NONE',  ( -40.21210701746133509, 7.644196001419694575, 60.29072935073781991 ) ) ;
#4388=ORIENTED_EDGE ( 'NONE', *, *, #18409, .F. ) ;
#4390=DIRECTION ( 'NONE',  ( 0.000000000000000000, 0.000000000000000000, -1.000000000000000000 ) ) ;
#4393=CARTESIAN_POINT ( 'NONE',  ( -43.37834615508418068, 1.121909970995877082, 39.44930799450052916 ) ) ;
#4401=DIRECTION ( 'NONE',  ( -0.9612616959383198934, -0.2756373558169956106, 0.000000000000000000 ) ) ;
#4403=ADVANCED_FACE ( 'NONE', ( #20942 ), #16500, .T. ) ;
#4412=EDGE_CURVE ( 'NONE', #2185, #21311, #4218, .T. ) ;
#4421=ORIENTED_EDGE ( 'NONE', *, *, #10351, .T. ) ;
#4437=ADVANCED_FACE ( 'NONE', ( #29144 ), #8422, .T. ) ;
#4441=DIRECTION ( 'NONE',  ( -0.2756373558169956106, 0.9612616959383197823, 0.000000000000000000 ) ) ;
#4448=FACE_OUTER_BOUND ( 'NONE', #2255, .T. ) ;
#4455=VECTOR ( 'NONE', #27324, 1000.000000000000000 ) ;
#4462=VERTEX_POINT ( 'NONE', #23891 ) ;
#4463=DIRECTION ( 'NONE',  ( 0.9612616959383205595, 0.2756373558169932236, -1.660411357259282445E-16 ) ) ;
#4464=DIRECTION ( 'NONE',  ( 0.2756373558169954441, -0.9612616959383198934, 1.479773560108263204E-16 ) ) ;
#4465=CARTESIAN_POINT ( 'NONE',  ( -40.11286833322908052, 2.887657226147511302, 57.04930799450051637 ) ) ;
#4471=( BOUNDED_CURVE ( )  B_SPLINE_CURVE ( 3, ( #7914, #5770, #18388, #22992 ),
 .UNSPECIFIED., .F., .F. ) 
 B_SPLINE_CURVE_WITH_KNOTS ( ( 4, 4 ),
 ( 1.570796326794896558, 2.093319089163915070 ),
 .UNSPECIFIED. ) 
 CURVE ( )  GEOMETRIC_REPRESENTATION_ITEM ( )  RATIONAL_B_SPLINE_CURVE ( ( 1.000000000000000000, 0.9773766218976396303, 0.9773766218976396303, 1.000000000000000000 ) ) 
 REPRESENTATION_ITEM ( '' )  );
#4476=CIRCLE ( 'NONE', #2376, 1.500000000000001332 ) ;
#4477=B_SPLINE_CURVE_WITH_KNOTS ( 'NONE', 3,
 ( #27117, #26953, #32050, #17429, #2339, #4311, #12524 ),
 .UNSPECIFIED., .F., .F.,
 ( 4, 3, 4 ),
 ( 0.000000000000000000, 5.088378629326043544E-05, 0.0001059921926251528864 ),
 .UNSPECIFIED. ) ;
#4490=DIRECTION ( 'NONE',  ( -0.9612616959383221138, -0.2756373558169876170, 0.000000000000000000 ) ) ;
#4493=CIRCLE ( 'NONE', #28620, 1.042135311067126979 ) ;
#4494=ADVANCED_FACE ( 'NONE', ( #21409 ), #1086, .T. ) ;
#4498=ORIENTED_EDGE ( 'NONE', *, *, #5015, .T. ) ;
#4500=CIRCLE ( 'NONE', #2922, 1.300000000000002487 ) ;
#4506=EDGE_LOOP ( 'NONE', ( #3741, #1457, #31664, #1452 ) ) ;
#4508=VERTEX_POINT ( 'NONE', #11113 ) ;
#4511=CARTESIAN_POINT ( 'NONE',  ( -40.68921029693431279, 6.794170072703461294, 39.46947734395037344 ) ) ;
#4512=ORIENTED_EDGE ( 'NONE', *, *, #10803, .T. ) ;
#4521=CARTESIAN_POINT ( 'NONE',  ( -40.05987053574653345, 7.506472619680465641, 35.39279590939684539 ) ) ;
#4526=ADVANCED_FACE ( 'NONE', ( #6020 ), #13733, .T. ) ;
#4527=CARTESIAN_POINT ( 'NONE',  ( -40.90015969217747482, 8.955334253785164123, 56.14611646155296398 ) ) ;
#4532=ADVANCED_FACE ( 'NONE', ( #24534 ), #6820, .T. ) ;
#4535=ORIENTED_EDGE ( 'NONE', *, *, #1036, .T. ) ;
#4540=CARTESIAN_POINT ( 'NONE',  ( -42.32583647289406770, 13.67174551105522617, 59.52414500118048579 ) ) ;
#4541=DIRECTION ( 'NONE',  ( 0.8746197071393928546, -0.4848096202463424986, -1.277302113040826515E-17 ) ) ;
#4543=CARTESIAN_POINT ( 'NONE',  ( -40.02540636251513462, 2.839176264122873050, 37.04930799450052348 ) ) ;
#4551=CARTESIAN_POINT ( 'NONE',  ( -42.66751614955960292, 15.14923148629343430, 35.64930799450052490 ) ) ;
#4553=CARTESIAN_POINT ( 'NONE',  ( -41.08785830660041682, 9.277514380576530328, 39.54930799450052348 ) ) ;
#4559=VERTEX_POINT ( 'NONE', #32099 ) ;
#4567=EDGE_CURVE ( 'NONE', #27545, #27140, #11558, .T. ) ;
#4571=EDGE_CURVE ( 'NONE', #12082, #2410, #16796, .T. ) ;
#4572=DIRECTION ( 'NONE',  ( -0.2756373558169932236, 0.9612616959383205595, -1.479773560108267395E-16 ) ) ;
#4574=CARTESIAN_POINT ( 'NONE',  ( -48.34557642001920641, 3.861744873591483440, 60.44930799450051495 ) ) ;
#4583=DIRECTION ( 'NONE',  ( -0.8746197071393890798, 0.4848096202463489934, 8.676864087100840673E-18 ) ) ;
#4597=CARTESIAN_POINT ( 'NONE',  ( -42.28651568955962858, 14.71554561121750559, 58.98666529074791498 ) ) ;
#4599=AXIS2_PLACEMENT_3D ( 'NONE', #29951, #15487, #15329 ) ;
#4608=CARTESIAN_POINT ( 'NONE',  ( -42.36153388572594736, 13.68895619636815653, 60.54930799450051637 ) ) ;
#4609=TOROIDAL_SURFACE ( 'NONE', #13021, 0.8928932188134564019, 0.1000000000000000056 ) ;
#4616=CARTESIAN_POINT ( 'NONE',  ( -43.90780810587784089, -0.03953120679776400692, 62.04930799450052348 ) ) ;
#4628=DIRECTION ( 'NONE',  ( -0.7848668881104203798, -0.2250569586005539691, 0.5773502691896258421 ) ) ;
#4635=FACE_OUTER_BOUND ( 'NONE', #8262, .T. ) ;
#4640=CIRCLE ( 'NONE', #1491, 0.1000000000000008243 ) ;
#4646=DIRECTION ( 'NONE',  ( -0.4848096202463627602, -0.8746197071393815303, 0.000000000000000000 ) ) ;
#4647=CONICAL_SURFACE ( 'NONE', #9352, 0.9031915329475502796, 0.7853981633974456145 ) ;
#4651=CYLINDRICAL_SURFACE ( 'NONE', #16230, 1.500000000000001332 ) ;
#4659=CARTESIAN_POINT ( 'NONE',  ( -41.91739890389096956, 13.90674392281399818, 54.59993297551692848 ) ) ;
#4671=ORIENTED_EDGE ( 'NONE', *, *, #28166, .T. ) ;
#4672=DIRECTION ( 'NONE',  ( 0.8746197071393960742, -0.4848096202463368365, -1.277302113040707570E-17 ) ) ;
#4674=LINE ( 'NONE', #24528, #4455 ) ;
#4675=EDGE_LOOP ( 'NONE', ( #7524, #2544, #13091, #3923 ) ) ;
#4685=ORIENTED_EDGE ( 'NONE', *, *, #6793, .T. ) ;
#4686=B_SPLINE_CURVE_WITH_KNOTS ( 'NONE', 3,
 ( #3994, #6463, #16462, #11546, #26481, #22030, #20068, #30096 ),
 .UNSPECIFIED., .F., .F.,
 ( 4, 2, 2, 4 ),
 ( 0.000000000000000000, 0.0002558676349343736952, 0.0005117352698687473904, 0.001023470539737489360 ),
 .UNSPECIFIED. ) ;
#4688=B_SPLINE_CURVE_WITH_KNOTS ( 'NONE', 3,
 ( #26148, #28465, #3498, #1045, #11071, #11376, #21367, #21054, #32223, #24169, #22024, #2181, #6775, #2011, #9241, #27121, #12027, #26956, #16777 ),
 .UNSPECIFIED., .F., .F.,
 ( 4, 3, 3, 3, 3, 3, 4 ),
 ( -2.006352434653661683E-06, 0.000000000000000000, 4.188863878082995122E-05, 9.359854324831489748E-05, 0.0001315996560788412501, 0.0001581967873567794803, 0.0001850264499128575937 ),
 .UNSPECIFIED. ) ;
#4697=VECTOR ( 'NONE', #27385, 1000.000000000000000 ) ;
#4705=EDGE_CURVE ( 'NONE', #29664, #27773, #15343, .T. ) ;
#4706=EDGE_CURVE ( 'NONE', #26371, #23543, #30768, .T. ) ;
#4710=FACE_OUTER_BOUND ( 'NONE', #28962, .T. ) ;
#4718=CARTESIAN_POINT ( 'NONE',  ( -40.73091736380679606, 9.483895492497154578, 34.64930799450051779 ) ) ;
#4719=DIRECTION ( 'NONE',  ( -0.4848096202463424986, -0.8746197071393928546, 2.220446049250312834E-16 ) ) ;
#4726=DIRECTION ( 'NONE',  ( 0.2756373558169954441, -0.9612616959383198934, 1.479773560108263204E-16 ) ) ;
#4732=VERTEX_POINT ( 'NONE', #5497 ) ;
#4736=VERTEX_POINT ( 'NONE', #2864 ) ;
#4738=VECTOR ( 'NONE', #4309, 1000.000000000000000 ) ;
#4742=AXIS2_PLACEMENT_3D ( 'NONE', #4087, #24114, #1631 ) ;
#4743=VECTOR ( 'NONE', #7223, 1000.000000000000000 ) ;
#4744=VERTEX_POINT ( 'NONE', #563 ) ;
#4749=ORIENTED_EDGE ( 'NONE', *, *, #4945, .F. ) ;
#4758=EDGE_CURVE ( 'NONE', #22576, #22420, #2487, .T. ) ;
#4768=VERTEX_POINT ( 'NONE', #10425 ) ;
#4771=CARTESIAN_POINT ( 'NONE',  ( -41.34584395867850048, 11.59800658573647425, 56.14611646155296398 ) ) ;
#4785=ORIENTED_EDGE ( 'NONE', *, *, #1993, .T. ) ;
#4796=DIRECTION ( 'NONE',  ( 0.3428121700606596156, 0.6184495258776486759, 0.7071067811865566766 ) ) ;
#4798=CARTESIAN_POINT ( 'NONE',  ( -41.50472230201275181, 5.945882615091417911, 37.04930799450052348 ) ) ;
#4807=DIRECTION ( 'NONE',  ( -0.4848096202463408888, -0.8746197071393936318, 0.000000000000000000 ) ) ;
#4811=CARTESIAN_POINT ( 'NONE',  ( -41.02687597405218156, 7.220473278338834788, 60.44930799450051495 ) ) ;
#4813=EDGE_CURVE ( 'NONE', #31727, #31154, #12566, .T. ) ;
#4816=CARTESIAN_POINT ( 'NONE',  ( -40.28779227465695101, 2.984619150196775816, 37.04930799450052348 ) ) ;
#4818=DIRECTION ( 'NONE',  ( 0.4848096202463636484, 0.8746197071393810862, 0.000000000000000000 ) ) ;
#4819=EDGE_CURVE ( 'NONE', #31739, #10736, #17798, .T. ) ;
#4824=ORIENTED_EDGE ( 'NONE', *, *, #6569, .F. ) ;
#4826=EDGE_CURVE ( 'NONE', #24828, #21830, #20418, .T. ) ;
#4829=CARTESIAN_POINT ( 'NONE',  ( -40.80097511801616150, 8.246641009394465982, 59.44930799450051495 ) ) ;
#4830=AXIS2_PLACEMENT_3D ( 'NONE', #9608, #24371, #19604 ) ;
#4835=ADVANCED_FACE ( 'NONE', ( #3499 ), #6131, .F. ) ;
#4836=VECTOR ( 'NONE', #11983, 1000.000000000000114 ) ;
#4838=CARTESIAN_POINT ( 'NONE',  ( -40.57832940339291383, 7.446916344587776848, 60.29072935073781991 ) ) ;
#4842=DIRECTION ( 'NONE',  ( -0.4848096202463450521, -0.8746197071393914113, 0.000000000000000000 ) ) ;
#4860=ORIENTED_EDGE ( 'NONE', *, *, #29020, .F. ) ;
#4862=AXIS2_PLACEMENT_3D ( 'NONE', #15773, #503, #23324 ) ;
#4885=ORIENTED_EDGE ( 'NONE', *, *, #27048, .F. ) ;
#4908=VECTOR ( 'NONE', #16206, 1000.000000000000114 ) ;
#4922=VERTEX_POINT ( 'NONE', #3667 ) ;
#4925=CARTESIAN_POINT ( 'NONE',  ( -40.68765130478461600, 6.801118111650039211, 34.74701532369150669 ) ) ;
#4927=CARTESIAN_POINT ( 'NONE',  ( -40.06561427811386267, 7.496110634155836117, 58.05249952744806308 ) ) ;
#4930=ORIENTED_EDGE ( 'NONE', *, *, #21642, .F. ) ;
#4932=CARTESIAN_POINT ( 'NONE',  ( -42.47434154250544225, 4.196643200812637531, 55.14930799450051779 ) ) ;
#4934=CIRCLE ( 'NONE', #23277, 0.8928932188134552916 ) ;
#4939=CARTESIAN_POINT ( 'NONE',  ( -42.36691375901575185, 13.72999064396537250, 59.48380644099231773 ) ) ;
#4945=EDGE_CURVE ( 'NONE', #3387, #10137, #28068, .T. ) ;
#4946=ORIENTED_EDGE ( 'NONE', *, *, #9416, .T. ) ;
#4947=CIRCLE ( 'NONE', #23792, 0.1000000000000014905 ) ;
#4948=ORIENTED_EDGE ( 'NONE', *, *, #23276, .F. ) ;
#4950=CARTESIAN_POINT ( 'NONE',  ( -43.37834615508418068, 1.121909970995876193, 34.64930799450052490 ) ) ;
#4956=DIRECTION ( 'NONE',  ( 0.8746197071393926326, -0.4848096202463430537, -8.676864087101709653E-18 ) ) ;
#4957=CARTESIAN_POINT ( 'NONE',  ( -42.48178708409979265, 14.60617548783703690, 55.10133939125226021 ) ) ;
#4964=DIRECTION ( 'NONE',  ( -1.188208965918165239E-16, -1.880121038077813132E-16, -1.000000000000000000 ) ) ;
#4968=ORIENTED_EDGE ( 'NONE', *, *, #11647, .F. ) ;
#4977=DIRECTION ( 'NONE',  ( -0.9612616959383221138, -0.2756373558169876170, 0.000000000000000000 ) ) ;
#4982=CYLINDRICAL_SURFACE ( 'NONE', #534, 2.000000000000001776 ) ;
#4986=DIRECTION ( 'NONE',  ( -0.2756373558169954441, 0.9612616959383198934, -1.479773560108263204E-16 ) ) ;
#4987=CARTESIAN_POINT ( 'NONE',  ( -41.40207097079809984, 10.37330416413728962, 36.63067884439899302 ) ) ;
#4989=FACE_OUTER_BOUND ( 'NONE', #30709, .T. ) ;
#4991=EDGE_CURVE ( 'NONE', #14507, #1187, #21878, .T. ) ;
#4992=VERTEX_POINT ( 'NONE', #27290 ) ;
#4995=VECTOR ( 'NONE', #15408, 999.9999999999998863 ) ;
#5003=EDGE_LOOP ( 'NONE', ( #16613, #13069, #19012, #31542 ) ) ;
#5004=CARTESIAN_POINT ( 'NONE',  ( -40.83597905555367902, 8.457813048054211080, 34.59301614167199546 ) ) ;
#5006=VECTOR ( 'NONE', #19923, 1000.000000000000114 ) ;
#5007=LINE ( 'NONE', #15173, #15728 ) ;
#5008=DIRECTION ( 'NONE',  ( 0.4848096202463636484, 0.8746197071393810862, 0.000000000000000000 ) ) ;
#5009=CARTESIAN_POINT ( 'NONE',  ( -42.50084779003665147, 14.56798984196178637, 37.04930799450052348 ) ) ;
#5010=CARTESIAN_POINT ( 'NONE',  ( -41.73034863705382946, 11.48775164340967514, 57.04930799450051637 ) ) ;
#5011=ORIENTED_EDGE ( 'NONE', *, *, #2770, .T. ) ;
#5014=CARTESIAN_POINT ( 'NONE',  ( -48.24907229644473716, 10.92050229712533316, 59.54930799450050927 ) ) ;
#5015=EDGE_CURVE ( 'NONE', #1586, #15332, #29259, .T. ) ;
#5022=EDGE_LOOP ( 'NONE', ( #3418, #66, #29323, #28044 ) ) ;
#5025=ORIENTED_EDGE ( 'NONE', *, *, #8427, .T. ) ;
#5027=DIRECTION ( 'NONE',  ( 0.8746197071393925215, -0.4848096202463429982, -8.676864087101708112E-18 ) ) ;
#5029=EDGE_CURVE ( 'NONE', #2485, #32314, #29740, .T. ) ;
#5030=AXIS2_PLACEMENT_3D ( 'NONE', #1357, #19568, #31405 ) ;
#5036=CARTESIAN_POINT ( 'NONE',  ( -42.38687957179150345, 4.148162238788003719, 57.04930799450051637 ) ) ;
#5056=LINE ( 'NONE', #15066, #8960 ) ;
#5064=( BOUNDED_CURVE ( )  B_SPLINE_CURVE ( 3, ( #21412, #3874, #6823, #19276 ),
 .UNSPECIFIED., .F., .F. ) 
 B_SPLINE_CURVE_WITH_KNOTS ( ( 4, 4 ),
 ( 5.930963073318635814, 6.283185307179586232 ),
 .UNSPECIFIED. ) 
 CURVE ( )  GEOMETRIC_REPRESENTATION_ITEM ( )  RATIONAL_B_SPLINE_CURVE ( ( 1.000000000000000000, 0.9896883177220884287, 0.9896883177220884287, 1.000000000000000000 ) ) 
 REPRESENTATION_ITEM ( '' )  );
#5066=DIRECTION ( 'NONE',  ( -0.9612616959383313286, -0.2756373558169555871, 0.000000000000000000 ) ) ;
#5067=ORIENTED_EDGE ( 'NONE', *, *, #3322, .T. ) ;
#5069=CARTESIAN_POINT ( 'NONE',  ( -40.51565501380215295, 9.065589196111961456, 58.05249952744806308 ) ) ;
#5079=ORIENTED_EDGE ( 'NONE', *, *, #28399, .F. ) ;
#5080=ORIENTED_EDGE ( 'NONE', *, *, #5015, .F. ) ;
#5083=EDGE_LOOP ( 'NONE', ( #26210, #18236 ) ) ;
#5087=CARTESIAN_POINT ( 'NONE',  ( -39.58809650894544774, 2.596771453999702661, 48.24930799450051211 ) ) ;
#5088=FACE_OUTER_BOUND ( 'NONE', #5022, .T. ) ;
#5093=AXIS2_PLACEMENT_3D ( 'NONE', #29846, #19985, #2099 ) ;
#5096=VERTEX_POINT ( 'NONE', #2503 ) ;
#5101=AXIS2_PLACEMENT_3D ( 'NONE', #29298, #16329, #19443 ) ;
#5105=ORIENTED_EDGE ( 'NONE', *, *, #12586, .T. ) ;
#5106=CARTESIAN_POINT ( 'NONE',  ( -42.82457667231739151, 15.69696662191612901, 37.04930799450052348 ) ) ;
#5115=DIRECTION ( 'NONE',  ( -0.1949050434465281478, 0.6797146636928673713, 0.7071067811865469066 ) ) ;
#5120=FACE_OUTER_BOUND ( 'NONE', #15545, .T. ) ;
#5138=LINE ( 'NONE', #29598, #12054 ) ;
#5139=VERTEX_POINT ( 'NONE', #16062 ) ;
#5151=LINE ( 'NONE', #12876, #20346 ) ;
#5163=EDGE_CURVE ( 'NONE', #802, #11200, #23983, .T. ) ;
#5164=LINE ( 'NONE', #10582, #27783 ) ;
#5168=DIRECTION ( 'NONE',  ( -0.3428121700606640565, -0.6184495258776567805, -0.7071067811865474617 ) ) ;
#5171=ORIENTED_EDGE ( 'NONE', *, *, #22634, .F. ) ;
#5174=DIRECTION ( 'NONE',  ( 1.188208965918164993E-16, 1.880121038077812639E-16, 1.000000000000000000 ) ) ;
#5180=CARTESIAN_POINT ( 'NONE',  ( -41.07644103349282005, 9.237697617431789965, 39.54930799450052348 ) ) ;
#5187=EDGE_CURVE ( 'NONE', #180, #25211, #19161, .T. ) ;
#5189=AXIS2_PLACEMENT_3D ( 'NONE', #19362, #26761, #21828 ) ;
#5190=EDGE_CURVE ( 'NONE', #4111, #3549, #32396, .T. ) ;
#5198=DIRECTION ( 'NONE',  ( -0.3428121700606640565, -0.6184495258776567805, 0.7071067811865474617 ) ) ;
#5201=EDGE_CURVE ( 'NONE', #1586, #8660, #5657, .T. ) ;
#5202=ORIENTED_EDGE ( 'NONE', *, *, #31623, .T. ) ;
#5206=CARTESIAN_POINT ( 'NONE',  ( -40.74365851677129768, 8.439942589813739460, 34.54930799450052348 ) ) ;
#5214=CARTESIAN_POINT ( 'NONE',  ( -42.94875805865124363, 16.13003858227299858, 37.04930799450052348 ) ) ;
#5216=FACE_BOUND ( 'NONE', #30469, .T. ) ;
#5228=VERTEX_POINT ( 'NONE', #29029 ) ;
#5231=ADVANCED_FACE ( 'NONE', ( #26402 ), #26887, .T. ) ;
#5234=ORIENTED_EDGE ( 'NONE', *, *, #8234, .F. ) ;
#5251=CARTESIAN_POINT ( 'NONE',  ( -40.69332644341264427, 6.790879890547277142, 34.68541711214640344 ) ) ;
#5257=CIRCLE ( 'NONE', #31448, 0.1000000000000016709 ) ;
#5262=ADVANCED_FACE ( 'NONE', ( #14420, #11309, #24419, #6381 ), #11153, .F. ) ;
#5268=ADVANCED_FACE ( 'NONE', ( #3914, #23770 ), #31813, .T. ) ;
#5275=ORIENTED_EDGE ( 'NONE', *, *, #31211, .F. ) ;
#5277=ORIENTED_EDGE ( 'NONE', *, *, #31470, .T. ) ;
#5285=CYLINDRICAL_SURFACE ( 'NONE', #32424, 1.500000000000001332 ) ;
#5287=VECTOR ( 'NONE', #10305, 999.9999999999998863 ) ;
#5303=PLANE ( 'NONE',  #10426 ) ;
#5305=CARTESIAN_POINT ( 'NONE',  ( -42.73182147790732444, -0.8057266458565844891, 32.04930799450052348 ) ) ;
#5316=CARTESIAN_POINT ( 'NONE',  ( -40.28779227465695101, 2.984619150196775372, 38.54930799450052348 ) ) ;
#5321=VECTOR ( 'NONE', #20466, 1000.000000000000114 ) ;
#5325=EDGE_LOOP ( 'NONE', ( #29985, #18356, #28595, #24555 ) ) ;
#5327=CYLINDRICAL_SURFACE ( 'NONE', #8287, 0.1000000000000018235 ) ;
#5333=CARTESIAN_POINT ( 'NONE',  ( -40.60333149162104860, 7.557375771971046596, 60.54930799450051637 ) ) ;
#5334=FACE_BOUND ( 'NONE', #28285, .T. ) ;
#5340=FACE_OUTER_BOUND ( 'NONE', #26145, .T. ) ;
#5346=DIRECTION ( 'NONE',  ( 0.8746197071393926326, -0.4848096202463430537, -8.676864087101709653E-18 ) ) ;
#5347=CARTESIAN_POINT ( 'NONE',  ( -42.47434154250544225, 4.196643200812637531, 55.74930799450051211 ) ) ;
#5349=VECTOR ( 'NONE', #14655, 1000.000000000000114 ) ;
#5350=DIRECTION ( 'NONE',  ( 0.000000000000000000, 0.000000000000000000, -1.000000000000000000 ) ) ;
#5351=CARTESIAN_POINT ( 'NONE',  ( -39.64148344771002286, 7.657122216028890982, 32.14930799450051779 ) ) ;
#5353=DIRECTION ( 'NONE',  ( 0.000000000000000000, 0.000000000000000000, 1.000000000000000000 ) ) ;
#5355=CYLINDRICAL_SURFACE ( 'NONE', #9917, 0.1000000000000004774 ) ;
#5356=ORIENTED_EDGE ( 'NONE', *, *, #11202, .F. ) ;
#5360=EDGE_CURVE ( 'NONE', #16253, #9695, #22115, .T. ) ;
#5364=CARTESIAN_POINT ( 'NONE',  ( -42.35386648718987601, 15.27751306094253891, 38.53464782781823317 ) ) ;
#5365=CARTESIAN_POINT ( 'NONE',  ( -39.58809650894544774, 2.596771453999702661, 45.74930799450051211 ) ) ;
#5368=EDGE_LOOP ( 'NONE', ( #22289, #21422 ) ) ;
#5372=CARTESIAN_POINT ( 'NONE',  ( -40.48129536610376533, 8.613360132207176889, 39.44930799450052206 ) ) ;
#5373=ORIENTED_EDGE ( 'NONE', *, *, #3322, .F. ) ;
#5375=VERTEX_POINT ( 'NONE', #32470 ) ;
#5379=CARTESIAN_POINT ( 'NONE',  ( -40.10456357475989364, 7.631942973856654433, 53.94930799450051495 ) ) ;
#5380=LINE ( 'NONE', #3056, #2170 ) ;
#5384=LINE ( 'NONE', #2907, #25737 ) ;
#5385=DIRECTION ( 'NONE',  ( -2.779292025043186357E-18, 1.288349127009862211E-17, -1.000000000000000000 ) ) ;
#5389=EDGE_CURVE ( 'NONE', #26389, #27795, #17710, .T. ) ;
#5391=ORIENTED_EDGE ( 'NONE', *, *, #7539, .T. ) ;
#5393=ORIENTED_EDGE ( 'NONE', *, *, #437, .F. ) ;
#5401=EDGE_LOOP ( 'NONE', ( #10083, #925, #24751, #21289 ) ) ;
#5402=CARTESIAN_POINT ( 'NONE',  ( -40.02540636251514172, 2.839176264122877047, 57.04930799450051637 ) ) ;
#5405=CARTESIAN_POINT ( 'NONE',  ( -40.50720532202722524, 7.584939507552746818, 54.64930799450051779 ) ) ;
#5421=CARTESIAN_POINT ( 'NONE',  ( -40.73091736380679606, 9.483895492497154578, 38.64930799450052490 ) ) ;
#5446=FACE_BOUND ( 'NONE', #10809, .T. ) ;
#5448=LINE ( 'NONE', #15933, #25930 ) ;
#5450=CARTESIAN_POINT ( 'NONE',  ( -38.05567176388106532, 15.54312433976834740, 59.44930799450051495 ) ) ;
#5452=DIRECTION ( 'NONE',  ( 0.8746197071393925215, -0.4848096202463429982, -8.676864087101708112E-18 ) ) ;
#5453=LINE ( 'NONE', #18223, #1611 ) ;
#5455=DIRECTION ( 'NONE',  ( 0.4848096202463906268, 0.8746197071393660982, 0.000000000000000000 ) ) ;
#5458=ORIENTED_EDGE ( 'NONE', *, *, #31861, .F. ) ;
#5468=CARTESIAN_POINT ( 'NONE',  ( -40.02661603751083419, 7.039661056838938613, 39.27950010995386521 ) ) ;
#5470=ORIENTED_EDGE ( 'NONE', *, *, #31627, .F. ) ;
#5471=DIRECTION ( 'NONE',  ( 0.6797146636928687036, 0.1949050434465272041, 0.7071067811865459074 ) ) ;
#5475=CIRCLE ( 'NONE', #7045, 0.2000000000000004274 ) ;
#5480=EDGE_LOOP ( 'NONE', ( #3957, #16898, #30299, #11350 ) ) ;
#5484=LINE ( 'NONE', #232, #24109 ) ;
#5487=VECTOR ( 'NONE', #8387, 1000.000000000000114 ) ;
#5495=CARTESIAN_POINT ( 'NONE',  ( -41.56459318755936749, 7.281738416154046156, 53.54930799450051637 ) ) ;
#5497=CARTESIAN_POINT ( 'NONE',  ( -42.24141723705587737, 13.63285518870473290, 54.54930799450051637 ) ) ;
#5498=CIRCLE ( 'NONE', #21189, 1.042135311067126979 ) ;
#5499=EDGE_CURVE ( 'NONE', #3287, #13675, #11977, .T. ) ;
#5500=CARTESIAN_POINT ( 'NONE',  ( -40.64160980462626327, 6.824069488939680461, 39.41866629635870822 ) ) ;
#5503=CARTESIAN_POINT ( 'NONE',  ( -41.08785830660042393, 9.277514380576530328, 35.49072935073782986 ) ) ;
#5512=VERTEX_POINT ( 'NONE', #27870 ) ;
#5537=EDGE_CURVE ( 'NONE', #1639, #1830, #12940, .T. ) ;
#5541=ADVANCED_FACE ( 'NONE', ( #13102 ), #4647, .F. ) ;
#5562=EDGE_LOOP ( 'NONE', ( #8864, #8703, #24882 ) ) ;
#5567=EDGE_LOOP ( 'NONE', ( #8351, #15622, #32252, #22472 ) ) ;
#5568=LINE ( 'NONE', #22797, #11656 ) ;
#5569=VERTEX_POINT ( 'NONE', #8170 ) ;
#5570=AXIS2_PLACEMENT_3D ( 'NONE', #32407, #7466, #7131 ) ;
#5573=CARTESIAN_POINT ( 'NONE',  ( -40.59581018552366061, 9.375516295340284856, 39.44930799450052206 ) ) ;
#5579=CARTESIAN_POINT ( 'NONE',  ( -41.06741244844305783, 5.703477804968248854, 47.04930799450051637 ) ) ;
#5583=ORIENTED_EDGE ( 'NONE', *, *, #11807, .T. ) ;
#5591=ORIENTED_EDGE ( 'NONE', *, *, #18031, .F. ) ;
#5593=PLANE ( 'NONE',  #12869 ) ;
#5607=CARTESIAN_POINT ( 'NONE',  ( -42.12525683681430877, 14.70933063813549424, 38.19144330556764544 ) ) ;
#5616=DIRECTION ( 'NONE',  ( 0.8746197071393925215, -0.4848096202463429982, -8.676864087101709653E-18 ) ) ;
#5619=CARTESIAN_POINT ( 'NONE',  ( -40.01477201457414878, 7.207664580857849224, 39.00001346453329631 ) ) ;
#5620=ORIENTED_EDGE ( 'NONE', *, *, #5187, .F. ) ;
#5634=EDGE_CURVE ( 'NONE', #25363, #26371, #23899, .T. ) ;
#5638=DIRECTION ( 'NONE',  ( -0.8746197071393805311, 0.4848096202463645921, 1.277302113040265530E-17 ) ) ;
#5641=DIRECTION ( 'NONE',  ( 0.8746197071393925215, -0.4848096202463429982, -8.676864087101708112E-18 ) ) ;
#5643=CARTESIAN_POINT ( 'NONE',  ( -40.11286833322907341, 2.887657226147507306, 37.04930799450052348 ) ) ;
#5646=FACE_OUTER_BOUND ( 'NONE', #24588, .T. ) ;
#5648=FACE_OUTER_BOUND ( 'NONE', #11106, .T. ) ;
#5650=FACE_OUTER_BOUND ( 'NONE', #14035, .T. ) ;
#5652=CARTESIAN_POINT ( 'NONE',  ( -40.64500813507293486, 6.819128862114092193, 39.51928662074344345 ) ) ;
#5657=CIRCLE ( 'NONE', #16641, 0.1000000000000028644 ) ;
#5658=VERTEX_POINT ( 'NONE', #8796 ) ;
#5664=VERTEX_POINT ( 'NONE', #11121 ) ;
#5667=VERTEX_POINT ( 'NONE', #26035 ) ;
#5673=EDGE_CURVE ( 'NONE', #25118, #9995, #16669, .T. ) ;
#5676=FACE_OUTER_BOUND ( 'NONE', #7663, .T. ) ;
#5679=EDGE_LOOP ( 'NONE', ( #15652, #29644, #14384, #17961 ) ) ;
#5681=DIRECTION ( 'NONE',  ( 0.9612616959383202264, 0.2756373558169946114, -1.699334552409296294E-15 ) ) ;
#5690=CARTESIAN_POINT ( 'NONE',  ( -40.47970302497625994, 7.463434137431151250, 53.64930799450051779 ) ) ;
#5693=DIRECTION ( 'NONE',  ( -0.9862637841664568805, -0.1651779284337366038, 0.000000000000000000 ) ) ;
#5695=DIRECTION ( 'NONE',  ( -0.8746197071393925215, 0.4848096202463429982, 8.676864087101708112E-18 ) ) ;
#5699=CARTESIAN_POINT ( 'NONE',  ( -40.11286833322908052, 2.887657226147509970, 58.24930799450051921 ) ) ;
#5707=AXIS2_PLACEMENT_3D ( 'NONE', #12412, #22398, #1898 ) ;
#5710=CIRCLE ( 'NONE', #14100, 0.1000000000000027811 ) ;
#5712=EDGE_CURVE ( 'NONE', #607, #1905, #18957, .T. ) ;
#5734=LINE ( 'NONE', #13299, #4359 ) ;
#5735=AXIS2_PLACEMENT_3D ( 'NONE', #13465, #1453, #15915 ) ;
#5739=EDGE_LOOP ( 'NONE', ( #12672, #1802, #27125, #14542, #7934, #7788, #29464, #23905 ) ) ;
#5740=DIRECTION ( 'NONE',  ( 2.779292025043186357E-18, -1.288349127009862211E-17, 1.000000000000000000 ) ) ;
#5743=DIRECTION ( 'NONE',  ( 0.2756373558169954441, -0.9612616959383198934, 5.348665517716782531E-31 ) ) ;
#5745=CARTESIAN_POINT ( 'NONE',  ( -42.26497471389478733, 14.66834543456875117, 59.01654570186344984 ) ) ;
#5751=VECTOR ( 'NONE', #14510, 1000.000000000000000 ) ;
#5752=ORIENTED_EDGE ( 'NONE', *, *, #1626, .T. ) ;
#5759=DIRECTION ( 'NONE',  ( 0.7141240004913198547, -0.3958453973320100738, -0.5773502691896283956 ) ) ;
#5768=AXIS2_PLACEMENT_3D ( 'NONE', #26507, #11577, #24364 ) ;
#5770=CARTESIAN_POINT ( 'NONE',  ( -41.95414548415062228, 13.78332541096821373, 59.54930799450050927 ) ) ;
#5772=CARTESIAN_POINT ( 'NONE',  ( -39.58809650894544774, 2.596771453999702661, 47.04930799450051637 ) ) ;
#5774=CARTESIAN_POINT ( 'NONE',  ( -40.69224796978070202, 6.791021494070471398, 34.63467695428018800 ) ) ;
#5776=( LENGTH_UNIT ( ) NAMED_UNIT ( * ) SI_UNIT ( .MILLI., .METRE. ) );
#5780=LINE ( 'NONE', #8562, #22454 ) ;
#5787=CARTESIAN_POINT ( 'NONE',  ( -40.23847960489091236, 6.935107575317840833, 39.54930799450052348 ) ) ;
#5792=TOROIDAL_SURFACE ( 'NONE', #30436, 1.899999999999999467, 0.1000000000000000056 ) ;
#5797=AXIS2_PLACEMENT_3D ( 'NONE', #22347, #17260, #7434 ) ;
#5798=ORIENTED_EDGE ( 'NONE', *, *, #10542, .T. ) ;
#5800=FACE_OUTER_BOUND ( 'NONE', #25926, .T. ) ;
#5804=ORIENTED_EDGE ( 'NONE', *, *, #26569, .T. ) ;
#5807=CARTESIAN_POINT ( 'NONE',  ( -43.64073206722599707, 1.267352857069779848, 39.44930799450052916 ) ) ;
#5810=DIRECTION ( 'NONE',  ( -0.8746197071393895239, 0.4848096202463481053, 0.000000000000000000 ) ) ;
#5813=CARTESIAN_POINT ( 'NONE',  ( -40.62282199596570109, 7.625347238340325795, 53.94439779120587986 ) ) ;
#5815=EDGE_CURVE ( 'NONE', #3106, #12291, #19835, .T. ) ;
#5828=CARTESIAN_POINT ( 'NONE',  ( -39.85048242108726413, 2.742214340073605428, 45.54930799450051637 ) ) ;
#5833=EDGE_CURVE ( 'NONE', #9196, #8819, #14093, .T. ) ;
#5839=CARTESIAN_POINT ( 'NONE',  ( -40.59783212598355107, 7.538197204814858665, 60.10545411752895006 ) ) ;
#5842=CIRCLE ( 'NONE', #4227, 0.1000000000000024064 ) ;
#5847=AXIS2_PLACEMENT_3D ( 'NONE', #22050, #16957, #24689 ) ;
#5850=ORIENTED_EDGE ( 'NONE', *, *, #3104, .T. ) ;
#5852=VERTEX_POINT ( 'NONE', #5351 ) ;
#5854=CARTESIAN_POINT ( 'NONE',  ( -41.63422246745999189, 11.51531537899137447, 56.14611646155296398 ) ) ;
#5856=CARTESIAN_POINT ( 'NONE',  ( -40.47970302497626705, 7.463434137431151250, 53.80788663826320573 ) ) ;
#5859=CARTESIAN_POINT ( 'NONE',  ( -40.65487266620045403, 9.475231293617264683, 35.46144002885649371 ) ) ;
#5860=VECTOR ( 'NONE', #22384, 1000.000000000000000 ) ;
#5861=ORIENTED_EDGE ( 'NONE', *, *, #25008, .F. ) ;
#5863=ORIENTED_EDGE ( 'NONE', *, *, #26204, .T. ) ;
#5865=CARTESIAN_POINT ( 'NONE',  ( -42.36153388572594736, 13.68895619636815653, 54.64930799450051779 ) ) ;
#5867=CARTESIAN_POINT ( 'NONE',  ( -41.24971778908466291, 11.62557032131817181, 56.04611646155296256 ) ) ;
#5868=ADVANCED_FACE ( 'NONE', ( #30620 ), #20593, .F. ) ;
#5873=CARTESIAN_POINT ( 'NONE',  ( -41.94956971822180947, 3.905757428664830222, 45.84930799450051353 ) ) ;
#5875=ORIENTED_EDGE ( 'NONE', *, *, #17045, .T. ) ;
#5877=VECTOR ( 'NONE', #17011, 1000.000000000000114 ) ;
#5878=ADVANCED_FACE ( 'NONE', ( #12746 ), #18280, .T. ) ;
#5881=ORIENTED_EDGE ( 'NONE', *, *, #15437, .F. ) ;
#5885=AXIS2_PLACEMENT_3D ( 'NONE', #11872, #18916, #14339 ) ;
#5889=AXIS2_PLACEMENT_3D ( 'NONE', #17336, #27358, #20931 ) ;
#5890=CARTESIAN_POINT ( 'NONE',  ( -40.52669582637187773, 7.652910973922034010, 53.94439779120588696 ) ) ;
#5897=EDGE_LOOP ( 'NONE', ( #27475, #8813, #31328, #23417 ) ) ;
#5913=CARTESIAN_POINT ( 'NONE',  ( -40.59307405792753798, 7.534955460439823227, 53.80788663826319862 ) ) ;
#5921=CARTESIAN_POINT ( 'NONE',  ( -41.04685960816998147, 9.497330455345890599, 38.54930799450052348 ) ) ;
#5926=DIRECTION ( 'NONE',  ( 0.8746197071393926326, -0.4848096202463430537, -8.676864087101709653E-18 ) ) ;
#5929=DIRECTION ( 'NONE',  ( -1.188208965918165239E-16, -1.880121038077812639E-16, -1.000000000000000000 ) ) ;
#5937=CIRCLE ( 'NONE', #171, 0.9031915329475500576 ) ;
#5947=ORIENTED_EDGE ( 'NONE', *, *, #8224, .F. ) ;
#5950=CARTESIAN_POINT ( 'NONE',  ( -40.02327307428360115, 7.071123406435155800, 39.20438120789051339 ) ) ;
#5962=VERTEX_POINT ( 'NONE', #22893 ) ;
#5970=EDGE_CURVE ( 'NONE', #10137, #29664, #12018, .T. ) ;
#5973=CARTESIAN_POINT ( 'NONE',  ( -40.60922101150777053, 7.585765375989693915, 53.90260032368192356 ) ) ;
#5976=DIRECTION ( 'NONE',  ( 2.779292025043186357E-18, -1.288349127009862211E-17, 1.000000000000000000 ) ) ;
#5977=DIRECTION ( 'NONE',  ( 1.000000000000000000, 0.000000000000000000, 0.000000000000000000 ) ) ;
#5987=CARTESIAN_POINT ( 'NONE',  ( -40.14354458344919863, 7.767885906595227929, 53.80788663826320573 ) ) ;
#5993=ORIENTED_EDGE ( 'NONE', *, *, #1293, .T. ) ;
#6007=ORIENTED_EDGE ( 'NONE', *, *, #28795, .T. ) ;
#6013=EDGE_LOOP ( 'NONE', ( #31914, #11162, #31952, #2106 ) ) ;
#6014=DIRECTION ( 'NONE',  ( -0.1540342867254181347, 0.6907746437949939811, -0.7064728091037127955 ) ) ;
#6020=FACE_OUTER_BOUND ( 'NONE', #2896, .T. ) ;
#6022=CARTESIAN_POINT ( 'NONE',  ( -39.55402147699608406, 7.608641254004257171, 62.04930799450052348 ) ) ;
#6026=CARTESIAN_POINT ( 'NONE',  ( -40.54123211584830244, 7.002658380788985504, 35.02021009580667510 ) ) ;
#6031=ORIENTED_EDGE ( 'NONE', *, *, #747, .T. ) ;
#6036=VECTOR ( 'NONE', #13484, 1000.000000000000227 ) ;
#6040=EDGE_CURVE ( 'NONE', #655, #3764, #20910, .T. ) ;
#6047=AXIS2_PLACEMENT_3D ( 'NONE', #27066, #12471, #27401 ) ;
#6049=CYLINDRICAL_SURFACE ( 'NONE', #12764, 0.1000000000000020595 ) ;
#6051=ORIENTED_EDGE ( 'NONE', *, *, #1036, .F. ) ;
#6053=AXIS2_PLACEMENT_3D ( 'NONE', #11741, #14698, #9605 ) ;
#6059=DIRECTION ( 'NONE',  ( -0.3597811455230787714, 0.7883456110718085608, -0.4990678559373643575 ) ) ;
#6065=CARTESIAN_POINT ( 'NONE',  ( -40.60333149162104860, 7.557375771971046596, 60.54930799450051637 ) ) ;
#6068=CARTESIAN_POINT ( 'NONE',  ( -39.64148344771002286, 7.657122216028890982, 32.04930799450052348 ) ) ;
#6069=EDGE_LOOP ( 'NONE', ( #21799, #20289 ) ) ;
#6077=CARTESIAN_POINT ( 'NONE',  ( -41.10316901461906980, 9.481183992871798694, 38.54930799450053058 ) ) ;
#6078=DIRECTION ( 'NONE',  ( 0.9612616959383200044, 0.2756373558169954996, -1.660411357259285896E-16 ) ) ;
#6088=ORIENTED_EDGE ( 'NONE', *, *, #2990, .F. ) ;
#6092=EDGE_LOOP ( 'NONE', ( #31691, #5583, #25751 ) ) ;
#6102=FACE_OUTER_BOUND ( 'NONE', #30618, .T. ) ;
#6106=VERTEX_POINT ( 'NONE', #26643 ) ;
#6109=CARTESIAN_POINT ( 'NONE',  ( -40.02540636251514172, 2.839176264122877047, 57.04930799450051637 ) ) ;
#6114=ADVANCED_FACE ( 'NONE', ( #24017 ), #11233, .T. ) ;
#6116=EDGE_CURVE ( 'NONE', #15784, #13775, #23567, .T. ) ;
#6118=CARTESIAN_POINT ( 'NONE',  ( -42.38687957179149635, 4.148162238787999279, 37.04930799450052348 ) ) ;
#6122=ORIENTED_EDGE ( 'NONE', *, *, #23975, .T. ) ;
#6123=CARTESIAN_POINT ( 'NONE',  ( -41.94323192092818431, 13.80701548633532560, 54.55385885333559060 ) ) ;
#6127=ORIENTED_EDGE ( 'NONE', *, *, #11222, .T. ) ;
#6131=CYLINDRICAL_SURFACE ( 'NONE', #21343, 0.9999999999999998890 ) ;
#6141=DIRECTION ( 'NONE',  ( 0.9612616959383207815, 0.2756373558169926685, 8.795445018804291370E-19 ) ) ;
#6143=ORIENTED_EDGE ( 'NONE', *, *, #28320, .T. ) ;
#6148=AXIS2_PLACEMENT_3D ( 'NONE', #28900, #23797, #26427 ) ;
#6151=CIRCLE ( 'NONE', #20822, 0.1000000000000018235 ) ;
#6152=DIRECTION ( 'NONE',  ( 1.188208965918165239E-16, 1.880121038077813132E-16, 1.000000000000000000 ) ) ;
#6155=EDGE_CURVE ( 'NONE', #26286, #4992, #13093, .T. ) ;
#6157=ORIENTED_EDGE ( 'NONE', *, *, #24724, .T. ) ;
#6163=CARTESIAN_POINT ( 'NONE',  ( -43.37834615508418068, 1.121909970995877304, 39.44930799450052916 ) ) ;
#6171=TOROIDAL_SURFACE ( 'NONE', #14555, 1.524998423334081643, 0.1000000000000000056 ) ;
#6173=CARTESIAN_POINT ( 'NONE',  ( -42.38687957179149635, 4.148162238787999279, 37.04930799450052348 ) ) ;
#6175=ORIENTED_EDGE ( 'NONE', *, *, #27198, .T. ) ;
#6183=EDGE_CURVE ( 'NONE', #32001, #25278, #8876, .T. ) ;
#6184=AXIS2_PLACEMENT_3D ( 'NONE', #26175, #23553, #11252 ) ;
#6199=ORIENTED_EDGE ( 'NONE', *, *, #28797, .T. ) ;
#6201=EDGE_LOOP ( 'NONE', ( #26954, #137, #7730, #16190 ) ) ;
#6203=AXIS2_PLACEMENT_3D ( 'NONE', #9434, #27760, #342 ) ;
#6218=CARTESIAN_POINT ( 'NONE',  ( -40.05987053574653345, 7.506472619680472746, 38.19144330556764544 ) ) ;
#6226=CARTESIAN_POINT ( 'NONE',  ( -41.92347351173194170, 13.84990507184044084, 59.52701028453313370 ) ) ;
#6227=CARTESIAN_POINT ( 'NONE',  ( -40.67837904183828357, 9.488261090400158082, 35.45356819842893259 ) ) ;
#6230=ADVANCED_FACE ( 'NONE', ( #19242 ), #4651, .T. ) ;
#6233=CIRCLE ( 'NONE', #7812, 1.500000000000001332 ) ;
#6235=FACE_OUTER_BOUND ( 'NONE', #32152, .T. ) ;
#6242=DIRECTION ( 'NONE',  ( -0.8746197071393805311, 0.4848096202463645921, 1.277302113040265530E-17 ) ) ;
#6247=CARTESIAN_POINT ( 'NONE',  ( -42.48178708409979265, 14.60617548783703690, 58.99727659774876543 ) ) ;
#6252=ORIENTED_EDGE ( 'NONE', *, *, #1550, .F. ) ;
#6256=AXIS2_PLACEMENT_3D ( 'NONE', #15990, #14184, #9087 ) ;
#6264=EDGE_CURVE ( 'NONE', #1774, #10919, #1494, .T. ) ;
#6266=CIRCLE ( 'NONE', #17269, 1.899999999999999023 ) ;
#6272=LINE ( 'NONE', #31232, #24111 ) ;
#6275=ORIENTED_EDGE ( 'NONE', *, *, #28637, .T. ) ;
#6276=CARTESIAN_POINT ( 'NONE',  ( -42.03703168893574116, 3.954238390689463145, 47.04930799450051637 ) ) ;
#6277=CARTESIAN_POINT ( 'NONE',  ( -41.07644103349281295, 9.237697617431788188, 34.64930799450051779 ) ) ;
#6283=CARTESIAN_POINT ( 'NONE',  ( -40.61574147496721565, 7.605736927813537385, 53.92359549476551450 ) ) ;
#6286=CARTESIAN_POINT ( 'NONE',  ( 0.000000000000000000, 0.000000000000000000, 0.000000000000000000 ) ) ;
#6287=ORIENTED_EDGE ( 'NONE', *, *, #14382, .T. ) ;
#6289=CARTESIAN_POINT ( 'NONE',  ( -40.02540636251513462, 2.839176264122873050, 37.04930799450052348 ) ) ;
#6292=CARTESIAN_POINT ( 'NONE',  ( -40.11902961310587301, 6.880801488287905165, 34.57491199848074359 ) ) ;
#6300=FACE_OUTER_BOUND ( 'NONE', #19576, .T. ) ;
#6303=CARTESIAN_POINT ( 'NONE',  ( -40.50410981870283678, 7.604537000166497585, 38.76008276981544753 ) ) ;
#6319=ORIENTED_EDGE ( 'NONE', *, *, #10123, .T. ) ;
#6323=FACE_OUTER_BOUND ( 'NONE', #21519, .T. ) ;
#6324=DIRECTION ( 'NONE',  ( -0.9612616959383200044, -0.2756373558169956106, -8.795445018804684260E-19 ) ) ;
#6326=CARTESIAN_POINT ( 'NONE',  ( -41.77464577679392477, 3.808795504615560379, 47.04930799450051637 ) ) ;
#6330=ORIENTED_EDGE ( 'NONE', *, *, #18728, .T. ) ;
#6336=VERTEX_POINT ( 'NONE', #17075 ) ;
#6340=CIRCLE ( 'NONE', #13169, 0.1000000000000028644 ) ;
#6342=CONICAL_SURFACE ( 'NONE', #10551, 0.9031915329475500576, 0.7853981633974548293 ) ;
#6349=VERTEX_POINT ( 'NONE', #19204 ) ;
#6355=AXIS2_PLACEMENT_3D ( 'NONE', #7636, #12730, #17628 ) ;
#6356=DIRECTION ( 'NONE',  ( 0.8746197071393925215, -0.4848096202463429982, -8.676864087101708112E-18 ) ) ;
#6364=CARTESIAN_POINT ( 'NONE',  ( -40.50726676055796105, 7.559560307024983494, 53.80788663826320573 ) ) ;
#6369=FACE_OUTER_BOUND ( 'NONE', #8986, .T. ) ;
#6371=ADVANCED_FACE ( 'NONE', ( #14795 ), #328, .T. ) ;
#6374=DIRECTION ( 'NONE',  ( -0.4848096202463429982, -0.8746197071393925215, -9.920727850371698576E-18 ) ) ;
#6381=FACE_BOUND ( 'NONE', #16204, .T. ) ;
#6382=DIRECTION ( 'NONE',  ( -0.2603858710390614672, 0.9080734476337354311, 0.3280271511107134552 ) ) ;
#6399=VECTOR ( 'NONE', #14933, 1000.000000000000114 ) ;
#6401=VERTEX_POINT ( 'NONE', #8059 ) ;
#6409=VERTEX_POINT ( 'NONE', #27425 ) ;
#6411=CARTESIAN_POINT ( 'NONE',  ( -42.41019933908752648, 14.71530103803245915, 58.95721942880052779 ) ) ;
#6414=CARTESIAN_POINT ( 'NONE',  ( -40.61463551858322063, 9.441168033762318501, 38.61901908761456781 ) ) ;
#6416=VERTEX_POINT ( 'NONE', #30373 ) ;
#6424=LINE ( 'NONE', #1165, #28290 ) ;
#6425=CIRCLE ( 'NONE', #6960, 1.199999999999999734 ) ;
#6426=ORIENTED_EDGE ( 'NONE', *, *, #7421, .T. ) ;
#6432=AXIS2_PLACEMENT_3D ( 'NONE', #31461, #29312, #12087 ) ;
#6433=ORIENTED_EDGE ( 'NONE', *, *, #5712, .F. ) ;
#6436=CARTESIAN_POINT ( 'NONE',  ( -40.49636040740121956, 6.939949491715667662, 39.44930799450052206 ) ) ;
#6437=DIRECTION ( 'NONE',  ( 0.4848096202463673676, 0.8746197071393789768, 0.000000000000000000 ) ) ;
#6447=DIRECTION ( 'NONE',  ( 0.2756373558169932236, -0.9612616959383206705, 1.479773560108267395E-16 ) ) ;
#6449=CYLINDRICAL_SURFACE ( 'NONE', #26205, 1.000000000000000666 ) ;
#6451=AXIS2_PLACEMENT_3D ( 'NONE', #7320, #27342, #22399 ) ;
#6457=B_SPLINE_CURVE_WITH_KNOTS ( 'NONE', 3,
 ( #20586, #23374, #25832, #23214, #30453, #15828, #731, #15658, #5500, #5652 ),
 .UNSPECIFIED., .F., .F.,
 ( 4, 2, 2, 2, 4 ),
 ( 0.000000000000000000, 0.0002984299662232473113, 0.0005968599324464946227, 0.0008952898986697419882, 0.001193719864892989245 ),
 .UNSPECIFIED. ) ;
#6462=CARTESIAN_POINT ( 'NONE',  ( -43.64647580959332629, 1.256990871545143440, 53.64930799450051779 ) ) ;
#6463=CARTESIAN_POINT ( 'NONE',  ( -40.23847960489091946, 6.935107575317837281, 39.46395734157443513 ) ) ;
#6466=CARTESIAN_POINT ( 'NONE',  ( -42.22138300640814634, 14.68176690255379491, 38.19144330556764544 ) ) ;
#6468=CARTESIAN_POINT ( 'NONE',  ( -43.86882709718853590, -0.1754741395363378920, 62.04930799450052348 ) ) ;
#6470=AXIS2_PLACEMENT_3D ( 'NONE', #32138, #30005, #27535 ) ;
#6476=CIRCLE ( 'NONE', #18528, 0.1000000000000018235 ) ;
#6488=CYLINDRICAL_SURFACE ( 'NONE', #5768, 0.1000000000000028644 ) ;
#6496=CARTESIAN_POINT ( 'NONE',  ( -42.47434154250543514, 4.196643200812633978, 37.04930799450052348 ) ) ;
#6497=DIRECTION ( 'NONE',  ( 0.1949050434465282866, -0.6797146636928672603, 0.7071067811865470176 ) ) ;
#6502=ORIENTED_EDGE ( 'NONE', *, *, #29120, .F. ) ;
#6505=ORIENTED_EDGE ( 'NONE', *, *, #22067, .T. ) ;
#6506=DIRECTION ( 'NONE',  ( -0.8746197071393926326, 0.4848096202463430537, 8.676864087101709653E-18 ) ) ;
#6509=ORIENTED_EDGE ( 'NONE', *, *, #27057, .F. ) ;
#6511=ORIENTED_EDGE ( 'NONE', *, *, #15358, .F. ) ;
#6512=TOROIDAL_SURFACE ( 'NONE', #26419, 1.899999999999999467, 0.1000000000000000056 ) ;
#6516=CARTESIAN_POINT ( 'NONE',  ( -41.61831254958298132, 11.12742816935064560, 38.19144330556764544 ) ) ;
#6517=ADVANCED_FACE ( 'NONE', ( #2796 ), #7367, .T. ) ;
#6532=EDGE_LOOP ( 'NONE', ( #21168, #6426, #3132, #10164 ) ) ;
#6533=CARTESIAN_POINT ( 'NONE',  ( -41.01929587258828747, 9.401204285752058354, 35.44930799450052206 ) ) ;
#6534=FACE_OUTER_BOUND ( 'NONE', #10532, .T. ) ;
#6538=AXIS2_PLACEMENT_3D ( 'NONE', #1468, #6242, #9026 ) ;
#6540=LINE ( 'NONE', #19647, #32142 ) ;
#6547=VECTOR ( 'NONE', #9706, 1000.000000000000114 ) ;
#6552=DIRECTION ( 'NONE',  ( 7.588956326749211550E-18, -4.206627182996911684E-18, 1.000000000000000000 ) ) ;
#6557=EDGE_CURVE ( 'NONE', #7574, #4462, #8415, .T. ) ;
#6568=CARTESIAN_POINT ( 'NONE',  ( -40.32034427004700916, 8.384459687302960873, 54.64930799450051779 ) ) ;
#6569=EDGE_CURVE ( 'NONE', #7978, #21737, #4640, .T. ) ;
#6575=EDGE_LOOP ( 'NONE', ( #28199, #7165, #2695, #24685 ) ) ;
#6579=EDGE_LOOP ( 'NONE', ( #10713, #29263, #4150, #31946, #4860 ) ) ;
#6589=DIRECTION ( 'NONE',  ( 0.9612616959383205595, 0.2756373558169932791, -1.660411357259282445E-16 ) ) ;
#6591=EDGE_CURVE ( 'NONE', #13209, #8738, #15116, .T. ) ;
#6596=AXIS2_PLACEMENT_3D ( 'NONE', #15521, #6152, #15850 ) ;
#6599=DIRECTION ( 'NONE',  ( 0.9612616959383205595, 0.2756373558169931681, -1.660411357259282445E-16 ) ) ;
#6600=CARTESIAN_POINT ( 'NONE',  ( -42.66751614955960292, 15.14923148629343430, 35.64930799450052490 ) ) ;
#6602=ORIENTED_EDGE ( 'NONE', *, *, #25671, .F. ) ;
#6603=CARTESIAN_POINT ( 'NONE',  ( -40.14354458344919863, 7.767885906595227929, 60.29072935073781991 ) ) ;
#6606=AXIS2_PLACEMENT_3D ( 'NONE', #23172, #18078, #1005 ) ;
#6611=DIRECTION ( 'NONE',  ( 0.2756373558169959437, -0.9612616959383197823, 0.000000000000000000 ) ) ;
#6612=CARTESIAN_POINT ( 'NONE',  ( -40.47970302497625994, 7.463434137431150361, 60.54930799450051637 ) ) ;
#6619=VECTOR ( 'NONE', #14688, 1000.000000000000000 ) ;
#6626=VERTEX_POINT ( 'NONE', #5745 ) ;
#6634=ORIENTED_EDGE ( 'NONE', *, *, #809, .T. ) ;
#6638=ADVANCED_FACE ( 'NONE', ( #19170 ), #9014, .T. ) ;
#6647=ORIENTED_EDGE ( 'NONE', *, *, #22018, .T. ) ;
#6652=CARTESIAN_POINT ( 'NONE',  ( -41.52218637998914375, 11.15499190493234494, 38.19144330556764544 ) ) ;
#6660=FACE_OUTER_BOUND ( 'NONE', #26848, .T. ) ;
#6663=CYLINDRICAL_SURFACE ( 'NONE', #25894, 0.1000000000000018235 ) ;
#6671=ADVANCED_FACE ( 'NONE', ( #19005 ), #23518, .T. ) ;
#6674=TOROIDAL_SURFACE ( 'NONE', #19235, 1.142135311067127068, 0.1000000000000000056 ) ;
#6678=CARTESIAN_POINT ( 'NONE',  ( -41.91739890389096956, 13.90674392281399818, 54.59993297551692848 ) ) ;
#6687=ORIENTED_EDGE ( 'NONE', *, *, #22373, .T. ) ;
#6692=DIRECTION ( 'NONE',  ( 0.000000000000000000, 0.000000000000000000, 1.000000000000000000 ) ) ;
#6696=LINE ( 'NONE', #24580, #32159 ) ;
#6700=VECTOR ( 'NONE', #25858, 1000.000000000000000 ) ;
#6705=DIRECTION ( 'NONE',  ( 0.8746197071393925215, -0.4848096202463429982, -8.676864087101708112E-18 ) ) ;
#6708=CARTESIAN_POINT ( 'NONE',  ( -42.32583647289407480, 13.67174551105522617, 54.57447098782054695 ) ) ;
#6717=AXIS2_PLACEMENT_3D ( 'NONE', #6436, #18416, #26295 ) ;
#6718=DIRECTION ( 'NONE',  ( -0.1949050434465251780, 0.6797146636928671493, -0.7071067811865481278 ) ) ;
#6724=DIRECTION ( 'NONE',  ( -1.188208965918165239E-16, -1.880121038077813132E-16, -1.000000000000000000 ) ) ;
#6729=AXIS2_PLACEMENT_3D ( 'NONE', #21851, #6924, #26784 ) ;
#6738=FACE_OUTER_BOUND ( 'NONE', #28916, .T. ) ;
#6747=AXIS2_PLACEMENT_3D ( 'NONE', #20190, #20514, #30542 ) ;
#6748=LINE ( 'NONE', #9378, #14878 ) ;
#6751=ADVANCED_FACE ( 'NONE', ( #24267 ), #9334, .T. ) ;
#6752=EDGE_CURVE ( 'NONE', #19450, #24287, #27509, .T. ) ;
#6753=AXIS2_PLACEMENT_3D ( 'NONE', #7234, #32348, #19858 ) ;
#6754=VERTEX_POINT ( 'NONE', #15037 ) ;
#6756=CARTESIAN_POINT ( 'NONE',  ( -42.38687957179149635, 4.148162238787999279, 37.04930799450052348 ) ) ;
#6762=CARTESIAN_POINT ( 'NONE',  ( -40.13606231985500017, 7.635531802539801127, 53.80788663826320573 ) ) ;
#6763=AXIS2_PLACEMENT_3D ( 'NONE', #5402, #22942, #466 ) ;
#6771=ORIENTED_EDGE ( 'NONE', *, *, #17859, .F. ) ;
#6772=EDGE_CURVE ( 'NONE', #30637, #6106, #25041, .T. ) ;
#6775=CARTESIAN_POINT ( 'NONE',  ( -40.41141501439636841, 8.548644083377668679, 34.56232498761289662 ) ) ;
#6776=CARTESIAN_POINT ( 'NONE',  ( -40.61178118339597631, 9.038025460530262123, 57.04930799450051637 ) ) ;
#6779=ORIENTED_EDGE ( 'NONE', *, *, #1550, .T. ) ;
#6782=DIRECTION ( 'NONE',  ( -0.8746197071393895239, 0.4848096202463481053, 0.000000000000000000 ) ) ;
#6786=CARTESIAN_POINT ( 'NONE',  ( -40.14234630318158281, 6.912323292265333485, 39.54347762122440457 ) ) ;
#6791=CARTESIAN_POINT ( 'NONE',  ( -40.51045226066063520, 7.589116544599138869, 60.22001867261916885 ) ) ;
#6793=EDGE_CURVE ( 'NONE', #30739, #17357, #6233, .T. ) ;
#6795=AXIS2_PLACEMENT_3D ( 'NONE', #15512, #30775, #887 ) ;
#6798=VECTOR ( 'NONE', #12374, 1000.000000000000114 ) ;
#6801=EDGE_CURVE ( 'NONE', #4992, #24759, #19313, .T. ) ;
#6802=DIRECTION ( 'NONE',  ( 0.2756373558169946114, -0.9612616959383201154, 3.004509245426093872E-15 ) ) ;
#6804=DIRECTION ( 'NONE',  ( -0.8746197071393926326, 0.4848096202463430537, 8.676864087101709653E-18 ) ) ;
#6809=ORIENTED_EDGE ( 'NONE', *, *, #5673, .T. ) ;
#6814=EDGE_CURVE ( 'NONE', #14753, #7068, #13389, .T. ) ;
#6819=CARTESIAN_POINT ( 'NONE',  ( -43.64073206722599707, 1.267352857069779848, 39.44930799450052916 ) ) ;
#6820=CYLINDRICAL_SURFACE ( 'NONE', #28346, 0.1000000000000018235 ) ;
#6821=CARTESIAN_POINT ( 'NONE',  ( -40.65235181538429288, 9.419364959807719373, 39.50704302141948432 ) ) ;
#6822=ADVANCED_FACE ( 'NONE', ( #27997 ), #5355, .T. ) ;
#6823=CARTESIAN_POINT ( 'NONE',  ( -42.36153388572594025, 13.68895619636815475, 54.63750615257477961 ) ) ;
#6825=CARTESIAN_POINT ( 'NONE',  ( -40.02353495282660845, 6.996741953892291477, 34.61178260766359926 ) ) ;
#6827=ORIENTED_EDGE ( 'NONE', *, *, #30719, .T. ) ;
#6835=CIRCLE ( 'NONE', #23602, 0.1000000000000014905 ) ;
#6836=EDGE_CURVE ( 'NONE', #30572, #8513, #22740, .T. ) ;
#6837=AXIS2_PLACEMENT_3D ( 'NONE', #4816, #32066, #14837 ) ;
#6839=EDGE_LOOP ( 'NONE', ( #27466, #20610, #8824, #22255 ) ) ;
#6842=PLANE ( 'NONE',  #26632 ) ;
#6846=ORIENTED_EDGE ( 'NONE', *, *, #12619, .F. ) ;
#6849=VECTOR ( 'NONE', #25590, 1000.000000000000114 ) ;
#6855=DIRECTION ( 'NONE',  ( -0.9612616959383200044, -0.2756373558169954996, 1.660411357259285896E-16 ) ) ;
#6857=LINE ( 'NONE', #14248, #31593 ) ;
#6862=FACE_OUTER_BOUND ( 'NONE', #3256, .T. ) ;
#6864=DIRECTION ( 'NONE',  ( 0.1949050434465276760, -0.6797146636928699248, -0.7071067811865447972 ) ) ;
#6868=PLANE ( 'NONE',  #26366 ) ;
#6880=CARTESIAN_POINT ( 'NONE',  ( -42.38687957179149635, 4.148162238787999279, 37.04930799450052348 ) ) ;
#6883=AXIS2_PLACEMENT_3D ( 'NONE', #6612, #8591, #9237 ) ;
#6884=VECTOR ( 'NONE', #12243, 1000.000000000000000 ) ;
#6886=DIRECTION ( 'NONE',  ( -0.9612616959383213366, -0.2756373558169906701, 9.294164490659098336E-15 ) ) ;
#6887=DIRECTION ( 'NONE',  ( 0.1949050434465267045, -0.6797146636928664831, -0.7071067811865482389 ) ) ;
#6889=AXIS2_PLACEMENT_3D ( 'NONE', #6961, #27312, #2368 ) ;
#6905=ORIENTED_EDGE ( 'NONE', *, *, #3104, .F. ) ;
#6907=LINE ( 'NONE', #32014, #30865 ) ;
#6917=B_SPLINE_CURVE_WITH_KNOTS ( 'NONE', 3,
 ( #14369, #24366, #1883, #21896, #2216, #22062, #26998, #4511, #27153, #15499, #7961, #17793, #10101, #15651, #20094, #30123, #10264, #557, #13214 ),
 .UNSPECIFIED., .F., .F.,
 ( 4, 3, 3, 3, 3, 3, 4 ),
 ( 5.204170427930421283E-17, 4.880491127589490851E-05, 6.736105324526939382E-05, 7.908518729062757934E-05, 8.835348272573385604E-05, 9.246404311662424498E-05, 9.397889733287322230E-05 ),
 .UNSPECIFIED. ) ;
#6920=DIRECTION ( 'NONE',  ( -0.2756373558169947779, 0.9612616959383200044, 0.000000000000000000 ) ) ;
#6924=DIRECTION ( 'NONE',  ( 0.1949050434465265935, -0.6797146636928685925, -0.7071067811865462405 ) ) ;
#6933=EDGE_CURVE ( 'NONE', #22591, #29694, #30625, .T. ) ;
#6936=ADVANCED_FACE ( 'NONE', ( #18284 ), #14926, .T. ) ;
#6945=AXIS2_PLACEMENT_3D ( 'NONE', #2828, #23935, #31499 ) ;
#6949=ORIENTED_EDGE ( 'NONE', *, *, #24383, .T. ) ;
#6950=EDGE_LOOP ( 'NONE', ( #22748, #22333, #11949, #11853 ) ) ;
#6951=CARTESIAN_POINT ( 'NONE',  ( -40.65093765668705572, 9.567768634527945792, 35.64930799450052490 ) ) ;
#6953=CARTESIAN_POINT ( 'NONE',  ( -42.60588768478345401, 14.57151196022700290, 38.19144330556764544 ) ) ;
#6955=ORIENTED_EDGE ( 'NONE', *, *, #28426, .T. ) ;
#6960=AXIS2_PLACEMENT_3D ( 'NONE', #23157, #16244, #14119 ) ;
#6961=CARTESIAN_POINT ( 'NONE',  ( -41.24971778908466291, 11.62557032131817181, 57.04930799450051637 ) ) ;
#6965=( BOUNDED_SURFACE ( )  B_SPLINE_SURFACE ( 3, 2, ( 
 ( #17424, #12520, #22994 ),
 ( #25143, #20213, #2969 ),
 ( #7261, #27603, #10541 ),
 ( #22835, #30236, #10372 ) ),
 .UNSPECIFIED., .F., .F., .F. ) 
 B_SPLINE_SURFACE_WITH_KNOTS ( ( 4, 4 ),
 ( 3, 3 ),
 ( 0.0002011154675331821196, 0.0003574932873931827796 ),
 ( 0.000000000000000000, 1.000000000000000000 ),
 .UNSPECIFIED. ) 
 GEOMETRIC_REPRESENTATION_ITEM ( )  RATIONAL_B_SPLINE_SURFACE ( (
 ( 1.000000000000000000, 0.7460133799027759416, 1.000000000000000000),
 ( 1.000000000000000000, 0.7464018141889758873, 1.000000000000000000),
 ( 1.000000000000000000, 0.7343312752103077212, 1.000000000000000000),
 ( 1.000000000000000000, 0.7219065546282223966, 1.000000000000000000) ) ) 
 REPRESENTATION_ITEM ( '' )  SURFACE ( )  );
#6973=CARTESIAN_POINT ( 'NONE',  ( -40.68422973805265030, 6.807290781432339344, 39.54930799450052348 ) ) ;
#6990=DIRECTION ( 'NONE',  ( -0.2756373558169954441, 0.9612616959383198934, -1.479773560108263204E-16 ) ) ;
#6991=ORIENTED_EDGE ( 'NONE', *, *, #27507, .F. ) ;
#6992=AXIS2_PLACEMENT_3D ( 'NONE', #1865, #16470, #31585 ) ;
#6993=VECTOR ( 'NONE', #29025, 1000.000000000000000 ) ;
#6995=ORIENTED_EDGE ( 'NONE', *, *, #15437, .T. ) ;
#6997=VERTEX_POINT ( 'NONE', #8763 ) ;
#7003=EDGE_LOOP ( 'NONE', ( #16498, #23640, #17082, #9718 ) ) ;
#7011=EDGE_CURVE ( 'NONE', #32358, #10736, #27293, .T. ) ;
#7014=ORIENTED_EDGE ( 'NONE', *, *, #11648, .F. ) ;
#7016=ORIENTED_EDGE ( 'NONE', *, *, #15204, .F. ) ;
#7018=CARTESIAN_POINT ( 'NONE',  ( -40.70335362822509495, 9.387769322903325886, 39.54930799450052348 ) ) ;
#7024=LINE ( 'NONE', #17020, #6993 ) ;
#7025=EDGE_LOOP ( 'NONE', ( #13740, #31535, #6949, #5275 ) ) ;
#7030=LINE ( 'NONE', #17032, #28777 ) ;
#7032=AXIS2_PLACEMENT_3D ( 'NONE', #12316, #12153, #2296 ) ;
#7043=FACE_OUTER_BOUND ( 'NONE', #8677, .T. ) ;
#7045=AXIS2_PLACEMENT_3D ( 'NONE', #6603, #1346, #28931 ) ;
#7053=TOROIDAL_SURFACE ( 'NONE', #12834, 0.2000000000000000111, 0.1000000000000000056 ) ;
#7068=VERTEX_POINT ( 'NONE', #32241 ) ;
#7071=ADVANCED_FACE ( 'NONE', ( #4989 ), #22533, .T. ) ;
#7073=DIRECTION ( 'NONE',  ( -0.6797146636928675933, -0.1949050434465284254, 0.7071067811865466846 ) ) ;
#7079=VECTOR ( 'NONE', #30277, 1000.000000000000114 ) ;
#7082=ORIENTED_EDGE ( 'NONE', *, *, #22974, .F. ) ;
#7084=CARTESIAN_POINT ( 'NONE',  ( -41.52218637998915085, 11.15499190493234671, 37.04930799450052348 ) ) ;
#7087=EDGE_LOOP ( 'NONE', ( #32060, #1150 ) ) ;
#7089=DIRECTION ( 'NONE',  ( 0.000000000000000000, -4.336808689941893885E-15, -1.000000000000000000 ) ) ;
#7094=PLANE ( 'NONE',  #1581 ) ;
#7107=ORIENTED_EDGE ( 'NONE', *, *, #3600, .T. ) ;
#7110=CARTESIAN_POINT ( 'NONE',  ( -43.37834615508418068, 1.121909970995877526, 39.54930799450052348 ) ) ;
#7112=VERTEX_POINT ( 'NONE', #19740 ) ;
#7113=CARTESIAN_POINT ( 'NONE',  ( -40.17244512953781310, 6.931285263614340941, 39.54930799450052348 ) ) ;
#7118=CARTESIAN_POINT ( 'NONE',  ( -42.37913764077812573, 15.23192269303852697, 38.44930799450052916 ) ) ;
#7131=DIRECTION ( 'NONE',  ( 0.2756373558169974425, -0.9612616959383193382, 0.000000000000000000 ) ) ;
#7135=CYLINDRICAL_SURFACE ( 'NONE', #13397, 0.1000000000000018235 ) ;
#7138=CARTESIAN_POINT ( 'NONE',  ( -41.88090303775678080, 13.82677487427665497, 59.44930799450051495 ) ) ;
#7144=CYLINDRICAL_SURFACE ( 'NONE', #28428, 2.000000000000001776 ) ;
#7145=DIRECTION ( 'NONE',  ( -0.8746197071393926326, 0.4848096202463430537, 8.676864087101709653E-18 ) ) ;
#7146=DIRECTION ( 'NONE',  ( -0.2756373558170082672, 0.9612616959383162296, 0.000000000000000000 ) ) ;
#7165=ORIENTED_EDGE ( 'NONE', *, *, #3477, .F. ) ;
#7168=DIRECTION ( 'NONE',  ( -2.779292025043186357E-18, 1.288349127009862211E-17, -1.000000000000000000 ) ) ;
#7171=VERTEX_POINT ( 'NONE', #5316 ) ;
#7175=CARTESIAN_POINT ( 'NONE',  ( -40.57832940339291383, 7.446916344587776848, 60.44930799450051495 ) ) ;
#7178=CARTESIAN_POINT ( 'NONE',  ( -40.23971823762673239, 6.784144620117122493, 53.64930799450051779 ) ) ;
#7192=EDGE_CURVE ( 'NONE', #24444, #32232, #26255, .T. ) ;
#7197=CARTESIAN_POINT ( 'NONE',  ( -42.36691375901575185, 13.72999064396537250, 54.61480954800870791 ) ) ;
#7203=EDGE_LOOP ( 'NONE', ( #21805, #31449, #23804, #17681 ) ) ;
#7209=DIRECTION ( 'NONE',  ( -0.4848096202463431648, -0.8746197071393924105, 0.000000000000000000 ) ) ;
#7212=ORIENTED_EDGE ( 'NONE', *, *, #11607, .F. ) ;
#7213=VECTOR ( 'NONE', #18709, 1000.000000000000114 ) ;
#7223=DIRECTION ( 'NONE',  ( -0.4848096202463429427, -0.8746197071393925215, 2.352477780477436294E-16 ) ) ;
#7231=ADVANCED_FACE ( 'NONE', ( #29710 ), #24448, .F. ) ;
#7234=CARTESIAN_POINT ( 'NONE',  ( -42.03703168893574116, 3.954238390689463145, 47.04930799450051637 ) ) ;
#7241=DIRECTION ( 'NONE',  ( 0.9915148059396263758, 0.1299938060159218089, -1.080935127887223745E-18 ) ) ;
#7244=CIRCLE ( 'NONE', #29235, 0.9999999999999998890 ) ;
#7246=CIRCLE ( 'NONE', #18242, 1.100000000000000311 ) ;
#7247=AXIS2_PLACEMENT_3D ( 'NONE', #18676, #26724, #4401 ) ;
#7251=CARTESIAN_POINT ( 'NONE',  ( -41.96544240928614755, 13.75880317176705603, 59.54930799450050927 ) ) ;
#7254=CARTESIAN_POINT ( 'NONE',  ( -40.45390504179176361, 8.517838719579989615, 39.46050754198200394 ) ) ;
#7257=DIRECTION ( 'NONE',  ( 0.9612616959383205595, 0.2756373558169930571, -1.660411357259282199E-16 ) ) ;
#7258=EDGE_CURVE ( 'NONE', #14586, #23429, #17220, .T. ) ;
#7261=CARTESIAN_POINT ( 'NONE',  ( -40.50745992490246294, 7.570570027725508133, 60.23867152839895311 ) ) ;
#7263=CYLINDRICAL_SURFACE ( 'NONE', #5797, 1.624998423334082620 ) ;
#7265=DIRECTION ( 'NONE',  ( 0.1138751963119829791, -0.8685717160922530322, -0.4823024089401439785 ) ) ;
#7273=CARTESIAN_POINT ( 'NONE',  ( -40.14234630318158281, 6.912323292265332597, 34.55513836777664238 ) ) ;
#7284=CYLINDRICAL_SURFACE ( 'NONE', #24662, 2.000000000000001776 ) ;
#7289=EDGE_LOOP ( 'NONE', ( #17602, #32411, #5861, #15706 ) ) ;
#7298=VECTOR ( 'NONE', #4247, 1000.000000000000000 ) ;
#7299=CARTESIAN_POINT ( 'NONE',  ( -40.85838585144898616, 8.484324852566594188, 34.62702073480610210 ) ) ;
#7315=DIRECTION ( 'NONE',  ( -0.2756373558169900040, 0.9612616959383215587, 0.000000000000000000 ) ) ;
#7320=CARTESIAN_POINT ( 'NONE',  ( -38.36853489569023168, 7.065850718397949315, 32.04930799450052348 ) ) ;
#7325=ORIENTED_EDGE ( 'NONE', *, *, #9139, .T. ) ;
#7327=CIRCLE ( 'NONE', #24609, 1.199999999999999734 ) ;
#7330=AXIS2_PLACEMENT_3D ( 'NONE', #3331, #20886, #31238 ) ;
#7336=CARTESIAN_POINT ( 'NONE',  ( -41.08785830660042393, 9.277514380576530328, 38.60788663826321709 ) ) ;
#7347=LINE ( 'NONE', #4553, #16764 ) ;
#7348=DIRECTION ( 'NONE',  ( -0.4848096202463424431, -0.8746197071393927436, 2.220446049250312588E-16 ) ) ;
#7349=PLANE ( 'NONE',  #27419 ) ;
#7355=LINE ( 'NONE', #30329, #10664 ) ;
#7358=VERTEX_POINT ( 'NONE', #12010 ) ;
#7359=AXIS2_PLACEMENT_3D ( 'NONE', #13931, #28863, #6374 ) ;
#7365=DIRECTION ( 'NONE',  ( 0.2756373558170082672, -0.9612616959383162296, 0.000000000000000000 ) ) ;
#7366=ORIENTED_EDGE ( 'NONE', *, *, #28288, .T. ) ;
#7367=( BOUNDED_SURFACE ( )  B_SPLINE_SURFACE ( 3, 2, ( 
 ( #22814, #10349, #26410 ),
 ( #25921, #23465, #10843 ),
 ( #30703, #975, #20834 ),
 ( #3436, #5913, #13466 ) ),
 .UNSPECIFIED., .F., .F., .F. ) 
 B_SPLINE_SURFACE_WITH_KNOTS ( ( 4, 4 ),
 ( 3, 3 ),
 ( 0.0002661489594880761360, 0.0004225458590890279168 ),
 ( 0.000000000000000000, 1.000000000000000000 ),
 .UNSPECIFIED. ) 
 GEOMETRIC_REPRESENTATION_ITEM ( )  RATIONAL_B_SPLINE_SURFACE ( (
 ( 1.000000000000000000, 0.7219065546282040780, 1.000000000000000000),
 ( 1.000000000000000000, 0.7343063454201389506, 1.000000000000000000),
 ( 1.000000000000000000, 0.7464000351581004944, 1.000000000000000000),
 ( 1.000000000000000000, 0.7460133799027759416, 1.000000000000000000) ) ) 
 REPRESENTATION_ITEM ( '' )  SURFACE ( )  );
#7386=CARTESIAN_POINT ( 'NONE',  ( -40.47970302497626705, 7.463434137431151250, 60.44930799450051495 ) ) ;
#7394=LINE ( 'NONE', #17388, #17043 ) ;
#7401=LINE ( 'NONE', #10342, #19173 ) ;
#7402=DIRECTION ( 'NONE',  ( 0.8746197071393926326, -0.4848096202463430537, -8.676864087101709653E-18 ) ) ;
#7413=DIRECTION ( 'NONE',  ( -0.1949050434465282589, 0.6797146636928674823, 0.7071067811865470176 ) ) ;
#7414=EDGE_CURVE ( 'NONE', #7845, #21311, #19872, .T. ) ;
#7417=ORIENTED_EDGE ( 'NONE', *, *, #25528, .F. ) ;
#7421=EDGE_CURVE ( 'NONE', #8855, #28053, #32199, .T. ) ;
#7423=AXIS2_PLACEMENT_3D ( 'NONE', #19931, #19765, #29963 ) ;
#7425=FACE_OUTER_BOUND ( 'NONE', #7003, .T. ) ;
#7426=CARTESIAN_POINT ( 'NONE',  ( -42.37913764077812573, 15.23192269303852875, 35.64930799450052490 ) ) ;
#7434=DIRECTION ( 'NONE',  ( 0.2756373558169945559, -0.9612616959383202264, 0.000000000000000000 ) ) ;
#7447=DIRECTION ( 'NONE',  ( 0.2756373558169974980, -0.9612616959383193382, -1.315048337272770589E-17 ) ) ;
#7450=DIRECTION ( 'NONE',  ( -0.4848096202463424431, -0.8746197071393927436, 2.220446049250312588E-16 ) ) ;
#7452=DIRECTION ( 'NONE',  ( -2.779292025043186357E-18, 1.288349127009862211E-17, -1.000000000000000000 ) ) ;
#7453=LINE ( 'NONE', #4987, #25878 ) ;
#7465=AXIS2_PLACEMENT_3D ( 'NONE', #19883, #15135, #9882 ) ;
#7466=DIRECTION ( 'NONE',  ( -0.9612616959383200044, -0.2756373558169954996, 1.660411357259285896E-16 ) ) ;
#7467=DIRECTION ( 'NONE',  ( -2.472450503250596893E-15, -7.226442137580869828E-16, 1.000000000000000000 ) ) ;
#7470=CARTESIAN_POINT ( 'NONE',  ( -40.86542064515101202, 8.501822640387086238, 34.64781247685129273 ) ) ;
#7471=ORIENTED_EDGE ( 'NONE', *, *, #15012, .T. ) ;
#7473=CARTESIAN_POINT ( 'NONE',  ( -41.91739890389096956, 13.90674392281398930, 59.49868301348410426 ) ) ;
#7484=DIRECTION ( 'NONE',  ( 0.2530443915477140204, -0.8824706660164525207, 0.3965022818682459316 ) ) ;
#7485=ORIENTED_EDGE ( 'NONE', *, *, #7192, .F. ) ;
#7499=DIRECTION ( 'NONE',  ( -2.779292025043186357E-18, 1.288349127009862211E-17, -1.000000000000000000 ) ) ;
#7515=DIRECTION ( 'NONE',  ( -0.9612616959383206705, -0.2756373558169931681, 1.660411357259282445E-16 ) ) ;
#7518=CARTESIAN_POINT ( 'NONE',  ( -40.11286833322907341, 2.887657226147505973, 38.24930799450051921 ) ) ;
#7524=ORIENTED_EDGE ( 'NONE', *, *, #5815, .F. ) ;
#7528=DIRECTION ( 'NONE',  ( -0.9612616959383183390, -0.2756373558170014948, -8.795445018805493151E-19 ) ) ;
#7532=EDGE_LOOP ( 'NONE', ( #5620, #17803, #6252, #17625 ) ) ;
#7539=EDGE_CURVE ( 'NONE', #4111, #2645, #19750, .T. ) ;
#7540=AXIS2_PLACEMENT_3D ( 'NONE', #27539, #5385, #24917 ) ;
#7550=ORIENTED_EDGE ( 'NONE', *, *, #550, .T. ) ;
#7551=VERTEX_POINT ( 'NONE', #2805 ) ;
#7556=CARTESIAN_POINT ( 'NONE',  ( -38.34904439134557919, 6.997879252028663011, 61.94930799450052206 ) ) ;
#7558=ORIENTED_EDGE ( 'NONE', *, *, #19334, .F. ) ;
#7559=ORIENTED_EDGE ( 'NONE', *, *, #29391, .F. ) ;
#7570=CARTESIAN_POINT ( 'NONE',  ( -39.67555847965937943, 2.645252416024337361, 48.94930799450051495 ) ) ;
#7574=VERTEX_POINT ( 'NONE', #15440 ) ;
#7579=CIRCLE ( 'NONE', #27495, 0.1000000000000004774 ) ;
#7585=DIRECTION ( 'NONE',  ( -0.2530443915477366690, 0.8824706660164322036, 0.3965022818682769623 ) ) ;
#7589=DIRECTION ( 'NONE',  ( 0.4151817967359235362, -0.9097384655268405673, 0.000000000000000000 ) ) ;
#7590=DIRECTION ( 'NONE',  ( -0.3879443550132459229, -0.6998701428318346851, 0.5997340748914504749 ) ) ;
#7595=VERTEX_POINT ( 'NONE', #12991 ) ;
#7602=ORIENTED_EDGE ( 'NONE', *, *, #26202, .F. ) ;
#7603=CARTESIAN_POINT ( 'NONE',  ( -43.64073206722599707, 1.267352857069778960, 34.54930799450052348 ) ) ;
#7605=DIRECTION ( 'NONE',  ( -0.8746197071393955191, 0.4848096202463378357, 8.676864087101651105E-18 ) ) ;
#7609=AXIS2_PLACEMENT_3D ( 'NONE', #2492, #17257, #10055 ) ;
#7615=CARTESIAN_POINT ( 'NONE',  ( -42.22138300640813924, 14.68176690255378603, 36.00717268343339583 ) ) ;
#7617=AXIS2_PLACEMENT_3D ( 'NONE', #25928, #15923, #28243 ) ;
#7620=ADVANCED_FACE ( 'NONE', ( #8222 ), #16037, .T. ) ;
#7621=CARTESIAN_POINT ( 'NONE',  ( -40.65120636623950645, 8.087130829066872195, 57.04930799450051637 ) ) ;
#7627=AXIS2_PLACEMENT_3D ( 'NONE', #14212, #22227, #12236 ) ;
#7629=ORIENTED_EDGE ( 'NONE', *, *, #30104, .F. ) ;
#7635=ADVANCED_FACE ( 'NONE', ( #1630 ), #31349, .T. ) ;
#7636=CARTESIAN_POINT ( 'NONE',  ( -40.11286833322907341, 2.887657226147507306, 38.34930799450052064 ) ) ;
#7643=CARTESIAN_POINT ( 'NONE',  ( -40.82323252358241206, 8.354654602666819585, 40.36793714460204541 ) ) ;
#7644=LINE ( 'NONE', #14538, #17346 ) ;
#7647=DIRECTION ( 'NONE',  ( -0.9612616959383194493, -0.2756373558169972759, -8.795445018804907668E-19 ) ) ;
#7653=ADVANCED_FACE ( 'NONE', ( #28565 ), #16240, .T. ) ;
#7654=ORIENTED_EDGE ( 'NONE', *, *, #16232, .T. ) ;
#7656=ORIENTED_EDGE ( 'NONE', *, *, #3963, .T. ) ;
#7660=DIRECTION ( 'NONE',  ( 0.000000000000000000, 0.000000000000000000, -1.000000000000000000 ) ) ;
#7663=EDGE_LOOP ( 'NONE', ( #8070, #6157, #1720, #23909 ) ) ;
#7666=CARTESIAN_POINT ( 'NONE',  ( -40.22018024869838371, 7.672350704644241404, 60.22001867261916885 ) ) ;
#7674=CIRCLE ( 'NONE', #18654, 0.1000000000000006301 ) ;
#7678=LINE ( 'NONE', #13092, #4289 ) ;
#7692=ORIENTED_EDGE ( 'NONE', *, *, #11761, .F. ) ;
#7694=CARTESIAN_POINT ( 'NONE',  ( -40.11286833322907341, 2.887657226147507306, 35.14930799450051779 ) ) ;
#7701=LINE ( 'NONE', #20317, #20372 ) ;
#7703=DIRECTION ( 'NONE',  ( 0.000000000000000000, 0.000000000000000000, -1.000000000000000000 ) ) ;
#7708=ORIENTED_EDGE ( 'NONE', *, *, #8413, .T. ) ;
#7711=CARTESIAN_POINT ( 'NONE',  ( -40.69230700880733309, 6.792718999258627655, 34.69881571428543765 ) ) ;
#7715=ORIENTED_EDGE ( 'NONE', *, *, #7258, .F. ) ;
#7721=EDGE_CURVE ( 'NONE', #30017, #16381, #4493, .T. ) ;
#7724=ORIENTED_EDGE ( 'NONE', *, *, #23018, .F. ) ;
#7729=FACE_OUTER_BOUND ( 'NONE', #17064, .T. ) ;
#7730=ORIENTED_EDGE ( 'NONE', *, *, #24983, .F. ) ;
#7733=ORIENTED_EDGE ( 'NONE', *, *, #1016, .T. ) ;
#7746=PLANE ( 'NONE',  #31704 ) ;
#7747=DIRECTION ( 'NONE',  ( 0.2756373558169974980, -0.9612616959383193382, 9.694974607321218218E-33 ) ) ;
#7748=DIRECTION ( 'NONE',  ( 0.6797146636928694807, 0.1949050434465297021, 0.7071067811865444641 ) ) ;
#7759=EDGE_CURVE ( 'NONE', #14556, #18455, #1142, .T. ) ;
#7761=ORIENTED_EDGE ( 'NONE', *, *, #1138, .F. ) ;
#7764=CARTESIAN_POINT ( 'NONE',  ( -43.90780810587784089, -0.03953120679776488122, 61.94930799450052206 ) ) ;
#7786=ORIENTED_EDGE ( 'NONE', *, *, #16965, .T. ) ;
#7787=CARTESIAN_POINT ( 'NONE',  ( -39.59300248568538194, 7.744584186742829779, 32.14930799450051779 ) ) ;
#7788=ORIENTED_EDGE ( 'NONE', *, *, #4826, .T. ) ;
#7812=AXIS2_PLACEMENT_3D ( 'NONE', #28158, #895, #30780 ) ;
#7813=ORIENTED_EDGE ( 'NONE', *, *, #25850, .T. ) ;
#7814=CONICAL_SURFACE ( 'NONE', #10413, 1.003191532947550701, 0.7853981633974447263 ) ;
#7815=EDGE_CURVE ( 'NONE', #20995, #13496, #14596, .T. ) ;
#7823=ORIENTED_EDGE ( 'NONE', *, *, #29046, .F. ) ;
#7839=DIRECTION ( 'NONE',  ( 0.4848096202463636484, 0.8746197071393810862, 0.000000000000000000 ) ) ;
#7842=( BOUNDED_CURVE ( )  B_SPLINE_CURVE ( 3, ( #27120, #14658, #26473, #21860 ),
 .UNSPECIFIED., .F., .F. ) 
 B_SPLINE_CURVE_WITH_KNOTS ( ( 4, 4 ),
 ( 4.712388980384679016, 4.772243325917784773 ),
 .UNSPECIFIED. ) 
 CURVE ( )  GEOMETRIC_REPRESENTATION_ITEM ( )  RATIONAL_B_SPLINE_CURVE ( ( 1.000000000000000000, 0.9997014770583808607, 0.9997014770583808607, 1.000000000000000000 ) ) 
 REPRESENTATION_ITEM ( '' )  );
#7843=DIRECTION ( 'NONE',  ( -0.4848096202463371696, -0.8746197071393958522, 0.000000000000000000 ) ) ;
#7845=VERTEX_POINT ( 'NONE', #27220 ) ;
#7846=EDGE_CURVE ( 'NONE', #6409, #23264, #3448, .T. ) ;
#7850=PLANE ( 'NONE',  #2213 ) ;
#7853=ORIENTED_EDGE ( 'NONE', *, *, #20924, .T. ) ;
#7854=FACE_OUTER_BOUND ( 'NONE', #6092, .T. ) ;
#7855=ORIENTED_EDGE ( 'NONE', *, *, #31795, .T. ) ;
#7873=VECTOR ( 'NONE', #250, 1000.000000000000227 ) ;
#7874=VERTEX_POINT ( 'NONE', #13076 ) ;
#7877=ORIENTED_EDGE ( 'NONE', *, *, #407, .F. ) ;
#7878=CARTESIAN_POINT ( 'NONE',  ( -43.73393778030726509, 1.305471833569777695, 53.64930799450051779 ) ) ;
#7880=LINE ( 'NONE', #2620, #12748 ) ;
#7881=LINE ( 'NONE', #20332, #29397 ) ;
#7896=VECTOR ( 'NONE', #17711, 1000.000000000000114 ) ;
#7897=AXIS2_PLACEMENT_3D ( 'NONE', #6600, #28597, #6437 ) ;
#7907=ADVANCED_FACE ( 'NONE', ( #5676 ), #11245, .T. ) ;
#7908=ADVANCED_FACE ( 'NONE', ( #13243 ), #28639, .F. ) ;
#7909=LINE ( 'NONE', #30557, #27702 ) ;
#7910=CARTESIAN_POINT ( 'NONE',  ( -40.65487266620045403, 9.475231293617264683, 39.43717596014455040 ) ) ;
#7913=AXIS2_PLACEMENT_3D ( 'NONE', #26027, #6497, #1236 ) ;
#7914=CARTESIAN_POINT ( 'NONE',  ( -41.96544240928614755, 13.75880317176705603, 59.54930799450050927 ) ) ;
#7915=DIRECTION ( 'NONE',  ( -2.779292025043186357E-18, 1.288349127009862211E-17, -1.000000000000000000 ) ) ;
#7920=DIRECTION ( 'NONE',  ( 0.4848096202463430537, 0.8746197071393926326, -1.125439520643636483E-16 ) ) ;
#7922=CIRCLE ( 'NONE', #11594, 1.500000000000001332 ) ;
#7926=AXIS2_PLACEMENT_3D ( 'NONE', #17140, #9611, #7146 ) ;
#7930=ORIENTED_EDGE ( 'NONE', *, *, #15431, .T. ) ;
#7933=DIRECTION ( 'NONE',  ( 0.8746197071393926326, -0.4848096202463430537, -8.676864087101709653E-18 ) ) ;
#7934=ORIENTED_EDGE ( 'NONE', *, *, #30543, .F. ) ;
#7935=ORIENTED_EDGE ( 'NONE', *, *, #27267, .T. ) ;
#7947=EDGE_CURVE ( 'NONE', #2831, #3387, #22312, .T. ) ;
#7953=DIRECTION ( 'NONE',  ( 1.188208965918165239E-16, 1.880121038077813132E-16, 1.000000000000000000 ) ) ;
#7956=ORIENTED_EDGE ( 'NONE', *, *, #16284, .T. ) ;
#7961=CARTESIAN_POINT ( 'NONE',  ( -40.69349378885117119, 6.789343923716915974, 39.46053429011656988 ) ) ;
#7965=CARTESIAN_POINT ( 'NONE',  ( -41.23380787120766655, 11.23768311167744294, 37.04930799450052348 ) ) ;
#7971=DIRECTION ( 'NONE',  ( -0.2756373558169932236, 0.9612616959383205595, 2.536267806945839542E-31 ) ) ;
#7978=VERTEX_POINT ( 'NONE', #586 ) ;
#7979=DIRECTION ( 'NONE',  ( -0.2756373558169938898, 0.9612616959383203374, 0.000000000000000000 ) ) ;
#7988=CARTESIAN_POINT ( 'NONE',  ( -40.59581018552366061, 9.375516295340281303, 34.64930799450051779 ) ) ;
#7991=ORIENTED_EDGE ( 'NONE', *, *, #15495, .T. ) ;
#7993=DIRECTION ( 'NONE',  ( 0.7141240004913222972, -0.3958453973320028019, -0.5773502691896303940 ) ) ;
#7994=CARTESIAN_POINT ( 'NONE',  ( -40.08841711228579641, 7.575633567407562552, 60.54930799450051637 ) ) ;
#7995=DIRECTION ( 'NONE',  ( 0.8718554444429661432, -0.4832773644130859969, 0.07944226231105885883 ) ) ;
#7996=ORIENTED_EDGE ( 'NONE', *, *, #30719, .F. ) ;
#8004=CARTESIAN_POINT ( 'NONE',  ( -42.39006672483308336, 15.27003693862973854, 38.54111136810265492 ) ) ;
#8012=EDGE_LOOP ( 'NONE', ( #22770, #5356, #27666, #7485, #21329 ) ) ;
#8015=ADVANCED_FACE ( 'NONE', ( #1067 ), #4343, .F. ) ;
#8023=EDGE_CURVE ( 'NONE', #27032, #13059, #28724, .T. ) ;
#8034=( BOUNDED_CURVE ( )  B_SPLINE_CURVE ( 3, ( #7473, #27323, #10262, #22222 ),
 .UNSPECIFIED., .F., .F. ) 
 B_SPLINE_CURVE_WITH_KNOTS ( ( 4, 4 ),
 ( 5.766788280868928140, 6.283185307179586232 ),
 .UNSPECIFIED. ) 
 CURVE ( )  GEOMETRIC_REPRESENTATION_ITEM ( )  RATIONAL_B_SPLINE_CURVE ( ( 1.000000000000000000, 0.9779010246516586236, 0.9779010246516586236, 1.000000000000000000 ) ) 
 REPRESENTATION_ITEM ( '' )  );
#8037=CARTESIAN_POINT ( 'NONE',  ( -42.92070284191122909, 15.66940288633442790, 37.04930799450052348 ) ) ;
#8046=LINE ( 'NONE', #4927, #30977 ) ;
#8047=DIRECTION ( 'NONE',  ( -0.9612616959383206705, -0.2756373558169931681, 1.660411357259282445E-16 ) ) ;
#8048=ADVANCED_FACE ( 'NONE', ( #21724 ), #9765, .T. ) ;
#8053=CARTESIAN_POINT ( 'NONE',  ( -41.52218637998914375, 11.15499190493234849, 35.90717268343339441 ) ) ;
#8055=DIRECTION ( 'NONE',  ( -2.946248497964555786E-19, -3.001156285468303092E-19, -1.000000000000000000 ) ) ;
#8057=ORIENTED_EDGE ( 'NONE', *, *, #1626, .F. ) ;
#8058=FACE_OUTER_BOUND ( 'NONE', #20804, .T. ) ;
#8059=CARTESIAN_POINT ( 'NONE',  ( -40.50726676055796105, 7.559560307024983494, 53.80788663826320573 ) ) ;
#8061=CARTESIAN_POINT ( 'NONE',  ( -40.90015969217747482, 8.955334253785164123, 56.14611646155296398 ) ) ;
#8068=CARTESIAN_POINT ( 'NONE',  ( -41.13156850465621517, 9.429949956619452678, 38.44930799450052916 ) ) ;
#8070=ORIENTED_EDGE ( 'NONE', *, *, #27616, .T. ) ;
#8075=CARTESIAN_POINT ( 'NONE',  ( -40.59689739711614465, 7.533859135569301202, 53.64930799450051779 ) ) ;
#8077=DIRECTION ( 'NONE',  ( 0.9612616959383205595, 0.2756373558169931681, -1.660411357259282445E-16 ) ) ;
#8082=CARTESIAN_POINT ( 'NONE',  ( -40.11286833322907341, 2.887657226147507306, 38.94930799450052206 ) ) ;
#8096=LINE ( 'NONE', #12863, #11042 ) ;
#8098=DIRECTION ( 'NONE',  ( -0.4848096202463645921, -0.8746197071393805311, 0.000000000000000000 ) ) ;
#8104=DIRECTION ( 'NONE',  ( 0.8746197071393925215, -0.4848096202463429982, -8.676864087101708112E-18 ) ) ;
#8111=CARTESIAN_POINT ( 'NONE',  ( -41.94956971822180947, 3.905757428664828890, 47.04930799450051637 ) ) ;
#8113=CARTESIAN_POINT ( 'NONE',  ( -43.38408989745150990, 1.111547985471240008, 53.64930799450051779 ) ) ;
#8116=FACE_OUTER_BOUND ( 'NONE', #20740, .T. ) ;
#8119=CYLINDRICAL_SURFACE ( 'NONE', #4292, 0.1000000000000007272 ) ;
#8128=CARTESIAN_POINT ( 'NONE',  ( -40.54770213959439218, 7.393765961829922517, 38.67976136800678688 ) ) ;
#8129=DIRECTION ( 'NONE',  ( -0.2756373558169932236, 0.9612616959383204485, -1.479773560108267395E-16 ) ) ;
#8132=DIRECTION ( 'NONE',  ( 0.4848096202463317295, 0.8746197071393987388, 0.000000000000000000 ) ) ;
#8134=EDGE_CURVE ( 'NONE', #19940, #23798, #23872, .T. ) ;
#8139=EDGE_CURVE ( 'NONE', #22591, #6106, #11731, .T. ) ;
#8140=CARTESIAN_POINT ( 'NONE',  ( -38.36853489569023168, 7.065850718397949315, 32.14930799450051779 ) ) ;
#8149=ORIENTED_EDGE ( 'NONE', *, *, #28320, .F. ) ;
#8159=SPHERICAL_SURFACE ( 'NONE', #12837, 0.1000000000000000056 ) ;
#8161=ORIENTED_EDGE ( 'NONE', *, *, #19565, .F. ) ;
#8169=EDGE_LOOP ( 'NONE', ( #19802, #6687, #4968, #28670 ) ) ;
#8170=CARTESIAN_POINT ( 'NONE',  ( -40.57832940339291383, 7.446916344587776848, 53.64930799450051779 ) ) ;
#8171=ORIENTED_EDGE ( 'NONE', *, *, #18599, .F. ) ;
#8172=AXIS2_PLACEMENT_3D ( 'NONE', #6286, #1354, #5977 ) ;
#8176=ADVANCED_FACE ( 'NONE', ( #68 ), #22215, .F. ) ;
#8188=ORIENTED_EDGE ( 'NONE', *, *, #11756, .F. ) ;
#8189=CARTESIAN_POINT ( 'NONE',  ( -43.90780810587784089, -0.03953120679776488122, 61.94930799450052206 ) ) ;
#8193=EDGE_CURVE ( 'NONE', #2479, #29694, #12722, .T. ) ;
#8202=LINE ( 'NONE', #10506, #168 ) ;
#8204=CYLINDRICAL_SURFACE ( 'NONE', #18435, 0.1000000000000006301 ) ;
#8220=EDGE_CURVE ( 'NONE', #14804, #28351, #8702, .T. ) ;
#8222=FACE_OUTER_BOUND ( 'NONE', #13117, .T. ) ;
#8224=EDGE_CURVE ( 'NONE', #14081, #4732, #2692, .T. ) ;
#8227=DIRECTION ( 'NONE',  ( 2.946248497964555786E-19, 3.001156285468303092E-19, 1.000000000000000000 ) ) ;
#8228=DIRECTION ( 'NONE',  ( 0.8746197071393925215, -0.4848096202463429982, -8.676864087101708112E-18 ) ) ;
#8234=EDGE_CURVE ( 'NONE', #10451, #30053, #19705, .T. ) ;
#8236=CARTESIAN_POINT ( 'NONE',  ( -43.90780810587784089, -0.03953120679776488122, 62.04930799450052348 ) ) ;
#8238=CARTESIAN_POINT ( 'NONE',  ( -40.60251150970604073, 6.748447833883065350, 53.54930799450051637 ) ) ;
#8242=CARTESIAN_POINT ( 'NONE',  ( -43.95628906790246759, -0.1269931775117038586, 32.14930799450051779 ) ) ;
#8248=CARTESIAN_POINT ( 'NONE',  ( -40.11036131418491379, 6.815955993705610894, 39.36132530173779287 ) ) ;
#8255=CIRCLE ( 'NONE', #19786, 2.000000000000001776 ) ;
#8261=ADVANCED_FACE ( 'NONE', ( #27479 ), #29158, .T. ) ;
#8262=EDGE_LOOP ( 'NONE', ( #10849, #4103, #17155, #22691, #17438, #10528, #4192 ) ) ;
#8265=CARTESIAN_POINT ( 'NONE',  ( -43.37834615508418068, 1.121909970995875971, 34.64930799450052490 ) ) ;
#8280=VERTEX_POINT ( 'NONE', #30112 ) ;
#8286=CARTESIAN_POINT ( 'NONE',  ( -39.85048242108726413, 2.742214340073605428, 48.54930799450051637 ) ) ;
#8287=AXIS2_PLACEMENT_3D ( 'NONE', #2693, #2845, #22714 ) ;
#8307=DIRECTION ( 'NONE',  ( 7.588956326749211550E-18, -4.206627182996912454E-18, 1.000000000000000000 ) ) ;
#8318=DIRECTION ( 'NONE',  ( -0.4848096202463636484, -0.8746197071393810862, 0.000000000000000000 ) ) ;
#8322=DIRECTION ( 'NONE',  ( 0.8746197071393960742, -0.4848096202463368365, -1.277302113040972115E-17 ) ) ;
#8323=FACE_OUTER_BOUND ( 'NONE', #8012, .T. ) ;
#8324=ORIENTED_EDGE ( 'NONE', *, *, #17254, .F. ) ;
#8329=AXIS2_PLACEMENT_3D ( 'NONE', #32185, #31694, #27083 ) ;
#8332=ORIENTED_EDGE ( 'NONE', *, *, #24151, .T. ) ;
#8342=ADVANCED_FACE ( 'NONE', ( #13360 ), #30120, .T. ) ;
#8348=ORIENTED_EDGE ( 'NONE', *, *, #5537, .T. ) ;
#8349=VERTEX_POINT ( 'NONE', #11056 ) ;
#8351=ORIENTED_EDGE ( 'NONE', *, *, #22484, .T. ) ;
#8352=CIRCLE ( 'NONE', #24585, 0.1000000000000018235 ) ;
#8354=DIRECTION ( 'NONE',  ( 1.188208965918165239E-16, 1.880121038077813132E-16, 1.000000000000000000 ) ) ;
#8364=VERTEX_POINT ( 'NONE', #30433 ) ;
#8371=EDGE_CURVE ( 'NONE', #1586, #19917, #4947, .T. ) ;
#8375=AXIS2_PLACEMENT_3D ( 'NONE', #32153, #9664, #17194 ) ;
#8376=ORIENTED_EDGE ( 'NONE', *, *, #1110, .F. ) ;
#8381=ORIENTED_EDGE ( 'NONE', *, *, #27873, .T. ) ;
#8383=CARTESIAN_POINT ( 'NONE',  ( -40.13606231985500017, 7.635531802539802015, 60.44930799450051495 ) ) ;
#8385=EDGE_CURVE ( 'NONE', #13254, #5658, #17945, .T. ) ;
#8387=DIRECTION ( 'NONE',  ( -0.9612616959383205595, -0.2756373558169931681, 1.660411357259282445E-16 ) ) ;
#8392=DIRECTION ( 'NONE',  ( 0.1949050434465251225, -0.6797146636928670382, 0.7071067811865481278 ) ) ;
#8395=LINE ( 'NONE', #8238, #9474 ) ;
#8397=ORIENTED_EDGE ( 'NONE', *, *, #23276, .T. ) ;
#8398=DIRECTION ( 'NONE',  ( 0.7141240004913198547, -0.3958453973320100738, 0.5773502691896283956 ) ) ;
#8405=CIRCLE ( 'NONE', #26738, 0.1000000000000004774 ) ;
#8407=EDGE_CURVE ( 'NONE', #16381, #8613, #15486, .T. ) ;
#8408=ORIENTED_EDGE ( 'NONE', *, *, #13860, .T. ) ;
#8409=CARTESIAN_POINT ( 'NONE',  ( -40.51002469154155250, 7.586466571548067250, 60.22268384422984155 ) ) ;
#8412=CIRCLE ( 'NONE', #6837, 1.500000000000001332 ) ;
#8413=EDGE_CURVE ( 'NONE', #12114, #21033, #16459, .T. ) ;
#8415=( BOUNDED_CURVE ( )  B_SPLINE_CURVE ( 3, ( #28709, #6227, #30859, #16228 ),
 .UNSPECIFIED., .F., .F. ) 
 B_SPLINE_CURVE_WITH_KNOTS ( ( 4, 4 ),
 ( 5.497787143782109531, 6.283185307179586232 ),
 .UNSPECIFIED. ) 
 CURVE ( )  GEOMETRIC_REPRESENTATION_ITEM ( )  RATIONAL_B_SPLINE_CURVE ( ( 1.000000000000000000, 0.9492530216741874582, 0.9492530216741874582, 1.000000000000000000 ) ) 
 REPRESENTATION_ITEM ( '' )  );
#8417=VECTOR ( 'NONE', #1352, 1000.000000000000114 ) ;
#8422=TOROIDAL_SURFACE ( 'NONE', #3156, 1.899999999999999467, 0.1000000000000000056 ) ;
#8423=ORIENTED_EDGE ( 'NONE', *, *, #16443, .F. ) ;
#8424=AXIS2_PLACEMENT_3D ( 'NONE', #3781, #16252, #31365 ) ;
#8427=EDGE_CURVE ( 'NONE', #8280, #2451, #15811, .T. ) ;
#8429=CARTESIAN_POINT ( 'NONE',  ( -40.69193635511749108, 9.347952559758583746, 39.44930799450052206 ) ) ;
#8431=ORIENTED_EDGE ( 'NONE', *, *, #2408, .F. ) ;
#8433=CARTESIAN_POINT ( 'NONE',  ( -41.02113223168485234, 7.230835263863472306, 39.54930799450052348 ) ) ;
#8438=DIRECTION ( 'NONE',  ( -0.4848096202463430537, -0.8746197071393926326, -9.920727850371701658E-18 ) ) ;
#8443=ORIENTED_EDGE ( 'NONE', *, *, #29864, .F. ) ;
#8448=ORIENTED_EDGE ( 'NONE', *, *, #8586, .T. ) ;
#8451=EDGE_CURVE ( 'NONE', #9995, #25118, #28001, .T. ) ;
#8459=EDGE_CURVE ( 'NONE', #27336, #27995, #14389, .T. ) ;
#8461=ADVANCED_FACE ( 'NONE', ( #11363 ), #18564, .T. ) ;
#8467=CARTESIAN_POINT ( 'NONE',  ( -40.58268305512095964, 6.836408824202115042, 34.54930799450052348 ) ) ;
#8481=EDGE_LOOP ( 'NONE', ( #2771, #30404, #12044, #21320 ) ) ;
#8483=DIRECTION ( 'NONE',  ( 0.8746197071393926326, -0.4848096202463430537, -8.676864087101709653E-18 ) ) ;
#8489=CARTESIAN_POINT ( 'NONE',  ( -40.68074350590972443, 6.811995273158242270, 34.67891654026473702 ) ) ;
#8491=ORIENTED_EDGE ( 'NONE', *, *, #18488, .F. ) ;
#8494=DIRECTION ( 'NONE',  ( 0.8746197071393925215, -0.4848096202463429982, -8.676864087101708112E-18 ) ) ;
#8495=EDGE_LOOP ( 'NONE', ( #24135, #11001, #30540, #10185, #7715 ) ) ;
#8500=ORIENTED_EDGE ( 'NONE', *, *, #707, .T. ) ;
#8508=CARTESIAN_POINT ( 'NONE',  ( -40.16174044770769314, 7.468546898574135895, 60.44930799450051495 ) ) ;
#8513=VERTEX_POINT ( 'NONE', #11209 ) ;
#8517=CARTESIAN_POINT ( 'NONE',  ( -41.08785830660041682, 9.277514380576528552, 39.44930799450052206 ) ) ;
#8525=DIRECTION ( 'NONE',  ( -0.9612616959383221138, -0.2756373558169876170, 0.000000000000000000 ) ) ;
#8527=LINE ( 'NONE', #14752, #7298 ) ;
#8528=LINE ( 'NONE', #23302, #30300 ) ;
#8532=EDGE_CURVE ( 'NONE', #3549, #29624, #3885, .T. ) ;
#8536=CIRCLE ( 'NONE', #2231, 0.2000000000000012601 ) ;
#8545=ORIENTED_EDGE ( 'NONE', *, *, #20529, .T. ) ;
#8554=DIRECTION ( 'NONE',  ( -0.2756373558170082672, 0.9612616959383162296, 6.938893903907184201E-14 ) ) ;
#8557=AXIS2_PLACEMENT_3D ( 'NONE', #19795, #14560, #32125 ) ;
#8561=CARTESIAN_POINT ( 'NONE',  ( -40.98902310965377183, 10.38401719860223160, 36.52712545380572351 ) ) ;
#8562=CARTESIAN_POINT ( 'NONE',  ( -43.68921302925062378, 1.179890886355839275, 34.64930799450052490 ) ) ;
#8569=DIRECTION ( 'NONE',  ( 0.9612616959383207815, 0.2756373558169927240, 8.795445018804291370E-19 ) ) ;
#8573=EDGE_CURVE ( 'NONE', #14753, #14877, #5475, .T. ) ;
#8584=DIRECTION ( 'NONE',  ( 0.4848096202463645921, 0.8746197071393805311, 0.000000000000000000 ) ) ;
#8586=EDGE_CURVE ( 'NONE', #14081, #20995, #13849, .T. ) ;
#8589=CARTESIAN_POINT ( 'NONE',  ( -40.51045226066063520, 7.589116544599139758, 53.87859731638185679 ) ) ;
#8591=DIRECTION ( 'NONE',  ( -2.779292025043186357E-18, 1.288349127009862211E-17, -1.000000000000000000 ) ) ;
#8593=ORIENTED_EDGE ( 'NONE', *, *, #23785, .T. ) ;
#8597=ADVANCED_FACE ( 'NONE', ( #28 ), #6512, .T. ) ;
#8604=CARTESIAN_POINT ( 'NONE',  ( -40.67014616567487195, 6.832698218566653381, 39.23645843885594786 ) ) ;
#8607=DIRECTION ( 'NONE',  ( -0.8746197071393926326, 0.4848096202463430537, 8.676864087101709653E-18 ) ) ;
#8611=ORIENTED_EDGE ( 'NONE', *, *, #14163, .F. ) ;
#8613=VERTEX_POINT ( 'NONE', #17582 ) ;
#8619=DIRECTION ( 'NONE',  ( 1.188208965918165239E-16, 1.880121038077813132E-16, 1.000000000000000000 ) ) ;
#8621=CIRCLE ( 'NONE', #28037, 0.1000000000000004774 ) ;
#8622=LINE ( 'NONE', #24031, #28747 ) ;
#8626=ORIENTED_EDGE ( 'NONE', *, *, #123, .F. ) ;
#8627=CARTESIAN_POINT ( 'NONE',  ( -40.64500813507293486, 6.819128862114091305, 34.57932936825760351 ) ) ;
#8636=ORIENTED_EDGE ( 'NONE', *, *, #19465, .F. ) ;
#8637=FACE_OUTER_BOUND ( 'NONE', #14352, .T. ) ;
#8640=VERTEX_POINT ( 'NONE', #29580 ) ;
#8645=ADVANCED_FACE ( 'NONE', ( #7425 ), #22339, .T. ) ;
#8647=ORIENTED_EDGE ( 'NONE', *, *, #19142, .F. ) ;
#8650=ORIENTED_EDGE ( 'NONE', *, *, #1582, .F. ) ;
#8652=DIRECTION ( 'NONE',  ( 0.1949050434465267878, -0.6797146636928667052, 0.7071067811865480168 ) ) ;
#8660=VERTEX_POINT ( 'NONE', #9877 ) ;
#8666=ORIENTED_EDGE ( 'NONE', *, *, #28439, .T. ) ;
#8675=VECTOR ( 'NONE', #1724, 1000.000000000000114 ) ;
#8677=EDGE_LOOP ( 'NONE', ( #13508, #16878, #13030, #10456 ) ) ;
#8679=CARTESIAN_POINT ( 'NONE',  ( -40.47576471041815438, 7.229986682741244230, 38.88540264398079671 ) ) ;
#8681=CARTESIAN_POINT ( 'NONE',  ( -40.69230700880735441, 6.792718999258594792, 39.39980027471584378 ) ) ;
#8687=CARTESIAN_POINT ( 'NONE',  ( -38.88086318059457369, 4.491453754352391137, 47.04930799450051637 ) ) ;
#8698=VECTOR ( 'NONE', #76, 1000.000000000000114 ) ;
#8702=CIRCLE ( 'NONE', #27051, 0.8928932188134572900 ) ;
#8703=ORIENTED_EDGE ( 'NONE', *, *, #11132, .T. ) ;
#8705=FACE_OUTER_BOUND ( 'NONE', #20148, .T. ) ;
#8712=FACE_OUTER_BOUND ( 'NONE', #8481, .T. ) ;
#8714=SURFACE_STYLE_FILL_AREA ( #3783 ) ;
#8718=AXIS2_PLACEMENT_3D ( 'NONE', #28108, #15614, #15462 ) ;
#8719=LINE ( 'NONE', #13976, #12005 ) ;
#8720=CARTESIAN_POINT ( 'NONE',  ( -42.30123736278718383, 13.66041317296246937, 59.53596428539564300 ) ) ;
#8723=SPHERICAL_SURFACE ( 'NONE', #491, 0.1000000000000000056 ) ;
#8725=CARTESIAN_POINT ( 'NONE',  ( -40.50934420915148593, 7.581602792840986815, 60.22845019481307105 ) ) ;
#8728=CARTESIAN_POINT ( 'NONE',  ( -40.65093765668705572, 9.567768634527945792, 38.44930799450052916 ) ) ;
#8735=FACE_OUTER_BOUND ( 'NONE', #12525, .T. ) ;
#8738=VERTEX_POINT ( 'NONE', #7254 ) ;
#8744=EDGE_CURVE ( 'NONE', #23397, #23989, #23817, .T. ) ;
#8747=ORIENTED_EDGE ( 'NONE', *, *, #998, .F. ) ;
#8751=ORIENTED_EDGE ( 'NONE', *, *, #28914, .T. ) ;
#8758=CIRCLE ( 'NONE', #5093, 0.1000000000000006301 ) ;
#8763=CARTESIAN_POINT ( 'NONE',  ( -40.28779227465695811, 2.984619150196779369, 58.54930799450051637 ) ) ;
#8765=VERTEX_POINT ( 'NONE', #20359 ) ;
#8767=EDGE_CURVE ( 'NONE', #382, #31093, #17540, .T. ) ;
#8771=CIRCLE ( 'NONE', #11919, 0.1000000000000018235 ) ;
#8772=AXIS2_PLACEMENT_3D ( 'NONE', #25438, #2944, #12975 ) ;
#8775=ORIENTED_EDGE ( 'NONE', *, *, #7721, .T. ) ;
#8789=AXIS2_PLACEMENT_3D ( 'NONE', #4574, #22579, #7660 ) ;
#8793=CARTESIAN_POINT ( 'NONE',  ( -40.02667234278197839, 7.000595883235172678, 34.67240784960148403 ) ) ;
#8794=CARTESIAN_POINT ( 'NONE',  ( -40.68283709841080054, 6.807248601135447608, 34.79766250843303510 ) ) ;
#8796=CARTESIAN_POINT ( 'NONE',  ( -40.76967387488526384, 8.530668925462078889, 39.54930799450052348 ) ) ;
#8807=EDGE_CURVE ( 'NONE', #10919, #110, #32089, .T. ) ;
#8809=AXIS2_PLACEMENT_3D ( 'NONE', #16761, #19057, #7089 ) ;
#8810=ADVANCED_FACE ( 'NONE', ( #2809 ), #20532, .T. ) ;
#8812=DIRECTION ( 'NONE',  ( -0.3428121700606640565, -0.6184495258776567805, -0.7071067811865474617 ) ) ;
#8813=ORIENTED_EDGE ( 'NONE', *, *, #26793, .T. ) ;
#8816=LINE ( 'NONE', #18977, #30055 ) ;
#8818=ADVANCED_FACE ( 'NONE', ( #12840 ), #30387, .T. ) ;
#8819=VERTEX_POINT ( 'NONE', #8383 ) ;
#8822=LINE ( 'NONE', #31320, #4908 ) ;
#8824=ORIENTED_EDGE ( 'NONE', *, *, #18068, .F. ) ;
#8827=CARTESIAN_POINT ( 'NONE',  ( -40.62190982258952943, 6.851786633712847241, 39.32876805848002277 ) ) ;
#8828=FACE_OUTER_BOUND ( 'NONE', #16582, .T. ) ;
#8855=VERTEX_POINT ( 'NONE', #1635 ) ;
#8864=ORIENTED_EDGE ( 'NONE', *, *, #14005, .F. ) ;
#8870=( NAMED_UNIT ( * ) PLANE_ANGLE_UNIT ( ) SI_UNIT ( $, .RADIAN. ) );
#8875=DIRECTION ( 'NONE',  ( 0.8746197071393927436, -0.4848096202463423876, -1.277302113040827440E-17 ) ) ;
#8876=CIRCLE ( 'NONE', #3103, 0.1000000000000018235 ) ;
#8878=ORIENTED_EDGE ( 'NONE', *, *, #9003, .F. ) ;
#8879=( BOUNDED_CURVE ( )  B_SPLINE_CURVE ( 3, ( #6951, #2679, #17932, #3314 ),
 .UNSPECIFIED., .F., .F. ) 
 B_SPLINE_CURVE_WITH_KNOTS ( ( 4, 4 ),
 ( 4.712388980384692339, 6.283185307179584456 ),
 .UNSPECIFIED. ) 
 CURVE ( )  GEOMETRIC_REPRESENTATION_ITEM ( )  RATIONAL_B_SPLINE_CURVE ( ( 1.000000000000000000, 0.8047378541243654926, 0.8047378541243654926, 1.000000000000000000 ) ) 
 REPRESENTATION_ITEM ( '' )  );
#8881=CARTESIAN_POINT ( 'NONE',  ( -40.12089182904525586, 6.795442088152956472, 39.54930799450052348 ) ) ;
#8888=CIRCLE ( 'NONE', #13109, 0.09999999999999795164 ) ;
#8889=AXIS2_PLACEMENT_3D ( 'NONE', #6466, #25995, #31098 ) ;
#8892=ADVANCED_FACE ( 'NONE', ( #8705 ), #31834, .T. ) ;
#8898=ORIENTED_EDGE ( 'NONE', *, *, #13583, .F. ) ;
#8899=CARTESIAN_POINT ( 'NONE',  ( -41.74033427429298371, 15.41509661078533355, 35.54930799450051637 ) ) ;
#8900=LINE ( 'NONE', #31396, #28314 ) ;
#8902=CARTESIAN_POINT ( 'NONE',  ( -40.59290689585612455, 7.518854022824584149, 53.97121529040492760 ) ) ;
#8905=PRODUCT_DEFINITION ( 'UNKNOWN', '', #2422, #11126 ) ;
#8907=CIRCLE ( 'NONE', #28912, 2.000000000000001776 ) ;
#8920=DIRECTION ( 'NONE',  ( 0.9612616959383194493, 0.2756373558169974980, 8.795445018804946186E-19 ) ) ;
#8922=DIRECTION ( 'NONE',  ( 0.8746197071393925215, -0.4848096202463429982, -8.676864087101708112E-18 ) ) ;
#8925=CARTESIAN_POINT ( 'NONE',  ( -41.08785830660042393, 9.277514380576532105, 39.40788663826320715 ) ) ;
#8936=TOROIDAL_SURFACE ( 'NONE', #31478, 1.899999999999999467, 0.1000000000000000056 ) ;
#8938=CARTESIAN_POINT ( 'NONE',  ( -40.11286833322907341, 2.887657226147507306, 37.04930799450052348 ) ) ;
#8946=ADVANCED_FACE ( 'NONE', ( #26095 ), #13962, .F. ) ;
#8951=DIRECTION ( 'NONE',  ( 0.2756373558170082672, -0.9612616959383162296, 1.387778780781436840E-13 ) ) ;
#8957=DIRECTION ( 'NONE',  ( -0.8746197071393926326, 0.4848096202463430537, 8.676864087101709653E-18 ) ) ;
#8960=VECTOR ( 'NONE', #4726, 1000.000000000000227 ) ;
#8962=CARTESIAN_POINT ( 'NONE',  ( -40.74228355057324791, 8.435147512834893391, 39.46050754198200394 ) ) ;
#8968=AXIS2_PLACEMENT_3D ( 'NONE', #30285, #17799, #27823 ) ;
#8970=ORIENTED_EDGE ( 'NONE', *, *, #8427, .F. ) ;
#8978=CARTESIAN_POINT ( 'NONE',  ( -36.18493864628602807, 8.798967949527998655, 60.24930799450051211 ) ) ;
#8986=EDGE_LOOP ( 'NONE', ( #13146, #28919, #5080, #28783 ) ) ;
#8987=ORIENTED_EDGE ( 'NONE', *, *, #24798, .T. ) ;
#8988=DIRECTION ( 'NONE',  ( -0.8746197071393790878, 0.4848096202463673676, 1.277302113040196197E-17 ) ) ;
#8992=EDGE_CURVE ( 'NONE', #13785, #25827, #26580, .T. ) ;
#8993=DIRECTION ( 'NONE',  ( 0.8746197071393926326, -0.4848096202463430537, -8.676864087101709653E-18 ) ) ;
#8994=CARTESIAN_POINT ( 'NONE',  ( -40.64264863745309952, 6.822556421825392015, 39.42643144487149698 ) ) ;
#8995=DIRECTION ( 'NONE',  ( -0.8746197071393926326, 0.4848096202463430537, 8.676864087101709653E-18 ) ) ;
#9000=EDGE_LOOP ( 'NONE', ( #25350, #3801, #27129, #14058, #5591, #14773 ) ) ;
#9001=LINE ( 'NONE', #18997, #20782 ) ;
#9003=EDGE_CURVE ( 'NONE', #16786, #10137, #10744, .T. ) ;
#9006=CIRCLE ( 'NONE', #27348, 0.8999999999999991340 ) ;
#9012=ORIENTED_EDGE ( 'NONE', *, *, #28527, .T. ) ;
#9014=CYLINDRICAL_SURFACE ( 'NONE', #28238, 0.1000000000000007272 ) ;
#9020=DIRECTION ( 'NONE',  ( 0.2756373558169974980, -0.9612616959383194493, -1.315048337272770743E-17 ) ) ;
#9021=DIRECTION ( 'NONE',  ( 1.188208965918165239E-16, 1.880121038077813132E-16, 1.000000000000000000 ) ) ;
#9023=ORIENTED_EDGE ( 'NONE', *, *, #11646, .F. ) ;
#9026=DIRECTION ( 'NONE',  ( 0.4848096202463645921, 0.8746197071393805311, 0.000000000000000000 ) ) ;
#9027=CARTESIAN_POINT ( 'NONE',  ( -40.09616233467398416, 6.848043556934189091, 39.27380670015330821 ) ) ;
#9036=ORIENTED_EDGE ( 'NONE', *, *, #15632, .F. ) ;
#9039=CARTESIAN_POINT ( 'NONE',  ( -40.02540636251513462, 2.839176264122873050, 38.54930799450052348 ) ) ;
#9040=EDGE_CURVE ( 'NONE', #24287, #10826, #24382, .T. ) ;
#9047=AXIS2_PLACEMENT_3D ( 'NONE', #7386, #10008, #12639 ) ;
#9049=PLANE ( 'NONE',  #29900 ) ;
#9056=CARTESIAN_POINT ( 'NONE',  ( -40.28779227465695811, 2.984619150196779369, 59.04930799450051637 ) ) ;
#9061=DIRECTION ( 'NONE',  ( -0.2756373558169932791, 0.9612616959383205595, 2.447694389463610066E-31 ) ) ;
#9066=EDGE_CURVE ( 'NONE', #22928, #229, #24440, .T. ) ;
#9070=CARTESIAN_POINT ( 'NONE',  ( -40.59758774925371938, 7.567737757495683226, 38.44930799450052916 ) ) ;
#9074=ORIENTED_EDGE ( 'NONE', *, *, #24260, .T. ) ;
#9075=DIRECTION ( 'NONE',  ( -0.8746197071393926326, 0.4848096202463430537, 8.676864087101709653E-18 ) ) ;
#9078=EDGE_CURVE ( 'NONE', #23287, #14081, #2454, .T. ) ;
#9087=DIRECTION ( 'NONE',  ( 0.4848096202463637039, 0.8746197071393810862, 0.000000000000000000 ) ) ;
#9088=DIRECTION ( 'NONE',  ( -0.4848096202463069715, -0.8746197071394126166, 0.000000000000000000 ) ) ;
#9089=DIRECTION ( 'NONE',  ( -0.8746197071393926326, 0.4848096202463430537, 8.676864087101709653E-18 ) ) ;
#9100=AXIS2_PLACEMENT_3D ( 'NONE', #18162, #25882, #28187 ) ;
#9104=LINE ( 'NONE', #24197, #2555 ) ;
#9105=ORIENTED_EDGE ( 'NONE', *, *, #26631, .T. ) ;
#9106=CARTESIAN_POINT ( 'NONE',  ( -42.37913764077812573, 15.23192269303852697, 38.44930799450052916 ) ) ;
#9107=ORIENTED_EDGE ( 'NONE', *, *, #3804, .T. ) ;
#9111=CARTESIAN_POINT ( 'NONE',  ( -43.73393778030726509, 1.305471833569777695, 60.54930799450051637 ) ) ;
#9113=CARTESIAN_POINT ( 'NONE',  ( -42.35386648718987601, 15.27751306094253714, 35.56396816118280668 ) ) ;
#9115=DIRECTION ( 'NONE',  ( -0.2756373558169956106, 0.9612616959383197823, 0.000000000000000000 ) ) ;
#9117=CARTESIAN_POINT ( 'NONE',  ( -40.47970302497625994, 7.463434137431151250, 53.64930799450051779 ) ) ;
#9119=DIRECTION ( 'NONE',  ( 0.4151817967359032746, -0.9097384655268496711, -1.287451903529927940E-17 ) ) ;
#9120=VECTOR ( 'NONE', #22732, 1000.000000000000000 ) ;
#9121=EDGE_CURVE ( 'NONE', #22576, #23397, #13393, .T. ) ;
#9124=EDGE_LOOP ( 'NONE', ( #23420, #19121, #24753, #5458 ) ) ;
#9127=ORIENTED_EDGE ( 'NONE', *, *, #25718, .T. ) ;
#9131=ORIENTED_EDGE ( 'NONE', *, *, #29417, .T. ) ;
#9135=VECTOR ( 'NONE', #26949, 1000.000000000000227 ) ;
#9138=PLANE ( 'NONE',  #31864 ) ;
#9139=EDGE_CURVE ( 'NONE', #5852, #2479, #26912, .T. ) ;
#9143=CARTESIAN_POINT ( 'NONE',  ( -39.67555847965937943, 2.645252416024337361, 47.04930799450051637 ) ) ;
#9146=ORIENTED_EDGE ( 'NONE', *, *, #12262, .F. ) ;
#9148=ORIENTED_EDGE ( 'NONE', *, *, #10905, .F. ) ;
#9149=FACE_OUTER_BOUND ( 'NONE', #12416, .T. ) ;
#9150=ORIENTED_EDGE ( 'NONE', *, *, #18158, .T. ) ;
#9153=CARTESIAN_POINT ( 'NONE',  ( -40.49379808738640207, 7.146223304872329152, 38.94335650327652587 ) ) ;
#9155=CYLINDRICAL_SURFACE ( 'NONE', #17457, 2.000000000000001776 ) ;
#9160=EDGE_CURVE ( 'NONE', #10311, #18805, #29545, .T. ) ;
#9161=FACE_OUTER_BOUND ( 'NONE', #19841, .T. ) ;
#9162=CARTESIAN_POINT ( 'NONE',  ( -41.02113223168485234, 7.230835263863471418, 34.54930799450052348 ) ) ;
#9168=VECTOR ( 'NONE', #17170, 1000.000000000000114 ) ;
#9169=DIRECTION ( 'NONE',  ( 0.8746197071393926326, -0.4848096202463430537, -8.676864087101709653E-18 ) ) ;
#9171=CIRCLE ( 'NONE', #19655, 0.1000000000000018235 ) ;
#9179=EDGE_LOOP ( 'NONE', ( #30866, #27654 ) ) ;
#9182=LINE ( 'NONE', #21806, #20175 ) ;
#9187=ADVANCED_FACE ( 'NONE', ( #23117 ), #283, .T. ) ;
#9189=CIRCLE ( 'NONE', #26477, 1.142135311067127512 ) ;
#9190=VERTEX_POINT ( 'NONE', #28207 ) ;
#9193=CARTESIAN_POINT ( 'NONE',  ( -40.11085926462317275, 6.816553873983420608, 39.35917588466254813 ) ) ;
#9196=VERTEX_POINT ( 'NONE', #15729 ) ;
#9206=DIRECTION ( 'NONE',  ( 0.000000000000000000, 0.000000000000000000, -1.000000000000000000 ) ) ;
#9217=ADVANCED_FACE ( 'NONE', ( #25901 ), #3081, .T. ) ;
#9219=EDGE_LOOP ( 'NONE', ( #15712, #7550, #24489, #12452 ) ) ;
#9221=DIRECTION ( 'NONE',  ( -0.4151817967359235362, 0.9097384655268405673, 0.000000000000000000 ) ) ;
#9225=EDGE_CURVE ( 'NONE', #17298, #26367, #30351, .T. ) ;
#9236=CARTESIAN_POINT ( 'NONE',  ( -39.58809650894544774, 2.596771453999702661, 47.04930799450051637 ) ) ;
#9237=DIRECTION ( 'NONE',  ( -0.4848096202463636484, -0.8746197071393810862, 0.000000000000000000 ) ) ;
#9238=EDGE_CURVE ( 'NONE', #180, #10311, #13120, .T. ) ;
#9241=CARTESIAN_POINT ( 'NONE',  ( -40.42362386230406912, 8.537703822322061598, 34.55508635502626902 ) ) ;
#9243=AXIS2_PLACEMENT_3D ( 'NONE', #8938, #3853, #32081 ) ;
#9248=CARTESIAN_POINT ( 'NONE',  ( -43.64647580959332629, 1.256990871545142774, 53.64930799450051779 ) ) ;
#9255=ORIENTED_EDGE ( 'NONE', *, *, #26298, .F. ) ;
#9266=( BOUNDED_CURVE ( )  B_SPLINE_CURVE ( 3, ( #25594, #15105, #27417, #5421 ),
 .UNSPECIFIED., .F., .F. ) 
 B_SPLINE_CURVE_WITH_KNOTS ( ( 4, 4 ),
 ( 5.497787143782109531, 6.283185307179586232 ),
 .UNSPECIFIED. ) 
 CURVE ( )  GEOMETRIC_REPRESENTATION_ITEM ( )  RATIONAL_B_SPLINE_CURVE ( ( 1.000000000000000000, 0.9492530216741874582, 0.9492530216741874582, 1.000000000000000000 ) ) 
 REPRESENTATION_ITEM ( '' )  );
#9270=DIRECTION ( 'NONE',  ( 0.2756373558169954441, -0.9612616959383198934, 1.479773560108263451E-16 ) ) ;
#9273=DIRECTION ( 'NONE',  ( 0.4848096202463655358, 0.8746197071393799760, 0.000000000000000000 ) ) ;
#9275=ORIENTED_EDGE ( 'NONE', *, *, #25092, .F. ) ;
#9280=LINE ( 'NONE', #14374, #115 ) ;
#9282=CARTESIAN_POINT ( 'NONE',  ( -40.13663441551143762, 7.212672898651366182, 35.13832588636704912 ) ) ;
#9299=DIRECTION ( 'NONE',  ( 0.4848096202463636484, 0.8746197071393810862, 0.000000000000000000 ) ) ;
#9303=CARTESIAN_POINT ( 'NONE',  ( -42.92119432306954252, 16.03391241267916811, 37.04930799450052348 ) ) ;
#9309=DIRECTION ( 'NONE',  ( -0.2756373558169958327, 0.9612616959383198934, 0.000000000000000000 ) ) ;
#9310=ORIENTED_EDGE ( 'NONE', *, *, #12133, .F. ) ;
#9315=CARTESIAN_POINT ( 'NONE',  ( -40.56960242289655838, 7.470141326142095473, 38.67132538937698882 ) ) ;
#9316=CARTESIAN_POINT ( 'NONE',  ( -40.68572042366827191, 6.804601513393670587, 39.33474082486971213 ) ) ;
#9317=CARTESIAN_POINT ( 'NONE',  ( -40.51045226066063520, 7.589116544599141534, 60.22001867261916885 ) ) ;
#9322=CARTESIAN_POINT ( 'NONE',  ( -36.37788479535792163, 9.471851136684824368, 59.54930799450050927 ) ) ;
#9329=ORIENTED_EDGE ( 'NONE', *, *, #1393, .T. ) ;
#9332=ORIENTED_EDGE ( 'NONE', *, *, #32492, .F. ) ;
#9334=CYLINDRICAL_SURFACE ( 'NONE', #29838, 0.1000000000000028644 ) ;
#9335=CIRCLE ( 'NONE', #6729, 0.1000000000000008243 ) ;
#9340=ORIENTED_EDGE ( 'NONE', *, *, #30110, .F. ) ;
#9351=CARTESIAN_POINT ( 'NONE',  ( -40.61530068986830599, 9.443487761709571160, 39.52001867261917312 ) ) ;
#9352=AXIS2_PLACEMENT_3D ( 'NONE', #3062, #30982, #10644 ) ;
#9355=VERTEX_POINT ( 'NONE', #10974 ) ;
#9359=CIRCLE ( 'NONE', #13029, 0.09999999999999921452 ) ;
#9365=VERTEX_POINT ( 'NONE', #1260 ) ;
#9371=CARTESIAN_POINT ( 'NONE',  ( -40.18454328187963398, 7.548069831825862330, 60.44930799450051495 ) ) ;
#9375=EDGE_CURVE ( 'NONE', #23989, #23397, #29645, .T. ) ;
#9378=CARTESIAN_POINT ( 'NONE',  ( -40.11598084786749752, 7.671759737001394797, 53.64930799450051779 ) ) ;
#9380=ORIENTED_EDGE ( 'NONE', *, *, #9448, .T. ) ;
#9386=ORIENTED_EDGE ( 'NONE', *, *, #27106, .F. ) ;
#9391=AXIS2_PLACEMENT_3D ( 'NONE', #27520, #17164, #15049 ) ;
#9392=AXIS2_PLACEMENT_3D ( 'NONE', #25839, #20753, #17643 ) ;
#9395=CARTESIAN_POINT ( 'NONE',  ( -43.38408989745150990, 1.111547985471240008, 53.64930799450051779 ) ) ;
#9402=CYLINDRICAL_SURFACE ( 'NONE', #26635, 0.1000000000000018235 ) ;
#9406=DIRECTION ( 'NONE',  ( -0.9612616959383194493, -0.2756373558169972759, -8.795445018804907668E-19 ) ) ;
#9409=VECTOR ( 'NONE', #17855, 1000.000000000000114 ) ;
#9414=DIRECTION ( 'NONE',  ( 0.000000000000000000, 0.000000000000000000, -1.000000000000000000 ) ) ;
#9416=EDGE_CURVE ( 'NONE', #6416, #8280, #21282, .T. ) ;
#9431=AXIS2_PLACEMENT_3D ( 'NONE', #30568, #27451, #10217 ) ;
#9434=CARTESIAN_POINT ( 'NONE',  ( -40.18454328187963398, 7.548069831825862330, 60.54930799450051637 ) ) ;
#9435=AXIS2_PLACEMENT_3D ( 'NONE', #16698, #3353, #5350 ) ;
#9439=CARTESIAN_POINT ( 'NONE',  ( -43.64073206722599707, 1.267352857069778960, 34.64930799450052490 ) ) ;
#9440=EDGE_CURVE ( 'NONE', #5228, #2485, #24898, .T. ) ;
#9442=DIRECTION ( 'NONE',  ( 0.1949050434465250947, -0.6797146636928670382, 0.7071067811865481278 ) ) ;
#9446=CIRCLE ( 'NONE', #12592, 2.000000000000001776 ) ;
#9448=EDGE_CURVE ( 'NONE', #17902, #9841, #10797, .T. ) ;
#9452=VERTEX_POINT ( 'NONE', #22416 ) ;
#9454=ORIENTED_EDGE ( 'NONE', *, *, #3933, .F. ) ;
#9455=DIRECTION ( 'NONE',  ( -2.779292025043186357E-18, 1.288349127009862211E-17, -1.000000000000000000 ) ) ;
#9457=CIRCLE ( 'NONE', #13115, 0.09999999999999753530 ) ;
#9458=DIRECTION ( 'NONE',  ( 0.2756373558169973870, -0.9612616959383193382, -1.315048337272770435E-17 ) ) ;
#9466=ORIENTED_EDGE ( 'NONE', *, *, #3889, .F. ) ;
#9470=VERTEX_POINT ( 'NONE', #19302 ) ;
#9473=DIRECTION ( 'NONE',  ( 0.4848096202463637039, 0.8746197071393810862, 0.000000000000000000 ) ) ;
#9474=VECTOR ( 'NONE', #1316, 1000.000000000000114 ) ;
#9475=CARTESIAN_POINT ( 'NONE',  ( -40.47970302497625994, 7.463434137431150361, 60.29072935073781991 ) ) ;
#9476=DIRECTION ( 'NONE',  ( -0.8746197071393926326, 0.4848096202463430537, 8.676864087101709653E-18 ) ) ;
#9486=LINE ( 'NONE', #19483, #5877 ) ;
#9489=CARTESIAN_POINT ( 'NONE',  ( -40.37748943095153464, 8.220953018982690708, 54.59072935073782418 ) ) ;
#9493=DIRECTION ( 'NONE',  ( 0.4848096202463424986, 0.8746197071393928546, -2.220446049250312834E-16 ) ) ;
#9494=EDGE_LOOP ( 'NONE', ( #20381, #26116, #23964, #513 ) ) ;
#9495=DIRECTION ( 'NONE',  ( 1.188208965918165239E-16, 1.880121038077813132E-16, 1.000000000000000000 ) ) ;
#9496=DIRECTION ( 'NONE',  ( 0.000000000000000000, 0.000000000000000000, -1.000000000000000000 ) ) ;
#9500=LINE ( 'NONE', #22119, #26858 ) ;
#9518=CARTESIAN_POINT ( 'NONE',  ( -40.15599670534037102, 7.478908884098767196, 34.54930799450052348 ) ) ;
#9520=ORIENTED_EDGE ( 'NONE', *, *, #12170, .F. ) ;
#9525=VECTOR ( 'NONE', #25352, 1000.000000000000114 ) ;
#9534=FACE_OUTER_BOUND ( 'NONE', #15714, .T. ) ;
#9550=AXIS2_PLACEMENT_3D ( 'NONE', #12409, #5346, #23047 ) ;
#9552=DIRECTION ( 'NONE',  ( -0.9612616959383205595, -0.2756373558169932236, 1.660411357259282445E-16 ) ) ;
#9555=ORIENTED_EDGE ( 'NONE', *, *, #21076, .T. ) ;
#9558=SPHERICAL_SURFACE ( 'NONE', #17865, 0.1000000000000000056 ) ;
#9559=DIRECTION ( 'NONE',  ( -0.8746197071393926326, 0.4848096202463430537, 8.676864087101709653E-18 ) ) ;
#9563=VECTOR ( 'NONE', #3127, 1000.000000000000000 ) ;
#9567=ORIENTED_EDGE ( 'NONE', *, *, #15966, .T. ) ;
#9579=LINE ( 'NONE', #54, #25658 ) ;
#9582=LINE ( 'NONE', #12039, #16270 ) ;
#9591=CIRCLE ( 'NONE', #27935, 1.500000000000001332 ) ;
#9599=VERTEX_POINT ( 'NONE', #25706 ) ;
#9602=DIRECTION ( 'NONE',  ( 1.188208965918165239E-16, 1.880121038077813132E-16, 1.000000000000000000 ) ) ;
#9603=DIRECTION ( 'NONE',  ( 0.3958453973320081309, 0.7141240004913237405, 0.5773502691896250649 ) ) ;
#9605=DIRECTION ( 'NONE',  ( 0.9612616959383266657, 0.2756373558169715743, 0.000000000000000000 ) ) ;
#9608=CARTESIAN_POINT ( 'NONE',  ( -40.48129536610376533, 8.613360132207176889, 39.44930799450052206 ) ) ;
#9611=DIRECTION ( 'NONE',  ( -0.9612616959383208926, -0.2756373558169918914, 1.188214443479423533E-14 ) ) ;
#9617=EDGE_CURVE ( 'NONE', #30017, #27962, #15371, .T. ) ;
#9620=AXIS2_PLACEMENT_3D ( 'NONE', #28308, #28471, #734 ) ;
#9623=TOROIDAL_SURFACE ( 'NONE', #12780, 1.299999999999999822, 0.1000000000000000056 ) ;
#9627=EDGE_CURVE ( 'NONE', #26975, #29567, #12305, .T. ) ;
#9631=ADVANCED_FACE ( 'NONE', ( #30642 ), #15953, .T. ) ;
#9632=EDGE_LOOP ( 'NONE', ( #7107, #28517, #8747 ) ) ;
#9636=AXIS2_PLACEMENT_3D ( 'NONE', #28625, #13382, #10760 ) ;
#9637=DIRECTION ( 'NONE',  ( 0.2756373558169974980, -0.9612616959383193382, -1.315048337272770589E-17 ) ) ;
#9638=CARTESIAN_POINT ( 'NONE',  ( -41.34584395867850048, 11.59800658573647247, 57.04930799450051637 ) ) ;
#9646=CARTESIAN_POINT ( 'NONE',  ( -40.65487266620045403, 9.475231293617262907, 34.66144002885648945 ) ) ;
#9652=DIRECTION ( 'NONE',  ( -0.7141240004913198547, 0.3958453973320100738, -0.5773502691896283956 ) ) ;
#9657=CARTESIAN_POINT ( 'NONE',  ( -40.23397449525940317, 6.794506605641760899, 39.44930799450052206 ) ) ;
#9664=DIRECTION ( 'NONE',  ( 0.8746197071393928546, -0.4848096202463424986, -1.277302113040826515E-17 ) ) ;
#9668=ADVANCED_FACE ( 'NONE', ( #23243 ), #30792, .F. ) ;
#9669=ORIENTED_EDGE ( 'NONE', *, *, #22634, .T. ) ;
#9676=DIRECTION ( 'NONE',  ( 0.2756373558169942228, -0.9612616959383203374, 0.000000000000000000 ) ) ;
#9677=DIRECTION ( 'NONE',  ( -0.9612616959383207815, -0.2756373558169926685, -8.795445018804289444E-19 ) ) ;
#9678=CARTESIAN_POINT ( 'NONE',  ( -41.02687597405218156, 7.220473278338834788, 60.44930799450051495 ) ) ;
#9685=VECTOR ( 'NONE', #16172, 1000.000000000000000 ) ;
#9688=TOROIDAL_SURFACE ( 'NONE', #20671, 1.299999999999999822, 0.1000000000000000056 ) ;
#9689=CARTESIAN_POINT ( 'NONE',  ( -40.70335362822509495, 9.387769322903324110, 34.54930799450052348 ) ) ;
#9690=CARTESIAN_POINT ( 'NONE',  ( -40.69571722278732295, 6.786566810383045656, 34.64930799450051779 ) ) ;
#9691=LINE ( 'NONE', #24451, #1090 ) ;
#9695=VERTEX_POINT ( 'NONE', #7666 ) ;
#9697=CARTESIAN_POINT ( 'NONE',  ( -39.59300248568538194, 7.744584186742828891, 61.94930799450052206 ) ) ;
#9699=CARTESIAN_POINT ( 'NONE',  ( -41.63422246745999189, 11.51531537899137447, 57.95249952744806166 ) ) ;
#9700=VERTEX_POINT ( 'NONE', #15209 ) ;
#9706=DIRECTION ( 'NONE',  ( -0.2756373558169932236, 0.9612616959383204485, -1.479773560108267395E-16 ) ) ;
#9712=ORIENTED_EDGE ( 'NONE', *, *, #18523, .T. ) ;
#9714=LINE ( 'NONE', #29574, #2327 ) ;
#9715=CARTESIAN_POINT ( 'NONE',  ( -40.51442171646695556, 7.400645970086839220, 60.37414278400746070 ) ) ;
#9717=EDGE_CURVE ( 'NONE', #8855, #777, #8621, .T. ) ;
#9718=ORIENTED_EDGE ( 'NONE', *, *, #11600, .F. ) ;
#9719=EDGE_CURVE ( 'NONE', #19450, #19780, #31169, .T. ) ;
#9721=CARTESIAN_POINT ( 'NONE',  ( -39.67555847965937943, 2.645252416024336028, 49.04930799450051637 ) ) ;
#9724=CARTESIAN_POINT ( 'NONE',  ( -40.11286833322908052, 2.887657226147509970, 59.04930799450051637 ) ) ;
#9729=VECTOR ( 'NONE', #3895, 1000.000000000000000 ) ;
#9737=CARTESIAN_POINT ( 'NONE',  ( -40.15599670534037102, 7.478908884098773413, 38.44930799450052916 ) ) ;
#9739=AXIS2_PLACEMENT_3D ( 'NONE', #8111, #3004, #720 ) ;
#9743=DIRECTION ( 'NONE',  ( -0.3958453973320076313, -0.7141240004913228523, 0.5773502691896265082 ) ) ;
#9745=VERTEX_POINT ( 'NONE', #3862 ) ;
#9757=MECHANICAL_DESIGN_GEOMETRIC_PRESENTATION_REPRESENTATION('',(#20765),#28110);
#9759=EDGE_CURVE ( 'NONE', #2732, #27609, #13556, .T. ) ;
#9763=FACE_OUTER_BOUND ( 'NONE', #27399, .T. ) ;
#9764=EDGE_CURVE ( 'NONE', #6401, #4559, #26448, .T. ) ;
#9765=TOROIDAL_SURFACE ( 'NONE', #9243, 1.899999999999999467, 0.1000000000000000056 ) ;
#9767=CARTESIAN_POINT ( 'NONE',  ( -40.79464149312965304, 8.438755658900303658, 34.56232498761289662 ) ) ;
#9768=ORIENTED_EDGE ( 'NONE', *, *, #6569, .T. ) ;
#9772=ORIENTED_EDGE ( 'NONE', *, *, #10861, .T. ) ;
#9775=PLANE ( 'NONE',  #21034 ) ;
#9776=DIRECTION ( 'NONE',  ( -1.188208965918165239E-16, -1.880121038077813132E-16, -1.000000000000000000 ) ) ;
#9777=DIRECTION ( 'NONE',  ( 0.4848096202463366700, 0.8746197071393961853, 9.920727850372755527E-18 ) ) ;
#9792=ORIENTED_EDGE ( 'NONE', *, *, #7414, .T. ) ;
#9796=VERTEX_POINT ( 'NONE', #23721 ) ;
#9797=ORIENTED_EDGE ( 'NONE', *, *, #5970, .T. ) ;
#9798=DIRECTION ( 'NONE',  ( 2.779292025043186357E-18, -1.288349127009862211E-17, 1.000000000000000000 ) ) ;
#9802=CARTESIAN_POINT ( 'NONE',  ( -41.77464577679392477, 3.808795504615560379, 49.04930799450051637 ) ) ;
#9811=FACE_OUTER_BOUND ( 'NONE', #10156, .T. ) ;
#9820=ORIENTED_EDGE ( 'NONE', *, *, #11767, .F. ) ;
#9833=ORIENTED_EDGE ( 'NONE', *, *, #707, .F. ) ;
#9835=ADVANCED_FACE ( 'NONE', ( #6323 ), #16325, .F. ) ;
#9837=DIRECTION ( 'NONE',  ( -1.188208965918165239E-16, -1.880121038077813132E-16, -1.000000000000000000 ) ) ;
#9841=VERTEX_POINT ( 'NONE', #1390 ) ;
#9846=CARTESIAN_POINT ( 'NONE',  ( -40.47630348341014184, 7.507564784836493921, 35.32879591952760734 ) ) ;
#9853=ORIENTED_EDGE ( 'NONE', *, *, #12500, .F. ) ;
#9860=ORIENTED_EDGE ( 'NONE', *, *, #26603, .F. ) ;
#9863=ORIENTED_EDGE ( 'NONE', *, *, #11646, .T. ) ;
#9865=EDGE_CURVE ( 'NONE', #21721, #15784, #2374, .T. ) ;
#9866=CARTESIAN_POINT ( 'NONE',  ( -39.85048242108726413, 2.742214340073605428, 45.04930799450051637 ) ) ;
#9869=ORIENTED_EDGE ( 'NONE', *, *, #2990, .T. ) ;
#9870=VECTOR ( 'NONE', #2502, 1000.000000000000000 ) ;
#9875=CIRCLE ( 'NONE', #20339, 0.1000000000000007688 ) ;
#9876=VERTEX_POINT ( 'NONE', #20048 ) ;
#9877=CARTESIAN_POINT ( 'NONE',  ( -43.64647580959332629, 1.256990871545142774, 60.54930799450051637 ) ) ;
#9878=LINE ( 'NONE', #20692, #23195 ) ;
#9881=CARTESIAN_POINT ( 'NONE',  ( -40.50726676055796105, 7.559560307024983494, 60.44930799450051495 ) ) ;
#9882=DIRECTION ( 'NONE',  ( 0.4848096202463424986, 0.8746197071393928546, -2.220446049250312834E-16 ) ) ;
#9885=LINE ( 'NONE', #3700, #290 ) ;
#9886=ADVANCED_FACE ( 'NONE', ( #15295 ), #7746, .T. ) ;
#9890=ORIENTED_EDGE ( 'NONE', *, *, #5499, .T. ) ;
#9904=CARTESIAN_POINT ( 'NONE',  ( -43.29088418437023478, 1.073429008971243714, 39.44930799450052916 ) ) ;
#9905=DIRECTION ( 'NONE',  ( 0.000000000000000000, 0.000000000000000000, -1.000000000000000000 ) ) ;
#9917=AXIS2_PLACEMENT_3D ( 'NONE', #17971, #15359, #25370 ) ;
#9925=DIRECTION ( 'NONE',  ( 0.4848096202463627602, 0.8746197071393815303, 0.000000000000000000 ) ) ;
#9944=EDGE_CURVE ( 'NONE', #5139, #3439, #3934, .T. ) ;
#9945=EDGE_LOOP ( 'NONE', ( #12203, #17606, #4155, #4008 ) ) ;
#9951=AXIS2_PLACEMENT_3D ( 'NONE', #11236, #3837, #14020 ) ;
#9952=VERTEX_POINT ( 'NONE', #9881 ) ;
#9955=CIRCLE ( 'NONE', #12048, 0.1000000000000014905 ) ;
#9969=LINE ( 'NONE', #30319, #26333 ) ;
#9985=AXIS2_PLACEMENT_3D ( 'NONE', #2832, #22699, #27951 ) ;
#9988=DIRECTION ( 'NONE',  ( -0.9612616959383193382, -0.2756373558169973870, -8.795445018804928853E-19 ) ) ;
#9990=EDGE_CURVE ( 'NONE', #18712, #2479, #28577, .T. ) ;
#9992=DIRECTION ( 'NONE',  ( -0.2250569586005335410, 0.7848668881104262640, -0.5773502691896259531 ) ) ;
#9994=CIRCLE ( 'NONE', #31984, 1.142135311067127512 ) ;
#9995=VERTEX_POINT ( 'NONE', #13646 ) ;
#10008=DIRECTION ( 'NONE',  ( -2.779292025043186742E-18, 1.288349127009862365E-17, -1.000000000000000000 ) ) ;
#10011=ORIENTED_EDGE ( 'NONE', *, *, #27073, .T. ) ;
#10013=CARTESIAN_POINT ( 'NONE',  ( -39.85048242108726413, 2.742214340073605428, 49.04930799450051637 ) ) ;
#10019=DIRECTION ( 'NONE',  ( -0.6184495258776567805, 0.3428121700606641120, -0.7071067811865474617 ) ) ;
#10020=DIRECTION ( 'NONE',  ( -0.2756373558169974980, 0.9612616959383193382, 1.315048337272770589E-17 ) ) ;
#10027=ORIENTED_EDGE ( 'NONE', *, *, #19334, .T. ) ;
#10034=EDGE_CURVE ( 'NONE', #11721, #3679, #30394, .T. ) ;
#10037=CIRCLE ( 'NONE', #584, 0.1000000000000006301 ) ;
#10038=EDGE_LOOP ( 'NONE', ( #3237, #12248, #18229, #25245 ) ) ;
#10044=EDGE_CURVE ( 'NONE', #32358, #3661, #25466, .T. ) ;
#10045=ORIENTED_EDGE ( 'NONE', *, *, #12235, .T. ) ;
#10046=CIRCLE ( 'NONE', #3208, 0.1000000000000020595 ) ;
#10055=DIRECTION ( 'NONE',  ( -0.2756373558169959437, 0.9612616959383197823, 0.000000000000000000 ) ) ;
#10064=FACE_OUTER_BOUND ( 'NONE', #12389, .T. ) ;
#10068=CARTESIAN_POINT ( 'NONE',  ( -40.15225626691278649, 6.735663658092487793, 53.64930799450051779 ) ) ;
#10071=FACE_OUTER_BOUND ( 'NONE', #5003, .T. ) ;
#10075=FACE_OUTER_BOUND ( 'NONE', #21476, .T. ) ;
#10078=CARTESIAN_POINT ( 'NONE',  ( -41.63422246745999189, 11.51531537899137447, 56.14611646155296398 ) ) ;
#10079=VECTOR ( 'NONE', #30045, 1000.000000000000000 ) ;
#10080=AXIS2_PLACEMENT_3D ( 'NONE', #13207, #718, #3163 ) ;
#10082=AXIS2_PLACEMENT_3D ( 'NONE', #24332, #1858, #28953 ) ;
#10083=ORIENTED_EDGE ( 'NONE', *, *, #3033, .T. ) ;
#10087=EDGE_CURVE ( 'NONE', #15339, #31154, #27512, .T. ) ;
#10095=CARTESIAN_POINT ( 'NONE',  ( -40.82429435450200828, 8.450784283921491280, 34.58262810048215385 ) ) ;
#10101=CARTESIAN_POINT ( 'NONE',  ( -40.69520067770175586, 6.787173244583783571, 39.45492316879074934 ) ) ;
#10104=DIRECTION ( 'NONE',  ( -0.7936353835927094647, 0.4399192766786362285, -0.4202545751282172337 ) ) ;
#10105=DIRECTION ( 'NONE',  ( 0.2756373558169947779, -0.9612616959383200044, 0.000000000000000000 ) ) ;
#10106=DIRECTION ( 'NONE',  ( 0.8746197071393925215, -0.4848096202463429982, -8.676864087101708112E-18 ) ) ;
#10108=ORIENTED_EDGE ( 'NONE', *, *, #4991, .T. ) ;
#10109=CARTESIAN_POINT ( 'NONE',  ( -43.38408989745150990, 1.111547985471240008, 53.64930799450051779 ) ) ;
#10119=ORIENTED_EDGE ( 'NONE', *, *, #11648, .T. ) ;
#10123=EDGE_CURVE ( 'NONE', #9745, #16786, #13485, .T. ) ;
#10124=ORIENTED_EDGE ( 'NONE', *, *, #6591, .F. ) ;
#10129=EDGE_CURVE ( 'NONE', #13517, #2319, #30146, .T. ) ;
#10132=AXIS2_PLACEMENT_3D ( 'NONE', #30157, #9476, #24399 ) ;
#10137=VERTEX_POINT ( 'NONE', #3779 ) ;
#10145=( BOUNDED_CURVE ( )  B_SPLINE_CURVE ( 3, ( #28435, #3637, #11195, #19537 ),
 .UNSPECIFIED., .F., .F. ) 
 B_SPLINE_CURVE_WITH_KNOTS ( ( 4, 4 ),
 ( 4.712388980384698556, 5.497787143782102426 ),
 .UNSPECIFIED. ) 
 CURVE ( )  GEOMETRIC_REPRESENTATION_ITEM ( )  RATIONAL_B_SPLINE_CURVE ( ( 1.000000000000000000, 0.9492530216741968951, 0.9492530216741968951, 1.000000000000000000 ) ) 
 REPRESENTATION_ITEM ( '' )  );
#10147=DIRECTION ( 'NONE',  ( -0.4848096202463430537, -0.8746197071393926326, -9.920727850371701658E-18 ) ) ;
#10151=ORIENTED_EDGE ( 'NONE', *, *, #30846, .T. ) ;
#10156=EDGE_LOOP ( 'NONE', ( #7692, #3702, #32112, #18463 ) ) ;
#10161=AXIS2_PLACEMENT_3D ( 'NONE', #15544, #17522, #32306 ) ;
#10164=ORIENTED_EDGE ( 'NONE', *, *, #3362, .F. ) ;
#10168=CIRCLE ( 'NONE', #28521, 0.1000000000000018235 ) ;
#10169=CARTESIAN_POINT ( 'NONE',  ( -40.11967773290336226, 9.763195579837789850, 35.54930799450052348 ) ) ;
#10173=ORIENTED_EDGE ( 'NONE', *, *, #9225, .T. ) ;
#10175=VERTEX_POINT ( 'NONE', #13802 ) ;
#10178=DIRECTION ( 'NONE',  ( -0.1949050434465268433, 0.6797146636928677044, 0.7071067811865470176 ) ) ;
#10185=ORIENTED_EDGE ( 'NONE', *, *, #27616, .F. ) ;
#10191=ORIENTED_EDGE ( 'NONE', *, *, #28606, .F. ) ;
#10195=EDGE_CURVE ( 'NONE', #18016, #17431, #28544, .T. ) ;
#10198=AXIS2_PLACEMENT_3D ( 'NONE', #11695, #29243, #21350 ) ;
#10201=DIRECTION ( 'NONE',  ( 0.000000000000000000, 0.000000000000000000, 1.000000000000000000 ) ) ;
#10205=AXIS2_PLACEMENT_3D ( 'NONE', #12831, #22823, #30382 ) ;
#10214=CARTESIAN_POINT ( 'NONE',  ( -42.22138300640814634, 14.68176690255379313, 38.09144330556765112 ) ) ;
#10217=DIRECTION ( 'NONE',  ( -0.4848096202463429427, -0.8746197071393925215, 2.352477780477436787E-16 ) ) ;
#10221=ORIENTED_EDGE ( 'NONE', *, *, #2248, .T. ) ;
#10224=CARTESIAN_POINT ( 'NONE',  ( -40.18454328187963398, 7.548069831825862330, 53.80788663826320573 ) ) ;
#10228=DIRECTION ( 'NONE',  ( 0.9612616959383221138, 0.2756373558169876170, 0.000000000000000000 ) ) ;
#10233=ORIENTED_EDGE ( 'NONE', *, *, #24724, .F. ) ;
#10239=DIRECTION ( 'NONE',  ( 0.8746197071393926326, -0.4848096202463430537, -8.676864087101709653E-18 ) ) ;
#10244=EDGE_CURVE ( 'NONE', #30572, #11324, #1641, .T. ) ;
#10248=CARTESIAN_POINT ( 'NONE',  ( -42.66751614955960292, 15.14923148629343430, 38.54930799450052348 ) ) ;
#10251=CARTESIAN_POINT ( 'NONE',  ( -40.69343167531472005, 8.234387981831401859, 54.54930799450051637 ) ) ;
#10254=ADVANCED_FACE ( 'NONE', ( #2135 ), #19847, .F. ) ;
#10258=CARTESIAN_POINT ( 'NONE',  ( -42.50976151518962354, 14.59907569580870224, 38.09144330556765112 ) ) ;
#10259=VERTEX_POINT ( 'NONE', #17553 ) ;
#10260=VECTOR ( 'NONE', #21199, 1000.000000000000114 ) ;
#10262=CARTESIAN_POINT ( 'NONE',  ( -41.88090303775678791, 13.82677487427666385, 59.46671529104048659 ) ) ;
#10264=CARTESIAN_POINT ( 'NONE',  ( -40.69575244446413365, 6.786495028291348319, 39.45034024385534366 ) ) ;
#10265=ORIENTED_EDGE ( 'NONE', *, *, #13638, .F. ) ;
#10267=FACE_OUTER_BOUND ( 'NONE', #9632, .T. ) ;
#10270=DIRECTION ( 'NONE',  ( -1.188208965918165239E-16, -1.880121038077813132E-16, -1.000000000000000000 ) ) ;
#10281=CARTESIAN_POINT ( 'NONE',  ( -40.61178118339597631, 9.038025460530262123, 57.95249952744806166 ) ) ;
#10298=FACE_OUTER_BOUND ( 'NONE', #1083, .T. ) ;
#10301=AXIS2_PLACEMENT_3D ( 'NONE', #25316, #25150, #2668 ) ;
#10305=DIRECTION ( 'NONE',  ( 0.9612616959383207815, 0.2756373558169926685, 8.795445018804289444E-19 ) ) ;
#10306=DIRECTION ( 'NONE',  ( 0.000000000000000000, -8.673617379884027583E-16, -1.000000000000000000 ) ) ;
#10307=FACE_OUTER_BOUND ( 'NONE', #18735, .T. ) ;
#10309=DIRECTION ( 'NONE',  ( 2.779292025043186357E-18, -1.288349127009862211E-17, 1.000000000000000000 ) ) ;
#10311=VERTEX_POINT ( 'NONE', #9689 ) ;
#10319=ADVANCED_FACE ( 'NONE', ( #12649 ), #17572, .T. ) ;
#10323=ORIENTED_EDGE ( 'NONE', *, *, #20200, .T. ) ;
#10326=ORIENTED_EDGE ( 'NONE', *, *, #16847, .T. ) ;
#10327=( BOUNDED_CURVE ( )  B_SPLINE_CURVE ( 3, ( #26983, #27141, #21883, #4659 ),
 .UNSPECIFIED., .F., .F. ) 
 B_SPLINE_CURVE_WITH_KNOTS ( ( 4, 4 ),
 ( 3.141592653589793116, 3.657989679900455648 ),
 .UNSPECIFIED. ) 
 CURVE ( )  GEOMETRIC_REPRESENTATION_ITEM ( )  RATIONAL_B_SPLINE_CURVE ( ( 1.000000000000000000, 0.9779010246516581795, 0.9779010246516581795, 1.000000000000000000 ) ) 
 REPRESENTATION_ITEM ( '' )  );
#10328=DIRECTION ( 'NONE',  ( -0.2756373558169932236, 0.9612616959383205595, 2.536267806945839542E-31 ) ) ;
#10332=ORIENTED_EDGE ( 'NONE', *, *, #28084, .F. ) ;
#10334=ORIENTED_EDGE ( 'NONE', *, *, #16842, .T. ) ;
#10335=LINE ( 'NONE', #8517, #12084 ) ;
#10337=PLANE ( 'NONE',  #28447 ) ;
#10341=ORIENTED_EDGE ( 'NONE', *, *, #10654, .T. ) ;
#10342=CARTESIAN_POINT ( 'NONE',  ( -41.88090303775678080, 13.82677487427665675, 54.54930799450051637 ) ) ;
#10349=CARTESIAN_POINT ( 'NONE',  ( -40.60330327974818942, 7.565477138576675920, 53.88146687024393344 ) ) ;
#10351=EDGE_CURVE ( 'NONE', #9452, #12894, #7394, .T. ) ;
#10362=TOROIDAL_SURFACE ( 'NONE', #18718, 1.899999999999999467, 0.1000000000000000056 ) ;
#10364=CARTESIAN_POINT ( 'NONE',  ( -42.37913764077812573, 15.23192269303852875, 35.64930799450052490 ) ) ;
#10372=CARTESIAN_POINT ( 'NONE',  ( -40.58856461370174173, 7.499380836222957925, 60.14930799450051069 ) ) ;
#10374=DIRECTION ( 'NONE',  ( 0.000000000000000000, 0.000000000000000000, -1.000000000000000000 ) ) ;
#10380=DIRECTION ( 'NONE',  ( 0.8746197071393926326, -0.4848096202463430537, -8.676864087101709653E-18 ) ) ;
#10387=CARTESIAN_POINT ( 'NONE',  ( -40.12099660621118602, 7.356848571226523248, 38.85576968460465963 ) ) ;
#10388=ORIENTED_EDGE ( 'NONE', *, *, #22025, .T. ) ;
#10389=ORIENTED_EDGE ( 'NONE', *, *, #13581, .F. ) ;
#10400=VECTOR ( 'NONE', #23991, 1000.000000000000114 ) ;
#10413=AXIS2_PLACEMENT_3D ( 'NONE', #24787, #11835, #4441 ) ;
#10418=LINE ( 'NONE', #30605, #7079 ) ;
#10425=CARTESIAN_POINT ( 'NONE',  ( -40.47970302497625994, 7.463434137431151250, 60.54930799450051637 ) ) ;
#10426=AXIS2_PLACEMENT_3D ( 'NONE', #25321, #5616, #23336 ) ;
#10431=ORIENTED_EDGE ( 'NONE', *, *, #10542, .F. ) ;
#10443=AXIS2_PLACEMENT_3D ( 'NONE', #16063, #13137, #652 ) ;
#10444=CIRCLE ( 'NONE', #10980, 2.000000000000001776 ) ;
#10445=EDGE_CURVE ( 'NONE', #11324, #23543, #19125, .T. ) ;
#10447=CARTESIAN_POINT ( 'NONE',  ( -37.42114908093812176, 11.86897798031838391, 60.44930799450051495 ) ) ;
#10450=ORIENTED_EDGE ( 'NONE', *, *, #32430, .F. ) ;
#10451=VERTEX_POINT ( 'NONE', #25586 ) ;
#10456=ORIENTED_EDGE ( 'NONE', *, *, #15069, .F. ) ;
#10459=CARTESIAN_POINT ( 'NONE',  ( -42.38687957179149635, 4.148162238787999279, 37.04930799450052348 ) ) ;
#10469=EDGE_CURVE ( 'NONE', #5512, #1774, #18352, .T. ) ;
#10471=LINE ( 'NONE', #17521, #5321 ) ;
#10479=ORIENTED_EDGE ( 'NONE', *, *, #13638, .T. ) ;
#10484=EDGE_LOOP ( 'NONE', ( #17343, #10045, #13259, #26021 ) ) ;
#10493=VECTOR ( 'NONE', #20408, 1000.000000000000114 ) ;
#10500=EDGE_LOOP ( 'NONE', ( #27325, #27178, #945 ) ) ;
#10503=ORIENTED_EDGE ( 'NONE', *, *, #9375, .T. ) ;
#10506=CARTESIAN_POINT ( 'NONE',  ( -39.58809650894544774, 2.596771453999702661, 49.04930799450051637 ) ) ;
#10508=DIRECTION ( 'NONE',  ( 0.000000000000000000, 0.000000000000000000, 1.000000000000000000 ) ) ;
#10520=AXIS2_PLACEMENT_3D ( 'NONE', #10447, #3039, #1950 ) ;
#10522=ORIENTED_EDGE ( 'NONE', *, *, #10195, .F. ) ;
#10523=AXIS2_PLACEMENT_3D ( 'NONE', #23801, #15780, #13648 ) ;
#10528=ORIENTED_EDGE ( 'NONE', *, *, #12619, .T. ) ;
#10532=EDGE_LOOP ( 'NONE', ( #4376, #11335, #24039, #6846, #18337 ) ) ;
#10535=LINE ( 'NONE', #13480, #31075 ) ;
#10541=CARTESIAN_POINT ( 'NONE',  ( -40.58117736050017754, 7.466252321088952648, 60.18657739374794602 ) ) ;
#10542=EDGE_CURVE ( 'NONE', #27140, #28668, #3744, .T. ) ;
#10543=DIRECTION ( 'NONE',  ( 0.000000000000000000, 0.000000000000000000, -1.000000000000000000 ) ) ;
#10545=EDGE_CURVE ( 'NONE', #27609, #9365, #4189, .T. ) ;
#10551=AXIS2_PLACEMENT_3D ( 'NONE', #31602, #6324, #28973 ) ;
#10554=DIRECTION ( 'NONE',  ( 0.8746197071393925215, -0.4848096202463429982, -8.676864087101708112E-18 ) ) ;
#10572=EDGE_CURVE ( 'NONE', #23334, #19780, #11293, .T. ) ;
#10574=VECTOR ( 'NONE', #2092, 1000.000000000000114 ) ;
#10580=CARTESIAN_POINT ( 'NONE',  ( -40.34207605779958072, 7.502898035225042506, 60.44930799450051495 ) ) ;
#10581=EDGE_CURVE ( 'NONE', #26808, #16322, #16970, .T. ) ;
#10582=CARTESIAN_POINT ( 'NONE',  ( -42.73182147790732444, -0.8057266458565844891, 61.94930799450052206 ) ) ;
#10584=EDGE_CURVE ( 'NONE', #32232, #1639, #20515, .T. ) ;
#10585=ADVANCED_FACE ( 'NONE', ( #8828 ), #31163, .F. ) ;
#10593=PLANE ( 'NONE',  #29261 ) ;
#10594=DIRECTION ( 'NONE',  ( -0.8746197071393926326, 0.4848096202463430537, 8.676864087101709653E-18 ) ) ;
#10600=CARTESIAN_POINT ( 'NONE',  ( -40.61197514715824752, 6.966360136513626955, 39.01065621547813578 ) ) ;
#10612=AXIS2_PLACEMENT_3D ( 'NONE', #9395, #32210, #14324 ) ;
#10622=ORIENTED_EDGE ( 'NONE', *, *, #2214, .T. ) ;
#10628=EDGE_LOOP ( 'NONE', ( #22164, #8448, #12909, #15941, #32487 ) ) ;
#10633=ORIENTED_EDGE ( 'NONE', *, *, #27914, .T. ) ;
#10637=DIRECTION ( 'NONE',  ( -1.431146867680865853E-17, -2.558717127065790464E-17, -1.000000000000000000 ) ) ;
#10639=LINE ( 'NONE', #18317, #27288 ) ;
#10641=CARTESIAN_POINT ( 'NONE',  ( -40.64522151305507691, 6.818818762547660839, 34.57215670535448027 ) ) ;
#10644=DIRECTION ( 'NONE',  ( 0.2756373558170018279, -0.9612616959383181170, 0.000000000000000000 ) ) ;
#10648=CIRCLE ( 'NONE', #28966, 1.899999999999999023 ) ;
#10654=EDGE_CURVE ( 'NONE', #13496, #5375, #13200, .T. ) ;
#10656=EDGE_CURVE ( 'NONE', #15237, #777, #10727, .T. ) ;
#10659=AXIS2_PLACEMENT_3D ( 'NONE', #28852, #4051, #11443 ) ;
#10662=DIRECTION ( 'NONE',  ( -0.9612616959383198934, -0.2756373558169956106, 0.000000000000000000 ) ) ;
#10663=VECTOR ( 'NONE', #17115, 1000.000000000000000 ) ;
#10664=VECTOR ( 'NONE', #15226, 1000.000000000000227 ) ;
#10665=DIRECTION ( 'NONE',  ( -0.9612616959383205595, -0.2756373558169931681, 1.660411357259282445E-16 ) ) ;
#10669=EDGE_CURVE ( 'NONE', #5852, #1546, #14411, .T. ) ;
#10672=DIRECTION ( 'NONE',  ( -0.4848096202463636484, -0.8746197071393810862, 0.000000000000000000 ) ) ;
#10685=AXIS2_PLACEMENT_3D ( 'NONE', #22345, #22505, #12844 ) ;
#10686=EDGE_CURVE ( 'NONE', #28686, #10826, #22108, .T. ) ;
#10688=CARTESIAN_POINT ( 'NONE',  ( -40.14651252454546437, 6.746025643617127088, 39.44930799450052206 ) ) ;
#10694=VECTOR ( 'NONE', #24309, 1000.000000000000000 ) ;
#10699=DIRECTION ( 'NONE',  ( -2.779292025043186357E-18, 1.288349127009862211E-17, -1.000000000000000000 ) ) ;
#10713=ORIENTED_EDGE ( 'NONE', *, *, #27347, .T. ) ;
#10715=DIRECTION ( 'NONE',  ( -0.4848096202463429427, -0.8746197071393925215, 2.352477780477436294E-16 ) ) ;
#10720=CARTESIAN_POINT ( 'NONE',  ( -40.06891218940336330, 7.538004613239522200, 38.80028690913361800 ) ) ;
#10727=( BOUNDED_CURVE ( )  B_SPLINE_CURVE ( 3, ( #14903, #26879, #2260, #27040 ),
 .UNSPECIFIED., .F., .F. ) 
 B_SPLINE_CURVE_WITH_KNOTS ( ( 4, 4 ),
 ( 4.652534634851591022, 4.712388980384696779 ),
 .UNSPECIFIED. ) 
 CURVE ( )  GEOMETRIC_REPRESENTATION_ITEM ( )  RATIONAL_B_SPLINE_CURVE ( ( 1.000000000000000000, 0.9997014770583808607, 0.9997014770583808607, 1.000000000000000000 ) ) 
 REPRESENTATION_ITEM ( '' )  );
#10733=EDGE_CURVE ( 'NONE', #17822, #29138, #19806, .T. ) ;
#10736=VERTEX_POINT ( 'NONE', #22427 ) ;
#10737=DIRECTION ( 'NONE',  ( -2.779292025043186357E-18, 1.288349127009862211E-17, -1.000000000000000000 ) ) ;
#10738=CARTESIAN_POINT ( 'NONE',  ( -40.99173213700658636, 9.305078116158226109, 34.54930799450052348 ) ) ;
#10744=CIRCLE ( 'NONE', #31188, 0.09999999999999940881 ) ;
#10745=DIRECTION ( 'NONE',  ( 0.8746197071393926326, -0.4848096202463430537, -8.676864087101709653E-18 ) ) ;
#10751=VECTOR ( 'NONE', #29831, 1000.000000000000114 ) ;
#10757=ORIENTED_EDGE ( 'NONE', *, *, #23846, .T. ) ;
#10759=CARTESIAN_POINT ( 'NONE',  ( -40.59758774925371938, 7.567737757495683226, 38.66054537865625917 ) ) ;
#10760=DIRECTION ( 'NONE',  ( -0.2756373558170082672, 0.9612616959383162296, 0.000000000000000000 ) ) ;
#10764=DIRECTION ( 'NONE',  ( -0.4848096202463429982, -0.8746197071393925215, -9.920727850371698576E-18 ) ) ;
#10767=DIRECTION ( 'NONE',  ( 0.2756373558169974980, -0.9612616959383193382, -1.315048337272770589E-17 ) ) ;
#10772=EDGE_CURVE ( 'NONE', #31154, #15339, #8907, .T. ) ;
#10773=VECTOR ( 'NONE', #21658, 999.9999999999998863 ) ;
#10778=DIRECTION ( 'NONE',  ( -0.9612616959383205595, -0.2756373558169931681, 1.660411357259282445E-16 ) ) ;
#10781=ORIENTED_EDGE ( 'NONE', *, *, #24761, .T. ) ;
#10783=CARTESIAN_POINT ( 'NONE',  ( -42.47434154250543514, 4.196643200812633978, 37.04930799450052348 ) ) ;
#10784=DIRECTION ( 'NONE',  ( 2.779292025043186357E-18, -1.288349127009862211E-17, 1.000000000000000000 ) ) ;
#10788=DIRECTION ( 'NONE',  ( 0.3879443550132459229, 0.6998701428318346851, 0.5997340748914504749 ) ) ;
#10789=ORIENTED_EDGE ( 'NONE', *, *, #22217, .F. ) ;
#10797=CIRCLE ( 'NONE', #29123, 0.1000000000000014905 ) ;
#10800=CARTESIAN_POINT ( 'NONE',  ( -42.50976151518962354, 14.59907569580870224, 35.90717268343339441 ) ) ;
#10803=EDGE_CURVE ( 'NONE', #27773, #20495, #5380, .T. ) ;
#10804=AXIS2_PLACEMENT_3D ( 'NONE', #15653, #23210, #26312 ) ;
#10809=EDGE_LOOP ( 'NONE', ( #10757, #27382 ) ) ;
#10810=CARTESIAN_POINT ( 'NONE',  ( -42.38351229602917414, 14.72295342448899014, 55.13902476097742777 ) ) ;
#10816=DIRECTION ( 'NONE',  ( -1.188208965918165239E-16, -1.880121038077813132E-16, -1.000000000000000000 ) ) ;
#10821=EDGE_CURVE ( 'NONE', #3234, #21817, #2098, .T. ) ;
#10826=VERTEX_POINT ( 'NONE', #27692 ) ;
#10827=ADVANCED_FACE ( 'NONE', ( #15540 ), #18315, .T. ) ;
#10836=ADVANCED_FACE ( 'NONE', ( #13262 ), #17839, .F. ) ;
#10843=CARTESIAN_POINT ( 'NONE',  ( -40.58118912560991731, 7.466305082325866316, 53.91209753419874318 ) ) ;
#10849=ORIENTED_EDGE ( 'NONE', *, *, #21558, .T. ) ;
#10854=ORIENTED_EDGE ( 'NONE', *, *, #13581, .T. ) ;
#10858=AXIS2_PLACEMENT_3D ( 'NONE', #6462, #11381, #15986 ) ;
#10861=EDGE_CURVE ( 'NONE', #21286, #23264, #15119, .T. ) ;
#10863=CARTESIAN_POINT ( 'NONE',  ( -39.50554051497144314, 7.696103224718195968, 32.04930799450052348 ) ) ;
#10864=CARTESIAN_POINT ( 'NONE',  ( -40.02540636251514172, 2.839176264122877047, 58.94930799450051495 ) ) ;
#10866=CARTESIAN_POINT ( 'NONE',  ( -40.63136629056263160, 9.462201496834364178, 38.62930412971698502 ) ) ;
#10868=ORIENTED_EDGE ( 'NONE', *, *, #2770, .F. ) ;
#10869=ORIENTED_EDGE ( 'NONE', *, *, #32245, .T. ) ;
#10877=CARTESIAN_POINT ( 'NONE',  ( -40.18126594841541532, 7.055686659394005744, 39.15537800943240399 ) ) ;
#10887=CARTESIAN_POINT ( 'NONE',  ( -40.86580004447909431, 8.503105189880379555, 34.64930799450051779 ) ) ;
#10888=CARTESIAN_POINT ( 'NONE',  ( -41.61831254958298132, 11.12742816935064738, 37.04930799450052348 ) ) ;
#10889=VERTEX_POINT ( 'NONE', #8004 ) ;
#10890=CARTESIAN_POINT ( 'NONE',  ( -42.63960953052571767, -0.7425051561549622647, 61.99930799450051921 ) ) ;
#10893=DIRECTION ( 'NONE',  ( -2.779292025043186357E-18, 1.288349127009862211E-17, -1.000000000000000000 ) ) ;
#10895=PLANE ( 'NONE',  #30708 ) ;
#10905=EDGE_CURVE ( 'NONE', #6106, #13785, #11268, .T. ) ;
#10906=DIRECTION ( 'NONE',  ( -0.4848096202463431648, -0.8746197071393924105, 0.000000000000000000 ) ) ;
#10908=ORIENTED_EDGE ( 'NONE', *, *, #14046, .F. ) ;
#10914=DIRECTION ( 'NONE',  ( 0.7141240004913198547, -0.3958453973320100738, -0.5773502691896283956 ) ) ;
#10919=VERTEX_POINT ( 'NONE', #31134 ) ;
#10920=CARTESIAN_POINT ( 'NONE',  ( -42.59697395963048194, 14.54042610638008526, 37.04930799450052348 ) ) ;
#10928=DIRECTION ( 'NONE',  ( 2.779292025043186357E-18, -1.288349127009862211E-17, 1.000000000000000000 ) ) ;
#10931=AXIS2_PLACEMENT_3D ( 'NONE', #13515, #26135, #23196 ) ;
#10937=FACE_OUTER_BOUND ( 'NONE', #29151, .T. ) ;
#10940=ORIENTED_EDGE ( 'NONE', *, *, #24108, .F. ) ;
#10955=ORIENTED_EDGE ( 'NONE', *, *, #29120, .T. ) ;
#10956=B_SPLINE_CURVE_WITH_KNOTS ( 'NONE', 3,
 ( #16429, #3961, #1329, #26443, #1014, #21337, #8725, #28590, #8409, #31375 ),
 .UNSPECIFIED., .F., .F.,
 ( 4, 3, 3, 4 ),
 ( 0.000000000000000000, 3.349481945380948403E-05, 6.704430007368558935E-05, 7.824643346661451331E-05 ),
 .UNSPECIFIED. ) ;
#10960=LINE ( 'NONE', #21108, #27945 ) ;
#10971=VECTOR ( 'NONE', #25689, 1000.000000000000000 ) ;
#10972=ORIENTED_EDGE ( 'NONE', *, *, #18961, .T. ) ;
#10974=CARTESIAN_POINT ( 'NONE',  ( -40.46271621608484281, 3.081581074246049212, 58.54930799450051637 ) ) ;
#10980=AXIS2_PLACEMENT_3D ( 'NONE', #30537, #23136, #28229 ) ;
#10984=ADVANCED_FACE ( 'NONE', ( #26028 ), #11561, .T. ) ;
#10993=FACE_OUTER_BOUND ( 'NONE', #1222, .T. ) ;
#10997=DIRECTION ( 'NONE',  ( -0.6184495258776538940, 0.3428121700606627242, 0.7071067811865505703 ) ) ;
#11001=ORIENTED_EDGE ( 'NONE', *, *, #9238, .F. ) ;
#11009=ADVANCED_FACE ( 'NONE', ( #16652 ), #18788, .F. ) ;
#11035=PLANE ( 'NONE',  #18195 ) ;
#11036=CIRCLE ( 'NONE', #1063, 0.09999999999999795164 ) ;
#11042=VECTOR ( 'NONE', #18089, 1000.000000000000114 ) ;
#11047=VERTEX_POINT ( 'NONE', #4030 ) ;
#11056=CARTESIAN_POINT ( 'NONE',  ( -40.08841711228579641, 7.575633567407562552, 53.80788663826320573 ) ) ;
#11058=CIRCLE ( 'NONE', #29402, 0.1000000000000011019 ) ;
#11062=CARTESIAN_POINT ( 'NONE',  ( -41.95414548415062939, 13.78332541096821373, 54.54930799450052348 ) ) ;
#11069=CARTESIAN_POINT ( 'NONE',  ( -40.09211399732166115, 9.667069410243959382, 39.44930799450052206 ) ) ;
#11070=AXIS2_PLACEMENT_3D ( 'NONE', #15060, #2746, #17671 ) ;
#11071=CARTESIAN_POINT ( 'NONE',  ( -40.38239436982999564, 8.630641782992572786, 34.63740864294511823 ) ) ;
#11074=VERTEX_POINT ( 'NONE', #6821 ) ;
#11076=FACE_OUTER_BOUND ( 'NONE', #23500, .T. ) ;
#11077=DIRECTION ( 'NONE',  ( -0.2756373558169897264, 0.9612616959383215587, 0.000000000000000000 ) ) ;
#11090=VECTOR ( 'NONE', #564, 1000.000000000000000 ) ;
#11095=EDGE_CURVE ( 'NONE', #22848, #16786, #651, .T. ) ;
#11101=ORIENTED_EDGE ( 'NONE', *, *, #24199, .T. ) ;
#11102=CARTESIAN_POINT ( 'NONE',  ( -43.38408989745150990, 1.111547985471239341, 60.54930799450051637 ) ) ;
#11105=SPHERICAL_SURFACE ( 'NONE', #41, 0.1000000000000000056 ) ;
#11106=EDGE_LOOP ( 'NONE', ( #25024, #16389, #13967, #14685 ) ) ;
#11109=CARTESIAN_POINT ( 'NONE',  ( -40.46271621608484281, 3.081581074246050544, 61.94930799450052206 ) ) ;
#11113=CARTESIAN_POINT ( 'NONE',  ( -40.60722745863126448, 9.415333058485023443, 35.49072935073782986 ) ) ;
#11119=CARTESIAN_POINT ( 'NONE',  ( -40.57420052961218460, 7.102220148651144704, 35.23168232079561335 ) ) ;
#11121=CARTESIAN_POINT ( 'NONE',  ( -41.61831254958298132, 11.12742816935064916, 35.90717268343339441 ) ) ;
#11126=PRODUCT_DEFINITION_CONTEXT ( 'detailed design', #3625, 'design' ) ;
#11132=EDGE_CURVE ( 'NONE', #8819, #30210, #6835, .T. ) ;
#11147=CARTESIAN_POINT ( 'NONE',  ( -40.66259927863510626, 6.843847033175615380, 39.31544081796293710 ) ) ;
#11151=DIRECTION ( 'NONE',  ( -7.588956326749211550E-18, 4.206627182996911684E-18, -1.000000000000000000 ) ) ;
#11152=ORIENTED_EDGE ( 'NONE', *, *, #3337, .T. ) ;
#11153=PLANE ( 'NONE',  #14587 ) ;
#11154=CYLINDRICAL_SURFACE ( 'NONE', #10443, 0.1000000000000018235 ) ;
#11160=CARTESIAN_POINT ( 'NONE',  ( -40.71976880025163581, 7.963440923891331735, 57.04930799450051637 ) ) ;
#11162=ORIENTED_EDGE ( 'NONE', *, *, #21700, .F. ) ;
#11166=EDGE_CURVE ( 'NONE', #19917, #3984, #6272, .T. ) ;
#11168=AXIS2_PLACEMENT_3D ( 'NONE', #27991, #22564, #22736 ) ;
#11170=ADVANCED_FACE ( 'NONE', ( #26457 ), #3644, .T. ) ;
#11172=CARTESIAN_POINT ( 'NONE',  ( -40.06561427811386267, 7.496110634155836117, 60.54930799450051637 ) ) ;
#11174=EDGE_LOOP ( 'NONE', ( #15901, #15690, #15323, #16225 ) ) ;
#11178=LINE ( 'NONE', #16408, #3521 ) ;
#11183=CARTESIAN_POINT ( 'NONE',  ( -40.68127404237834099, 6.801539337588502931, 34.61638395550082237 ) ) ;
#11187=CARTESIAN_POINT ( 'NONE',  ( -40.02540636251513462, 2.839176264122873050, 35.04930799450051637 ) ) ;
#11192=FACE_OUTER_BOUND ( 'NONE', #27957, .T. ) ;
#11195=CARTESIAN_POINT ( 'NONE',  ( -40.63136629056263160, 9.462201496834364178, 34.66931185928405057 ) ) ;
#11199=CARTESIAN_POINT ( 'NONE',  ( -40.75848109938849717, 9.580021662090986823, 38.54930799450052348 ) ) ;
#11200=VERTEX_POINT ( 'NONE', #13671 ) ;
#11202=EDGE_CURVE ( 'NONE', #30206, #5667, #26514, .T. ) ;
#11205=DIRECTION ( 'NONE',  ( 0.8746197071393858602, -0.4848096202463547666, 0.000000000000000000 ) ) ;
#11208=VECTOR ( 'NONE', #1824, 1000.000000000000000 ) ;
#11209=CARTESIAN_POINT ( 'NONE',  ( -40.61178118339597631, 9.038025460530262123, 57.95249952744806166 ) ) ;
#11212=ORIENTED_EDGE ( 'NONE', *, *, #27096, .F. ) ;
#11216=EDGE_CURVE ( 'NONE', #5139, #7595, #2643, .T. ) ;
#11221=DIRECTION ( 'NONE',  ( 0.2250569586005335410, -0.7848668881104262640, -0.5773502691896259531 ) ) ;
#11222=EDGE_CURVE ( 'NONE', #9700, #13764, #29922, .T. ) ;
#11223=CARTESIAN_POINT ( 'NONE',  ( -40.11688989807090167, 6.803825020423235337, 34.64825762772819218 ) ) ;
#11229=CARTESIAN_POINT ( 'NONE',  ( -40.11729073372970333, 6.802967823440400075, 34.64930799450051779 ) ) ;
#11233=SPHERICAL_SURFACE ( 'NONE', #6256, 0.1000000000000000056 ) ;
#11235=ADVANCED_FACE ( 'NONE', ( #21346 ), #19051, .T. ) ;
#11236=CARTESIAN_POINT ( 'NONE',  ( -42.37913764077812573, 15.23192269303852697, 38.44930799450052916 ) ) ;
#11239=ORIENTED_EDGE ( 'NONE', *, *, #14763, .F. ) ;
#11242=EDGE_LOOP ( 'NONE', ( #4946, #5025, #5079 ) ) ;
#11245=CYLINDRICAL_SURFACE ( 'NONE', #2405, 0.1000000000000007272 ) ;
#11252=DIRECTION ( 'NONE',  ( 0.7141240004913198547, -0.3958453973320100738, 0.5773502691896283956 ) ) ;
#11263=DIRECTION ( 'NONE',  ( 2.779292025043186357E-18, -1.288349127009862211E-17, 1.000000000000000000 ) ) ;
#11268=LINE ( 'NONE', #28658, #18929 ) ;
#11272=CARTESIAN_POINT ( 'NONE',  ( -40.56500720768330837, 7.149487417330789185, 35.17537323039149300 ) ) ;
#11273=EDGE_LOOP ( 'NONE', ( #17530, #29469, #23046, #19047 ) ) ;
#11277=EDGE_LOOP ( 'NONE', ( #1903, #21909 ) ) ;
#11288=CARTESIAN_POINT ( 'NONE',  ( -42.34864001897649644, 13.69590355195401621, 59.50603524064797512 ) ) ;
#11293=CIRCLE ( 'NONE', #29647, 1.899999999999999023 ) ;
#11305=CARTESIAN_POINT ( 'NONE',  ( -43.72819403793993587, 1.315833819094413659, 34.64930799450052490 ) ) ;
#11306=CARTESIAN_POINT ( 'NONE',  ( -40.70484894842233103, 8.274204744976163539, 59.54930799450050927 ) ) ;
#11309=FACE_BOUND ( 'NONE', #12704, .T. ) ;
#11311=ADVANCED_FACE ( 'NONE', ( #32452 ), #12107, .F. ) ;
#11316=VERTEX_POINT ( 'NONE', #9802 ) ;
#11324=VERTEX_POINT ( 'NONE', #20284 ) ;
#11332=CARTESIAN_POINT ( 'NONE',  ( -40.04869510400517640, 6.988917179838707305, 39.04796398176969063 ) ) ;
#11334=DIRECTION ( 'NONE',  ( -0.8746197071393840838, 0.4848096202463581528, 0.000000000000000000 ) ) ;
#11335=ORIENTED_EDGE ( 'NONE', *, *, #10545, .F. ) ;
#11338=CARTESIAN_POINT ( 'NONE',  ( -39.58809650894544774, 2.596771453999702661, 47.04930799450051637 ) ) ;
#11343=CARTESIAN_POINT ( 'NONE',  ( -40.02540636251514172, 2.839176264122877047, 57.04930799450051637 ) ) ;
#11350=ORIENTED_EDGE ( 'NONE', *, *, #9121, .F. ) ;
#11355=LINE ( 'NONE', #31380, #11208 ) ;
#11356=EDGE_LOOP ( 'NONE', ( #30124, #21106, #27786, #20033, #29315, #5393 ) ) ;
#11363=FACE_OUTER_BOUND ( 'NONE', #29848, .T. ) ;
#11367=AXIS2_PLACEMENT_3D ( 'NONE', #30226, #30383, #184 ) ;
#11369=CARTESIAN_POINT ( 'NONE',  ( -40.52064652407317169, 7.631814549704933448, 53.92245119299456491 ) ) ;
#11376=CARTESIAN_POINT ( 'NONE',  ( -40.38150472626228549, 8.621068314769347651, 34.62702073480610210 ) ) ;
#11381=DIRECTION ( 'NONE',  ( 0.4848096202463430537, 0.8746197071393926326, 9.920727850371700117E-18 ) ) ;
#11384=ORIENTED_EDGE ( 'NONE', *, *, #24383, .F. ) ;
#11388=FACE_OUTER_BOUND ( 'NONE', #14885, .T. ) ;
#11390=ORIENTED_EDGE ( 'NONE', *, *, #22971, .F. ) ;
#11393=ORIENTED_EDGE ( 'NONE', *, *, #23233, .T. ) ;
#11401=ORIENTED_EDGE ( 'NONE', *, *, #2599, .F. ) ;
#11413=ORIENTED_EDGE ( 'NONE', *, *, #12398, .T. ) ;
#11421=DIRECTION ( 'NONE',  ( 0.4848096202463506588, 0.8746197071393884137, 9.920727850371624621E-18 ) ) ;
#11429=VECTOR ( 'NONE', #32283, 1000.000000000000000 ) ;
#11443=DIRECTION ( 'NONE',  ( 0.2756373558169974980, -0.9612616959383193382, 9.694974607321218218E-33 ) ) ;
#11448=AXIS2_PLACEMENT_3D ( 'NONE', #29287, #1876, #16161 ) ;
#11452=CARTESIAN_POINT ( 'NONE',  ( -40.56083369918798098, 7.405617721157757849, 38.79123571389602887 ) ) ;
#11453=CARTESIAN_POINT ( 'NONE',  ( -40.69114442294520728, 6.794816359673525596, 39.38644499583401881 ) ) ;
#11455=CIRCLE ( 'NONE', #1493, 1.300000000000002487 ) ;
#11458=DIRECTION ( 'NONE',  ( 0.000000000000000000, 0.000000000000000000, -1.000000000000000000 ) ) ;
#11464=AXIS2_PLACEMENT_3D ( 'NONE', #14501, #32225, #19571 ) ;
#11465=FACE_OUTER_BOUND ( 'NONE', #5480, .T. ) ;
#11467=ORIENTED_EDGE ( 'NONE', *, *, #25356, .T. ) ;
#11473=EDGE_CURVE ( 'NONE', #4508, #7574, #29788, .T. ) ;
#11476=ADVANCED_FACE ( 'NONE', ( #10937 ), #11105, .T. ) ;
#11492=CARTESIAN_POINT ( 'NONE',  ( -41.23493495844309109, 10.15322714841875040, 37.04930799450052348 ) ) ;
#11504=DIRECTION ( 'NONE',  ( -0.8746197071393810862, 0.4848096202463637039, 8.676864087101942305E-18 ) ) ;
#11506=FACE_BOUND ( 'NONE', #18956, .T. ) ;
#11515=FACE_OUTER_BOUND ( 'NONE', #30343, .T. ) ;
#11516=CARTESIAN_POINT ( 'NONE',  ( -40.68422973805265030, 6.807290781432338456, 34.77612644482307758 ) ) ;
#11527=EDGE_CURVE ( 'NONE', #14804, #8738, #5842, .T. ) ;
#11529=VECTOR ( 'NONE', #24462, 1000.000000000000114 ) ;
#11530=DIRECTION ( 'NONE',  ( 0.4848096202463424986, 0.8746197071393928546, -2.220446049250312834E-16 ) ) ;
#11533=DIRECTION ( 'NONE',  ( -0.1949050434465282866, 0.6797146636928672603, -0.7071067811865470176 ) ) ;
#11534=AXIS2_PLACEMENT_3D ( 'NONE', #28767, #30760, #18580 ) ;
#11544=ORIENTED_EDGE ( 'NONE', *, *, #3963, .F. ) ;
#11545=DIRECTION ( 'NONE',  ( 0.9612616959383221138, 0.2756373558169876170, 0.000000000000000000 ) ) ;
#11546=CARTESIAN_POINT ( 'NONE',  ( -40.19913497620438392, 7.013551051776435230, 39.22537497467693157 ) ) ;
#11549=EDGE_LOOP ( 'NONE', ( #3417, #16301, #19567, #14155, #26636, #25473, #14173, #4535, #29485, #23469 ) ) ;
#11550=DIRECTION ( 'NONE',  ( 0.1949050434465275650, -0.6797146636928697028, 0.7071067811865449082 ) ) ;
#11553=DIRECTION ( 'NONE',  ( -4.252959262497663712E-16, 2.543118322573790544E-15, 1.000000000000000000 ) ) ;
#11558=CIRCLE ( 'NONE', #14192, 0.09999999999999753530 ) ;
#11561=TOROIDAL_SURFACE ( 'NONE', #15761, 1.142135311067127068, 0.1000000000000000056 ) ;
#11567=( BOUNDED_SURFACE ( )  B_SPLINE_SURFACE ( 3, 2, ( 
 ( #26359, #28827, #18484 ),
 ( #16343, #31140, #13739 ),
 ( #614, #3877, #26195 ),
 ( #23736, #23419, #20948 ),
 ( #30979, #11272, #11119 ),
 ( #6026, #20792, #16027 ),
 ( #1244, #21103, #21264 ),
 ( #18320, #23096, #8794 ),
 ( #18792, #8489, #31294 ),
 ( #10641, #20634, #30656 ) ),
 .UNSPECIFIED., .F., .F., .F. ) 
 B_SPLINE_SURFACE_WITH_KNOTS ( ( 4, 2, 2, 2, 4 ),
 ( 3, 3 ),
 ( -2.222614453595284090E-18, 0.0003347409949957051148, 0.0006694819899914123979, 0.001004222984987119573, 0.001338963979982826964 ),
 ( 0.000000000000000000, 1.000000000000000000 ),
 .UNSPECIFIED. ) 
 GEOMETRIC_REPRESENTATION_ITEM ( )  RATIONAL_B_SPLINE_SURFACE ( (
 ( 1.000000000000000000, 0.7071067811865465735, 1.000000000000000000),
 ( 1.000000000000000000, 0.7102524952755833176, 1.000000000000000000),
 ( 1.000000000000000000, 0.7282169120226342773, 1.000000000000000000),
 ( 1.000000000000000000, 0.7754022836010627806, 1.000000000000000000),
 ( 1.000000000000000000, 0.8043059223109642053, 1.000000000000000000),
 ( 1.000000000000000000, 0.8571167854607034675, 1.000000000000000000),
 ( 1.000000000000000000, 0.8816198077927471788, 1.000000000000000000),
 ( 1.000000000000000000, 0.9175117844836407910, 1.000000000000000000),
 ( 1.000000000000000000, 0.9295466150070802458, 1.000000000000000000),
 ( 1.000000000000000000, 0.9308844615756591834, 1.000000000000000000) ) ) 
 REPRESENTATION_ITEM ( '' )  SURFACE ( )  );
#11577=DIRECTION ( 'NONE',  ( -0.4848096202463430537, -0.8746197071393926326, -9.920727850371700117E-18 ) ) ;
#11579=DIRECTION ( 'NONE',  ( 0.8746197071393926326, -0.4848096202463430537, -8.676864087101709653E-18 ) ) ;
#11582=FACE_OUTER_BOUND ( 'NONE', #32079, .T. ) ;
#11583=ORIENTED_EDGE ( 'NONE', *, *, #9617, .T. ) ;
#11594=AXIS2_PLACEMENT_3D ( 'NONE', #28813, #31762, #18625 ) ;
#11599=ORIENTED_EDGE ( 'NONE', *, *, #20529, .F. ) ;
#11600=EDGE_CURVE ( 'NONE', #13675, #3287, #7922, .T. ) ;
#11603=ORIENTED_EDGE ( 'NONE', *, *, #15890, .T. ) ;
#11606=CARTESIAN_POINT ( 'NONE',  ( -42.73182147790732444, -0.8057266458565844891, 32.04930799450052348 ) ) ;
#11607=EDGE_CURVE ( 'NONE', #27622, #607, #11058, .T. ) ;
#11611=FACE_OUTER_BOUND ( 'NONE', #25190, .T. ) ;
#11623=CARTESIAN_POINT ( 'NONE',  ( -40.68293647075795860, 6.808040729367310639, 39.52524033956975558 ) ) ;
#11625=DIRECTION ( 'NONE',  ( -1.188208965918165239E-16, -1.880121038077813132E-16, -1.000000000000000000 ) ) ;
#11627=DIRECTION ( 'NONE',  ( -1.188208965918165239E-16, -1.880121038077813132E-16, -1.000000000000000000 ) ) ;
#11630=ORIENTED_EDGE ( 'NONE', *, *, #32133, .T. ) ;
#11632=DIRECTION ( 'NONE',  ( -0.8746197071393925215, 0.4848096202463429982, 1.121857559391816958E-19 ) ) ;
#11637=CARTESIAN_POINT ( 'NONE',  ( -43.86882709718853590, -0.1754741395363378920, 61.94930799450052206 ) ) ;
#11638=AXIS2_PLACEMENT_3D ( 'NONE', #9303, #19300, #16846 ) ;
#11640=CARTESIAN_POINT ( 'NONE',  ( -42.38687957179150345, 4.148162238788003719, 57.04930799450051637 ) ) ;
#11642=VECTOR ( 'NONE', #27620, 1000.000000000000000 ) ;
#11646=EDGE_CURVE ( 'NONE', #21033, #31848, #26344, .T. ) ;
#11647=EDGE_CURVE ( 'NONE', #2889, #6349, #15245, .T. ) ;
#11648=EDGE_CURVE ( 'NONE', #21311, #24691, #21572, .T. ) ;
#11649=ORIENTED_EDGE ( 'NONE', *, *, #21558, .F. ) ;
#11650=CIRCLE ( 'NONE', #24740, 0.1000000000000014905 ) ;
#11651=ORIENTED_EDGE ( 'NONE', *, *, #4813, .F. ) ;
#11656=VECTOR ( 'NONE', #22462, 1000.000000000000114 ) ;
#11657=EDGE_LOOP ( 'NONE', ( #18645, #20261, #3171, #3305, #11101 ) ) ;
#11659=DIRECTION ( 'NONE',  ( -0.6184495258776564475, 0.3428121700606708844, 0.7071067811865443531 ) ) ;
#11663=ORIENTED_EDGE ( 'NONE', *, *, #3614, .T. ) ;
#11667=ADVANCED_FACE ( 'NONE', ( #19266 ), #6342, .F. ) ;
#11674=CARTESIAN_POINT ( 'NONE',  ( -39.85048242108726413, 2.742214340073605872, 47.04930799450051637 ) ) ;
#11684=AXIS2_PLACEMENT_3D ( 'NONE', #32132, #19148, #29510 ) ;
#11687=ORIENTED_EDGE ( 'NONE', *, *, #2663, .F. ) ;
#11691=DIRECTION ( 'NONE',  ( 0.000000000000000000, 0.000000000000000000, -1.000000000000000000 ) ) ;
#11695=CARTESIAN_POINT ( 'NONE',  ( -40.99628586177130529, 8.927770518203464789, 57.04930799450051637 ) ) ;
#11696=AXIS2_PLACEMENT_3D ( 'NONE', #23916, #11774, #4382 ) ;
#11697=DIRECTION ( 'NONE',  ( 0.9612616959383205595, 0.2756373558169931681, -1.660411357259282445E-16 ) ) ;
#11711=VERTEX_POINT ( 'NONE', #20093 ) ;
#11721=VERTEX_POINT ( 'NONE', #7138 ) ;
#11730=CYLINDRICAL_SURFACE ( 'NONE', #5847, 0.1000000000000020595 ) ;
#11731=LINE ( 'NONE', #19256, #1362 ) ;
#11740=ORIENTED_EDGE ( 'NONE', *, *, #776, .T. ) ;
#11741=CARTESIAN_POINT ( 'NONE',  ( -40.76967387488526384, 8.530668925462078889, 39.44930799450052206 ) ) ;
#11751=CARTESIAN_POINT ( 'NONE',  ( -40.22853490217747208, 6.951940700334876766, 34.71623747574528807 ) ) ;
#11754=DIRECTION ( 'NONE',  ( -0.6797146636928672603, -0.1949050434465268711, 0.7071067811865474617 ) ) ;
#11756=EDGE_CURVE ( 'NONE', #12114, #23633, #31532, .T. ) ;
#11760=ORIENTED_EDGE ( 'NONE', *, *, #21210, .T. ) ;
#11761=EDGE_CURVE ( 'NONE', #9365, #5667, #15176, .T. ) ;
#11766=VECTOR ( 'NONE', #19709, 999.9999999999998863 ) ;
#11767=EDGE_CURVE ( 'NONE', #13582, #17141, #4255, .T. ) ;
#11768=DIRECTION ( 'NONE',  ( 0.000000000000000000, 1.000000000000000000, 0.000000000000000000 ) ) ;
#11771=CARTESIAN_POINT ( 'NONE',  ( -42.36691375901575185, 13.72999064396537250, 59.48380644099231773 ) ) ;
#11774=DIRECTION ( 'NONE',  ( 0.8746197071393926326, -0.4848096202463430537, -8.676864087101709653E-18 ) ) ;
#11778=DIRECTION ( 'NONE',  ( -0.9612616959383205595, -0.2756373558169932236, 1.660411357259282445E-16 ) ) ;
#11780=SPHERICAL_SURFACE ( 'NONE', #2236, 0.1000000000000000056 ) ;
#11784=DIRECTION ( 'NONE',  ( 1.188208965918165239E-16, 1.880121038077813132E-16, 1.000000000000000000 ) ) ;
#11785=CARTESIAN_POINT ( 'NONE',  ( -40.47970302497625994, 7.463434137431150361, 60.54930799450051637 ) ) ;
#11792=VECTOR ( 'NONE', #8077, 1000.000000000000114 ) ;
#11804=ORIENTED_EDGE ( 'NONE', *, *, #25320, .F. ) ;
#11807=EDGE_CURVE ( 'NONE', #1546, #2479, #24699, .T. ) ;
#11815=AXIS2_PLACEMENT_3D ( 'NONE', #6326, #26668, #32262 ) ;
#11820=ORIENTED_EDGE ( 'NONE', *, *, #13860, .F. ) ;
#11824=EDGE_CURVE ( 'NONE', #16387, #17225, #13197, .T. ) ;
#11825=ORIENTED_EDGE ( 'NONE', *, *, #20525, .T. ) ;
#11826=EDGE_LOOP ( 'NONE', ( #8423, #7935, #22448, #31774 ) ) ;
#11827=EDGE_CURVE ( 'NONE', #4768, #22442, #26785, .T. ) ;
#11833=ORIENTED_EDGE ( 'NONE', *, *, #5537, .F. ) ;
#11835=DIRECTION ( 'NONE',  ( 0.9612616959383206705, 0.2756373558169926130, 8.795445018804289444E-19 ) ) ;
#11839=FACE_OUTER_BOUND ( 'NONE', #5562, .T. ) ;
#11853=ORIENTED_EDGE ( 'NONE', *, *, #28914, .F. ) ;
#11859=ADVANCED_FACE ( 'NONE', ( #5334, #13213 ), #25665, .T. ) ;
#11862=DIRECTION ( 'NONE',  ( 0.1949050434465268156, -0.6797146636928675933, -0.7071067811865470176 ) ) ;
#11872=CARTESIAN_POINT ( 'NONE',  ( -40.18454328187963398, 7.548069831825863218, 60.44930799450051495 ) ) ;
#11878=PLANE ( 'NONE',  #2606 ) ;
#11892=B_SPLINE_CURVE_WITH_KNOTS ( 'NONE', 3,
 ( #18299, #8467, #31276, #8627 ),
 .UNSPECIFIED., .F., .F.,
 ( 4, 4 ),
 ( 0.000000000000000000, 0.0001058398962549312607 ),
 .UNSPECIFIED. ) ;
#11898=CARTESIAN_POINT ( 'NONE',  ( -41.13768170161382898, 11.26524684725914227, 37.04930799450052348 ) ) ;
#11907=ORIENTED_EDGE ( 'NONE', *, *, #1662, .T. ) ;
#11908=CARTESIAN_POINT ( 'NONE',  ( -38.41701585771487260, 6.978388747684010518, 32.04930799450052348 ) ) ;
#11913=ORIENTED_EDGE ( 'NONE', *, *, #8451, .T. ) ;
#11919=AXIS2_PLACEMENT_3D ( 'NONE', #17440, #27462, #4977 ) ;
#11922=DIRECTION ( 'NONE',  ( -0.2756373558169926130, 0.9612616959383207815, -2.065119226596364453E-17 ) ) ;
#11932=DIRECTION ( 'NONE',  ( 2.779292025043186357E-18, -1.288349127009862057E-17, 1.000000000000000000 ) ) ;
#11933=EDGE_CURVE ( 'NONE', #17141, #4744, #600, .T. ) ;
#11942=CARTESIAN_POINT ( 'NONE',  ( -41.07560527903737579, 9.385057823277964673, 35.44930799450052206 ) ) ;
#11945=FACE_OUTER_BOUND ( 'NONE', #17501, .T. ) ;
#11949=ORIENTED_EDGE ( 'NONE', *, *, #28426, .F. ) ;
#11963=AXIS2_PLACEMENT_3D ( 'NONE', #3485, #1184, #23514 ) ;
#11965=ADVANCED_FACE ( 'NONE', ( #15819 ), #28769, .T. ) ;
#11973=AXIS2_PLACEMENT_3D ( 'NONE', #7965, #15342, #30766 ) ;
#11977=CIRCLE ( 'NONE', #18769, 1.500000000000001332 ) ;
#11982=EDGE_LOOP ( 'NONE', ( #875, #29753, #25300, #18963 ) ) ;
#11983=DIRECTION ( 'NONE',  ( 0.6184495258776571136, -0.3428121700606572286, -0.7071067811865505703 ) ) ;
#11984=EDGE_LOOP ( 'NONE', ( #27240, #23490, #5993, #15946, #21376 ) ) ;
#11989=FACE_OUTER_BOUND ( 'NONE', #13294, .T. ) ;
#11994=PLANE ( 'NONE',  #5189 ) ;
#11996=ORIENTED_EDGE ( 'NONE', *, *, #26298, .T. ) ;
#11999=ORIENTED_EDGE ( 'NONE', *, *, #1745, .T. ) ;
#12000=PLANE ( 'NONE',  #19950 ) ;
#12004=FACE_OUTER_BOUND ( 'NONE', #12873, .T. ) ;
#12005=VECTOR ( 'NONE', #18707, 1000.000000000000000 ) ;
#12007=AXIS2_PLACEMENT_3D ( 'NONE', #22287, #16871, #12907 ) ;
#12008=ORIENTED_EDGE ( 'NONE', *, *, #28676, .T. ) ;
#12009=DIRECTION ( 'NONE',  ( -0.2250569586005261857, 0.7848668881104258199, 0.5773502691896292838 ) ) ;
#12010=CARTESIAN_POINT ( 'NONE',  ( -41.93344242462055149, 13.82826554927148166, 54.56265170360538264 ) ) ;
#12018=CIRCLE ( 'NONE', #30375, 0.9000000000000011324 ) ;
#12024=CARTESIAN_POINT ( 'NONE',  ( -42.68872152249107188, 16.18454730271123054, 55.97778115698459089 ) ) ;
#12027=CARTESIAN_POINT ( 'NONE',  ( -40.43834990939047458, 8.528791397241549888, 34.55055826194722357 ) ) ;
#12031=ORIENTED_EDGE ( 'NONE', *, *, #22578, .F. ) ;
#12034=CARTESIAN_POINT ( 'NONE',  ( -40.59758774925371938, 7.567737757495682338, 35.43807061034478778 ) ) ;
#12039=CARTESIAN_POINT ( 'NONE',  ( -40.02540636251514172, 2.839176264122877047, 58.54930799450051637 ) ) ;
#12043=CARTESIAN_POINT ( 'NONE',  ( -41.94956971822180947, 3.905757428664828890, 47.04930799450051637 ) ) ;
#12044=ORIENTED_EDGE ( 'NONE', *, *, #5499, .F. ) ;
#12046=EDGE_LOOP ( 'NONE', ( #24626, #17124, #26874, #15315, #29984 ) ) ;
#12048=AXIS2_PLACEMENT_3D ( 'NONE', #25186, #2212, #5008 ) ;
#12054=VECTOR ( 'NONE', #7447, 1000.000000000000114 ) ;
#12072=DIRECTION ( 'NONE',  ( 0.1949050434465251225, -0.6797146636928670382, 0.7071067811865481278 ) ) ;
#12074=DIRECTION ( 'NONE',  ( 0.8746197071393926326, -0.4848096202463430537, -8.676864087101709653E-18 ) ) ;
#12076=CARTESIAN_POINT ( 'NONE',  ( -40.22836982583548604, 6.952244300597145710, 34.71735136656046450 ) ) ;
#12079=CARTESIAN_POINT ( 'NONE',  ( -40.06891218940336330, 7.538004613239514207, 35.29832907986742185 ) ) ;
#12082=VERTEX_POINT ( 'NONE', #19564 ) ;
#12084=VECTOR ( 'NONE', #18510, 1000.000000000000114 ) ;
#12085=CIRCLE ( 'NONE', #3157, 0.09999999999999795164 ) ;
#12087=DIRECTION ( 'NONE',  ( -0.8746197071393858602, 0.4848096202463547666, 0.000000000000000000 ) ) ;
#12095=ORIENTED_EDGE ( 'NONE', *, *, #23018, .T. ) ;
#12101=DIRECTION ( 'NONE',  ( -0.1949050434465267878, 0.6797146636928665941, -0.7071067811865480168 ) ) ;
#12107=CYLINDRICAL_SURFACE ( 'NONE', #29366, 0.1000000000000006301 ) ;
#12108=ORIENTED_EDGE ( 'NONE', *, *, #17453, .T. ) ;
#12109=CARTESIAN_POINT ( 'NONE',  ( -39.58809650894544774, 2.596771453999702661, 48.54930799450051637 ) ) ;
#12113=AXIS2_PLACEMENT_3D ( 'NONE', #18748, #3668, #21215 ) ;
#12114=VERTEX_POINT ( 'NONE', #17262 ) ;
#12121=CYLINDRICAL_SURFACE ( 'NONE', #24155, 0.1000000000000008243 ) ;
#12122=DIRECTION ( 'NONE',  ( 0.1949050434465265935, -0.6797146636928685925, -0.7071067811865462405 ) ) ;
#12125=DIRECTION ( 'NONE',  ( 0.9612616959383207815, 0.2756373558169926685, 8.795445018804289444E-19 ) ) ;
#12128=CARTESIAN_POINT ( 'NONE',  ( -37.49824857498671093, 12.70128680827697387, 57.04930799450051637 ) ) ;
#12132=CARTESIAN_POINT ( 'NONE',  ( -42.30123736278718383, 13.66041317296246937, 54.56265170360538264 ) ) ;
#12133=EDGE_CURVE ( 'NONE', #21157, #9796, #14980, .T. ) ;
#12140=DIRECTION ( 'NONE',  ( -0.9612616959383221138, -0.2756373558169876170, 0.000000000000000000 ) ) ;
#12152=MECHANICAL_DESIGN_GEOMETRIC_PRESENTATION_REPRESENTATION('',(#25252),#30508);
#12153=DIRECTION ( 'NONE',  ( 0.6797146636928683705, 0.1949050434465285919, 0.7071067811865459074 ) ) ;
#12154=CARTESIAN_POINT ( 'NONE',  ( -40.68422973805265030, 6.807290781432338456, 34.77612644482307758 ) ) ;
#12158=ORIENTED_EDGE ( 'NONE', *, *, #14005, .T. ) ;
#12161=DIRECTION ( 'NONE',  ( -0.9612616959383183390, -0.2756373558170014948, -8.795445018805493151E-19 ) ) ;
#12162=LINE ( 'NONE', #22155, #18803 ) ;
#12163=ORIENTED_EDGE ( 'NONE', *, *, #12814, .F. ) ;
#12169=FACE_OUTER_BOUND ( 'NONE', #26764, .T. ) ;
#12170=EDGE_CURVE ( 'NONE', #27545, #12894, #24825, .T. ) ;
#12171=EDGE_CURVE ( 'NONE', #2697, #2431, #4477, .T. ) ;
#12177=AXIS2_PLACEMENT_3D ( 'NONE', #1447, #18836, #23621 ) ;
#12183=CARTESIAN_POINT ( 'NONE',  ( -40.02540636251514172, 2.839176264122877047, 57.04930799450051637 ) ) ;
#12186=CARTESIAN_POINT ( 'NONE',  ( -40.11286833322908052, 2.887657226147511302, 55.74930799450051211 ) ) ;
#12190=AXIS2_PLACEMENT_3D ( 'NONE', #5772, #26273, #3621 ) ;
#12198=EDGE_CURVE ( 'NONE', #25211, #21636, #20767, .T. ) ;
#12203=ORIENTED_EDGE ( 'NONE', *, *, #13246, .T. ) ;
#12206=DIRECTION ( 'NONE',  ( -0.9612616959383205595, -0.2756373558169931681, 1.660411357259282445E-16 ) ) ;
#12210=CARTESIAN_POINT ( 'NONE',  ( -40.02540636251513462, 2.839176264122873050, 37.04930799450052348 ) ) ;
#12216=EDGE_CURVE ( 'NONE', #28526, #14460, #2669, .T. ) ;
#12228=EDGE_LOOP ( 'NONE', ( #7559, #27407, #9036, #1470 ) ) ;
#12234=ORIENTED_EDGE ( 'NONE', *, *, #10244, .F. ) ;
#12235=EDGE_CURVE ( 'NONE', #19419, #7551, #16801, .T. ) ;
#12236=DIRECTION ( 'NONE',  ( 0.4848096202463673676, 0.8746197071393789768, 0.000000000000000000 ) ) ;
#12243=DIRECTION ( 'NONE',  ( -2.946248497964555786E-19, -3.001156285468303092E-19, -1.000000000000000000 ) ) ;
#12248=ORIENTED_EDGE ( 'NONE', *, *, #26162, .T. ) ;
#12254=( BOUNDED_CURVE ( )  B_SPLINE_CURVE ( 3, ( #29, #27441, #15131, #4957 ),
 .UNSPECIFIED., .F., .F. ) 
 B_SPLINE_CURVE_WITH_KNOTS ( ( 4, 4 ),
 ( 2.992702705980254230, 4.414609085165686508 ),
 .UNSPECIFIED. ) 
 CURVE ( )  GEOMETRIC_REPRESENTATION_ITEM ( )  RATIONAL_B_SPLINE_CURVE ( ( 1.000000000000000000, 0.8384934736035498659, 0.8384934736035498659, 1.000000000000000000 ) ) 
 REPRESENTATION_ITEM ( '' )  );
#12261=DIRECTION ( 'NONE',  ( 0.000000000000000000, 0.000000000000000000, 1.000000000000000000 ) ) ;
#12262=EDGE_CURVE ( 'NONE', #3764, #6409, #30983, .T. ) ;
#12272=ORIENTED_EDGE ( 'NONE', *, *, #9759, .T. ) ;
#12276=VERTEX_POINT ( 'NONE', #28104 ) ;
#12278=CARTESIAN_POINT ( 'NONE',  ( -43.64647580959332629, 1.256990871545142774, 60.44930799450051495 ) ) ;
#12283=CARTESIAN_POINT ( 'NONE',  ( -41.94956971822180947, 3.905757428664828890, 47.04930799450051637 ) ) ;
#12284=CARTESIAN_POINT ( 'NONE',  ( -40.66586793973302605, 8.138261812237590931, 54.59072935073782418 ) ) ;
#12285=ORIENTED_EDGE ( 'NONE', *, *, #16232, .F. ) ;
#12290=CARTESIAN_POINT ( 'NONE',  ( -40.05987053574653345, 7.506472619680472746, 38.44930799450052916 ) ) ;
#12291=VERTEX_POINT ( 'NONE', #20701 ) ;
#12296=ORIENTED_EDGE ( 'NONE', *, *, #21810, .F. ) ;
#12297=EDGE_LOOP ( 'NONE', ( #2065, #3610, #8650, #31467 ) ) ;
#12305=CIRCLE ( 'NONE', #20666, 1.300000000000002487 ) ;
#12311=CIRCLE ( 'NONE', #30148, 0.09999999999999714673 ) ;
#12315=AXIS2_PLACEMENT_3D ( 'NONE', #21117, #25740, #944 ) ;
#12316=CARTESIAN_POINT ( 'NONE',  ( -40.90015969217747482, 8.955334253785162346, 57.95249952744806166 ) ) ;
#12327=CARTESIAN_POINT ( 'NONE',  ( -40.98031486389898248, 9.265261353013489298, 39.54930799450052348 ) ) ;
#12334=DIRECTION ( 'NONE',  ( -0.1299938060159217812, 0.9915148059396262648, 1.313546309486176444E-17 ) ) ;
#12342=FACE_OUTER_BOUND ( 'NONE', #25053, .T. ) ;
#12360=CARTESIAN_POINT ( 'NONE',  ( -40.50410981870283678, 7.604537000166496696, 35.33853321918559232 ) ) ;
#12364=DIRECTION ( 'NONE',  ( 0.000000000000000000, 0.000000000000000000, -1.000000000000000000 ) ) ;
#12367=DIRECTION ( 'NONE',  ( 0.2756373558169954441, -0.9612616959383198934, 1.479773560108263451E-16 ) ) ;
#12368=CARTESIAN_POINT ( 'NONE',  ( -40.16409007829387434, 6.927803014773068035, 34.54930799450055190 ) ) ;
#12371=ORIENTED_EDGE ( 'NONE', *, *, #10469, .F. ) ;
#12373=LINE ( 'NONE', #17765, #11642 ) ;
#12374=DIRECTION ( 'NONE',  ( -0.2756373558169926130, 0.9612616959383206705, 3.682857393832930037E-14 ) ) ;
#12377=CARTESIAN_POINT ( 'NONE',  ( -40.02540636251513462, 2.839176264122873050, 37.04930799450052348 ) ) ;
#12381=CARTESIAN_POINT ( 'NONE',  ( -40.71297758125562183, 7.970149924291493271, 39.96793714460204683 ) ) ;
#12386=EDGE_CURVE ( 'NONE', #21830, #1812, #10639, .T. ) ;
#12388=( GEOMETRIC_REPRESENTATION_CONTEXT ( 3 ) GLOBAL_UNCERTAINTY_ASSIGNED_CONTEXT ( ( #21915 ) ) GLOBAL_UNIT_ASSIGNED_CONTEXT ( ( #18546, #23332, #15940 ) ) REPRESENTATION_CONTEXT ( 'NONE', 'WORKASPACE' ) );
#12389=EDGE_LOOP ( 'NONE', ( #31634, #19657, #21639, #28280 ) ) ;
#12398=EDGE_CURVE ( 'NONE', #9796, #1812, #5064, .T. ) ;
#12406=DIRECTION ( 'NONE',  ( 0.000000000000000000, 0.000000000000000000, 1.000000000000000000 ) ) ;
#12409=CARTESIAN_POINT ( 'NONE',  ( -40.02540636251513462, 2.839176264122873050, 37.04930799450052348 ) ) ;
#12412=CARTESIAN_POINT ( 'NONE',  ( -42.38687957179150345, 4.148162238788003719, 55.74930799450051211 ) ) ;
#12416=EDGE_LOOP ( 'NONE', ( #20682, #13411, #24851 ) ) ;
#12429=CARTESIAN_POINT ( 'NONE',  ( -38.37328487235789964, 6.954148266671692724, 32.09930799450052064 ) ) ;
#12430=DIRECTION ( 'NONE',  ( -0.4848096202463636484, -0.8746197071393810862, 0.000000000000000000 ) ) ;
#12438=DIRECTION ( 'NONE',  ( 0.4848096202463673121, 0.8746197071393789768, 0.000000000000000000 ) ) ;
#12439=ORIENTED_EDGE ( 'NONE', *, *, #10733, .T. ) ;
#12441=DIRECTION ( 'NONE',  ( 0.7141240004913198547, -0.3958453973320100738, -0.5773502691896283956 ) ) ;
#12447=DIRECTION ( 'NONE',  ( 1.431146867680865853E-17, 2.558717127065790464E-17, 1.000000000000000000 ) ) ;
#12449=ORIENTED_EDGE ( 'NONE', *, *, #4819, .F. ) ;
#12450=LINE ( 'NONE', #27206, #31305 ) ;
#12452=ORIENTED_EDGE ( 'NONE', *, *, #22709, .T. ) ;
#12458=LINE ( 'NONE', #27709, #4697 ) ;
#12462=ORIENTED_EDGE ( 'NONE', *, *, #18153, .F. ) ;
#12463=VECTOR ( 'NONE', #20585, 1000.000000000000000 ) ;
#12471=DIRECTION ( 'NONE',  ( -0.4848096202463430537, -0.8746197071393926326, -9.920727850371701658E-18 ) ) ;
#12475=AXIS2_PLACEMENT_3D ( 'NONE', #3759, #13944, #1450 ) ;
#12486=PRODUCT_CONTEXT ( 'NONE', #30906, 'mechanical' ) ;
#12489=DIRECTION ( 'NONE',  ( -0.3428121700606640565, -0.6184495258776567805, 0.7071067811865474617 ) ) ;
#12496=ADVANCED_FACE ( 'NONE', ( #6660 ), #27499, .T. ) ;
#12500=EDGE_CURVE ( 'NONE', #4462, #180, #7644, .T. ) ;
#12510=LINE ( 'NONE', #24808, #17534 ) ;
#12514=ORIENTED_EDGE ( 'NONE', *, *, #27507, .T. ) ;
#12520=CARTESIAN_POINT ( 'NONE',  ( -40.59307405792756640, 7.534955460439816122, 60.29072935073783412 ) ) ;
#12524=CARTESIAN_POINT ( 'NONE',  ( -40.54828680531407770, 6.846271790121643441, 39.54930799450052348 ) ) ;
#12525=EDGE_LOOP ( 'NONE', ( #32086, #6602, #23310 ) ) ;
#12537=ORIENTED_EDGE ( 'NONE', *, *, #19743, .F. ) ;
#12538=DIRECTION ( 'NONE',  ( -0.2756373558169932236, 0.9612616959383205595, -2.271050992151962865E-31 ) ) ;
#12541=CARTESIAN_POINT ( 'NONE',  ( -42.21195563036361875, 4.051200314738730768, 35.04930799450051637 ) ) ;
#12546=EDGE_CURVE ( 'NONE', #30210, #9196, #13177, .T. ) ;
#12548=AXIS2_PLACEMENT_3D ( 'NONE', #1634, #19019, #29048 ) ;
#12549=VECTOR ( 'NONE', #13068, 1000.000000000000000 ) ;
#12555=DIRECTION ( 'NONE',  ( -0.9612616959383205595, -0.2756373558169931681, 1.660411357259282445E-16 ) ) ;
#12561=DIRECTION ( 'NONE',  ( -0.2756373558169952220, 0.9612616959383201154, 0.000000000000000000 ) ) ;
#12565=DIRECTION ( 'NONE',  ( 0.000000000000000000, 0.000000000000000000, -1.000000000000000000 ) ) ;
#12566=LINE ( 'NONE', #82, #25566 ) ;
#12568=EDGE_LOOP ( 'NONE', ( #13737, #17039, #2678, #3890 ) ) ;
#12571=ORIENTED_EDGE ( 'NONE', *, *, #12235, .F. ) ;
#12582=ORIENTED_EDGE ( 'NONE', *, *, #9627, .T. ) ;
#12586=EDGE_CURVE ( 'NONE', #20229, #22591, #29799, .T. ) ;
#12592=AXIS2_PLACEMENT_3D ( 'NONE', #27815, #22548, #19926 ) ;
#12593=EDGE_LOOP ( 'NONE', ( #22840, #26688, #22243, #18693, #26364 ) ) ;
#12597=DIRECTION ( 'NONE',  ( 0.8746197071393925215, -0.4848096202463429982, -8.676864087101708112E-18 ) ) ;
#12601=EDGE_LOOP ( 'NONE', ( #22052, #17638, #30839, #4388, #754, #1653 ) ) ;
#12604=VERTEX_POINT ( 'NONE', #31092 ) ;
#12606=DIRECTION ( 'NONE',  ( 0.4848096202463645921, 0.8746197071393805311, 0.000000000000000000 ) ) ;
#12614=CARTESIAN_POINT ( 'NONE',  ( -40.11085926462317275, 6.816553873983406397, 34.73944010433842067 ) ) ;
#12619=EDGE_CURVE ( 'NONE', #13764, #2697, #6457, .T. ) ;
#12631=ORIENTED_EDGE ( 'NONE', *, *, #20084, .F. ) ;
#12635=EDGE_LOOP ( 'NONE', ( #21398, #786, #8970, #2160 ) ) ;
#12639=DIRECTION ( 'NONE',  ( 0.4848096202463783588, 0.8746197071393729816, 0.000000000000000000 ) ) ;
#12645=CIRCLE ( 'NONE', #11070, 0.1000000000000018235 ) ;
#12649=FACE_OUTER_BOUND ( 'NONE', #18586, .T. ) ;
#12652=DIRECTION ( 'NONE',  ( 0.000000000000000000, 0.000000000000000000, -1.000000000000000000 ) ) ;
#12661=DIRECTION ( 'NONE',  ( 0.4848096202463429982, 0.8746197071393925215, 9.920727850371698576E-18 ) ) ;
#12664=AXIS2_PLACEMENT_3D ( 'NONE', #15225, #2584, #12447 ) ;
#12666=CARTESIAN_POINT ( 'NONE',  ( -42.36153388572594736, 13.68895619636815475, 59.46110983642625314 ) ) ;
#12670=ADVANCED_FACE ( 'NONE', ( #18273 ), #20487, .T. ) ;
#12671=CIRCLE ( 'NONE', #15282, 0.9999999999999986677 ) ;
#12672=ORIENTED_EDGE ( 'NONE', *, *, #16517, .F. ) ;
#12683=EDGE_CURVE ( 'NONE', #12114, #27545, #23531, .T. ) ;
#12687=FACE_OUTER_BOUND ( 'NONE', #25968, .T. ) ;
#12689=FACE_OUTER_BOUND ( 'NONE', #4506, .T. ) ;
#12691=CARTESIAN_POINT ( 'NONE',  ( -40.90015969217747482, 8.955334253785164123, 57.04930799450051637 ) ) ;
#12692=DIRECTION ( 'NONE',  ( 0.8746197071393926326, -0.4848096202463430537, -8.676864087101709653E-18 ) ) ;
#12693=CARTESIAN_POINT ( 'NONE',  ( -42.38687957179149635, 4.148162238787999279, 35.14930799450051779 ) ) ;
#12704=EDGE_LOOP ( 'NONE', ( #10011, #9567 ) ) ;
#12708=ORIENTED_EDGE ( 'NONE', *, *, #6183, .T. ) ;
#12715=CARTESIAN_POINT ( 'NONE',  ( -40.64500813507293486, 6.819128862114091305, 34.57932936825760351 ) ) ;
#12717=EDGE_LOOP ( 'NONE', ( #7558, #9329, #22593, #17548 ) ) ;
#12719=AXIS2_PLACEMENT_3D ( 'NONE', #3541, #13732, #23566 ) ;
#12722=LINE ( 'NONE', #17619, #26534 ) ;
#12723=CARTESIAN_POINT ( 'NONE',  ( -40.38516919650994197, 8.640923867788874446, 39.44930799450052206 ) ) ;
#12730=DIRECTION ( 'NONE',  ( 0.4848096202463430537, 0.8746197071393926326, -1.125439520643636483E-16 ) ) ;
#12732=ORIENTED_EDGE ( 'NONE', *, *, #9375, .F. ) ;
#12734=LINE ( 'NONE', #240, #9525 ) ;
#12737=DIRECTION ( 'NONE',  ( -0.4848096202463424431, -0.8746197071393927436, 2.220446049250312588E-16 ) ) ;
#12746=FACE_OUTER_BOUND ( 'NONE', #16742, .T. ) ;
#12747=CYLINDRICAL_SURFACE ( 'NONE', #11168, 1.500000000000001332 ) ;
#12748=VECTOR ( 'NONE', #317, 1000.000000000000000 ) ;
#12752=ORIENTED_EDGE ( 'NONE', *, *, #2663, .T. ) ;
#12754=ORIENTED_EDGE ( 'NONE', *, *, #26689, .F. ) ;
#12764=AXIS2_PLACEMENT_3D ( 'NONE', #5405, #15409, #25420 ) ;
#12765=DIRECTION ( 'NONE',  ( 0.9612616959383207815, 0.2756373558169927240, 8.795445018804291370E-19 ) ) ;
#12768=ORIENTED_EDGE ( 'NONE', *, *, #8407, .T. ) ;
#12780=AXIS2_PLACEMENT_3D ( 'NONE', #18191, #3910, #11151 ) ;
#12781=DIRECTION ( 'NONE',  ( 0.8746197071393858602, -0.4848096202463547666, 0.000000000000000000 ) ) ;
#12782=FACE_OUTER_BOUND ( 'NONE', #19945, .T. ) ;
#12786=CARTESIAN_POINT ( 'NONE',  ( -40.44437521412186243, 7.396217677353668307, 34.54930799450052348 ) ) ;
#12788=CARTESIAN_POINT ( 'NONE',  ( -41.34584395867850048, 11.59800658573647425, 57.95249952744806166 ) ) ;
#12789=EDGE_LOOP ( 'NONE', ( #4324, #7991, #1736, #15236, #1558, #9131 ) ) ;
#12791=DIRECTION ( 'NONE',  ( -0.2756373558169638582, 0.9612616959383291082, -1.479773560108318178E-16 ) ) ;
#12799=VERTEX_POINT ( 'NONE', #1688 ) ;
#12810=AXIS2_PLACEMENT_3D ( 'NONE', #20176, #29711, #24615 ) ;
#12814=EDGE_CURVE ( 'NONE', #24996, #18438, #19969, .T. ) ;
#12817=ORIENTED_EDGE ( 'NONE', *, *, #5970, .F. ) ;
#12824=DIRECTION ( 'NONE',  ( -0.2756373558169973870, 0.9612616959383193382, -9.615507602343155278E-33 ) ) ;
#12827=ORIENTED_EDGE ( 'NONE', *, *, #482, .F. ) ;
#12829=( BOUNDED_SURFACE ( )  B_SPLINE_SURFACE ( 3, 2, ( 
 ( #13342, #10720, #23499 ),
 ( #10387, #30416, #2983 ),
 ( #30741, #5619, #27948 ),
 ( #10877, #5950, #23011 ),
 ( #527, #5468, #1012 ),
 ( #15468, #3141, #8248 ),
 ( #18235, #13185, #28268 ),
 ( #5787, #15794, #8881 ) ),
 .UNSPECIFIED., .F., .F., .F. ) 
 B_SPLINE_SURFACE_WITH_KNOTS ( ( 4, 2, 2, 4 ),
 ( 3, 3 ),
 ( -3.388131789017201356E-18, 0.0005623261017282641955, 0.0008434891525923980280, 0.001124652203456531861 ),
 ( 0.000000000000000000, 1.000000000000000000 ),
 .UNSPECIFIED. ) 
 GEOMETRIC_REPRESENTATION_ITEM ( )  RATIONAL_B_SPLINE_SURFACE ( (
 ( 1.000000000000000000, 0.7071067811865558994, 1.000000000000000000),
 ( 1.000000000000000000, 0.6846567335763826812, 1.000000000000000000),
 ( 1.000000000000000000, 0.6190846722315239692, 1.000000000000000000),
 ( 1.000000000000000000, 0.5161161862684999768, 1.000000000000000000),
 ( 1.000000000000000000, 0.4814351115863779174, 1.000000000000000000),
 ( 1.000000000000000000, 0.4264341115146433325, 1.000000000000000000),
 ( 1.000000000000000000, 0.4080770041854601127, 1.000000000000000000),
 ( 1.000000000000000000, 0.4082482904638556342, 1.000000000000000000) ) ) 
 REPRESENTATION_ITEM ( '' )  SURFACE ( )  );
#12831=CARTESIAN_POINT ( 'NONE',  ( -39.67555847965937943, 2.645252416024337361, 47.04930799450051637 ) ) ;
#12832=ADVANCED_FACE ( 'NONE', ( #14336 ), #24328, .F. ) ;
#12834=AXIS2_PLACEMENT_3D ( 'NONE', #12925, #2417, #25383 ) ;
#12837=AXIS2_PLACEMENT_3D ( 'NONE', #3538, #433, #31128 ) ;
#12839=ORIENTED_EDGE ( 'NONE', *, *, #7258, .T. ) ;
#12840=FACE_OUTER_BOUND ( 'NONE', #26647, .T. ) ;
#12842=DIRECTION ( 'NONE',  ( -1.188208965918165239E-16, -1.880121038077813132E-16, -1.000000000000000000 ) ) ;
#12844=DIRECTION ( 'NONE',  ( 0.9612616959383221138, 0.2756373558169876170, 0.000000000000000000 ) ) ;
#12847=FACE_OUTER_BOUND ( 'NONE', #19476, .T. ) ;
#12863=CARTESIAN_POINT ( 'NONE',  ( -41.75126335834794133, 15.45321085637654690, 38.54111136810265492 ) ) ;
#12869=AXIS2_PLACEMENT_3D ( 'NONE', #31031, #666, #10699 ) ;
#12872=ADVANCED_FACE ( 'NONE', ( #24995 ), #31902, .T. ) ;
#12873=EDGE_LOOP ( 'NONE', ( #22423, #19115, #9772, #23565, #24895 ) ) ;
#12874=B_SPLINE_CURVE_WITH_KNOTS ( 'NONE', 3,
 ( #14213, #16497, #19271, #21577 ),
 .UNSPECIFIED., .F., .F.,
 ( 4, 4 ),
 ( 0.000000000000000000, 0.0001555497290426954599 ),
 .UNSPECIFIED. ) ;
#12876=CARTESIAN_POINT ( 'NONE',  ( -39.58809650894544774, 2.596771453999702661, 45.04930799450051637 ) ) ;
#12878=ORIENTED_EDGE ( 'NONE', *, *, #19208, .F. ) ;
#12886=ORIENTED_EDGE ( 'NONE', *, *, #6933, .F. ) ;
#12890=FACE_OUTER_BOUND ( 'NONE', #17714, .T. ) ;
#12894=VERTEX_POINT ( 'NONE', #10068 ) ;
#12899=AXIS2_PLACEMENT_3D ( 'NONE', #22298, #6887, #30473 ) ;
#12900=CARTESIAN_POINT ( 'NONE',  ( -43.29662792673756400, 1.063067023446606196, 60.54930799450051637 ) ) ;
#12903=DIRECTION ( 'NONE',  ( 0.9612616959383205595, 0.2756373558169932236, -1.660411357259282445E-16 ) ) ;
#12907=DIRECTION ( 'NONE',  ( 0.000000000000000000, 0.000000000000000000, -1.000000000000000000 ) ) ;
#12909=ORIENTED_EDGE ( 'NONE', *, *, #15164, .F. ) ;
#12919=ORIENTED_EDGE ( 'NONE', *, *, #27914, .F. ) ;
#12925=CARTESIAN_POINT ( 'NONE',  ( -40.23967075304302909, 7.740322171013526820, 60.29072935073781991 ) ) ;
#12928=VECTOR ( 'NONE', #13492, 1000.000000000000227 ) ;
#12929=CARTESIAN_POINT ( 'NONE',  ( -40.98031486389898248, 9.265261353013489298, 39.44930799450052206 ) ) ;
#12934=DIRECTION ( 'NONE',  ( -0.4848096202463421656, -0.8746197071393929656, -9.920727850371707821E-18 ) ) ;
#12937=DIRECTION ( 'NONE',  ( -0.2756373558169974980, 0.9612616959383193382, 1.315048337272770589E-17 ) ) ;
#12940=LINE ( 'NONE', #12786, #21919 ) ;
#12947=ORIENTED_EDGE ( 'NONE', *, *, #10772, .F. ) ;
#12954=ADVANCED_FACE ( 'NONE', ( #23175, #20547 ), #5303, .T. ) ;
#12958=CARTESIAN_POINT ( 'NONE',  ( -41.24971778908466291, 11.62557032131817358, 58.05249952744806308 ) ) ;
#12974=CIRCLE ( 'NONE', #23431, 1.042135311067126979 ) ;
#12975=DIRECTION ( 'NONE',  ( 0.7141240004913198547, -0.3958453973320100738, -0.5773502691896283956 ) ) ;
#12984=ORIENTED_EDGE ( 'NONE', *, *, #4758, .F. ) ;
#12988=EDGE_CURVE ( 'NONE', #16322, #32074, #361, .T. ) ;
#12991=CARTESIAN_POINT ( 'NONE',  ( -40.02540636251514172, 2.839176264122877047, 58.34930799450052064 ) ) ;
#12995=CARTESIAN_POINT ( 'NONE',  ( -40.02540636251513462, 2.839176264122874382, 35.74930799450051921 ) ) ;
#12998=CARTESIAN_POINT ( 'NONE',  ( -40.28779227465695811, 2.984619150196779369, 55.54930799450051637 ) ) ;
#13000=DIRECTION ( 'NONE',  ( 0.9612616959383193382, 0.2756373558169973870, 8.795445018804928853E-19 ) ) ;
#13021=AXIS2_PLACEMENT_3D ( 'NONE', #18360, #18524, #5743 ) ;
#13024=VECTOR ( 'NONE', #10778, 1000.000000000000114 ) ;
#13029=AXIS2_PLACEMENT_3D ( 'NONE', #19218, #31874, #19388 ) ;
#13030=ORIENTED_EDGE ( 'NONE', *, *, #5201, .F. ) ;
#13035=DIRECTION ( 'NONE',  ( -0.9612616959383204485, -0.2756373558169933347, 1.660411357259282692E-16 ) ) ;
#13040=ORIENTED_EDGE ( 'NONE', *, *, #13362, .T. ) ;
#13041=DIRECTION ( 'NONE',  ( 0.000000000000000000, 0.000000000000000000, 1.000000000000000000 ) ) ;
#13050=DIRECTION ( 'NONE',  ( 0.1949050434465250392, -0.6797146636928682595, -0.7071067811865470176 ) ) ;
#13052=EDGE_CURVE ( 'NONE', #11721, #6336, #16735, .T. ) ;
#13054=AXIS2_PLACEMENT_3D ( 'NONE', #11674, #31695, #9206 ) ;
#13059=VERTEX_POINT ( 'NONE', #8720 ) ;
#13068=DIRECTION ( 'NONE',  ( 2.779292025043186357E-18, -1.288349127009862211E-17, 1.000000000000000000 ) ) ;
#13069=ORIENTED_EDGE ( 'NONE', *, *, #8134, .T. ) ;
#13076=CARTESIAN_POINT ( 'NONE',  ( -41.77464577679392477, 3.808795504615560379, 45.04930799450051637 ) ) ;
#13091=ORIENTED_EDGE ( 'NONE', *, *, #17568, .T. ) ;
#13092=CARTESIAN_POINT ( 'NONE',  ( -40.02540636251514172, 2.839176264122877047, 59.04930799450051637 ) ) ;
#13093=CIRCLE ( 'NONE', #21956, 1.524998423334080533 ) ;
#13097=LINE ( 'NONE', #13569, #27438 ) ;
#13101=ORIENTED_EDGE ( 'NONE', *, *, #15890, .F. ) ;
#13102=FACE_OUTER_BOUND ( 'NONE', #6201, .T. ) ;
#13106=CARTESIAN_POINT ( 'NONE',  ( -42.38687957179149635, 4.148162238787999279, 37.04930799450052348 ) ) ;
#13107=EDGE_CURVE ( 'NONE', #1328, #31727, #22985, .T. ) ;
#13109=AXIS2_PLACEMENT_3D ( 'NONE', #7694, #2597, #30182 ) ;
#13112=ORIENTED_EDGE ( 'NONE', *, *, #29432, .F. ) ;
#13115=AXIS2_PLACEMENT_3D ( 'NONE', #3422, #15737, #20659 ) ;
#13117=EDGE_LOOP ( 'NONE', ( #20273, #28247, #27892, #14080, #15517 ) ) ;
#13120=LINE ( 'NONE', #30834, #4995 ) ;
#13125=ORIENTED_EDGE ( 'NONE', *, *, #16222, .F. ) ;
#13128=ORIENTED_EDGE ( 'NONE', *, *, #24154, .F. ) ;
#13132=DIRECTION ( 'NONE',  ( 0.9612616959383205595, 0.2756373558169932236, -1.660411357259282445E-16 ) ) ;
#13135=CARTESIAN_POINT ( 'NONE',  ( -43.73393778030726509, 1.305471833569777695, 60.44930799450051495 ) ) ;
#13137=DIRECTION ( 'NONE',  ( -0.2756373558169954441, 0.9612616959383198934, -1.479773560108263451E-16 ) ) ;
#13140=DIRECTION ( 'NONE',  ( -0.9612616959383207815, -0.2756373558169926685, -8.795445018804289444E-19 ) ) ;
#13145=CARTESIAN_POINT ( 'NONE',  ( -43.43257085947613660, 1.024086014757300989, 53.64930799450051779 ) ) ;
#13146=ORIENTED_EDGE ( 'NONE', *, *, #11166, .T. ) ;
#13147=CIRCLE ( 'NONE', #28850, 0.9031915329475519449 ) ;
#13148=AXIS2_PLACEMENT_3D ( 'NONE', #29082, #4128, #11691 ) ;
#13152=ORIENTED_EDGE ( 'NONE', *, *, #9865, .F. ) ;
#13162=VECTOR ( 'NONE', #30284, 999.9999999999998863 ) ;
#13169=AXIS2_PLACEMENT_3D ( 'NONE', #19389, #16763, #17252 ) ;
#13170=CARTESIAN_POINT ( 'NONE',  ( -42.38687957179150345, 4.148162238788004608, 59.04930799450051637 ) ) ;
#13174=ORIENTED_EDGE ( 'NONE', *, *, #28797, .F. ) ;
#13176=LINE ( 'NONE', #8242, #13953 ) ;
#13177=CIRCLE ( 'NONE', #7926, 0.1000000000000006301 ) ;
#13181=EDGE_CURVE ( 'NONE', #3549, #4111, #3071, .T. ) ;
#13183=ORIENTED_EDGE ( 'NONE', *, *, #7759, .F. ) ;
#13184=LINE ( 'NONE', #21175, #7213 ) ;
#13185=CARTESIAN_POINT ( 'NONE',  ( -40.02353495282824980, 6.996741953892005483, 39.48683338133720611 ) ) ;
#13187=ORIENTED_EDGE ( 'NONE', *, *, #6836, .F. ) ;
#13197=CIRCLE ( 'NONE', #27337, 1.624998423334082620 ) ;
#13200=CIRCLE ( 'NONE', #30490, 0.1000000000000037248 ) ;
#13205=EDGE_CURVE ( 'NONE', #32001, #1884, #5710, .T. ) ;
#13207=CARTESIAN_POINT ( 'NONE',  ( -40.44300931641782171, 7.361061430353638357, 60.31640775708849844 ) ) ;
#13209=VERTEX_POINT ( 'NONE', #22477 ) ;
#13210=CARTESIAN_POINT ( 'NONE',  ( -41.01929587258828036, 9.401204285752060130, 38.64930799450052490 ) ) ;
#13211=LINE ( 'NONE', #28138, #10493 ) ;
#13212=CARTESIAN_POINT ( 'NONE',  ( -40.28779227465695101, 2.984619150196775816, 37.04930799450052348 ) ) ;
#13213=FACE_OUTER_BOUND ( 'NONE', #19322, .T. ) ;
#13214=CARTESIAN_POINT ( 'NONE',  ( -40.69571722278731585, 6.786566810383049209, 39.44930799450052206 ) ) ;
#13215=VERTEX_POINT ( 'NONE', #2471 ) ;
#13218=CARTESIAN_POINT ( 'NONE',  ( -40.46271621608484281, 3.081581074246049212, 55.54930799450051637 ) ) ;
#13226=PLANE ( 'NONE',  #1239 ) ;
#13228=CARTESIAN_POINT ( 'NONE',  ( -42.47434154250543514, 4.196643200812633978, 35.74930799450051921 ) ) ;
#13229=EDGE_CURVE ( 'NONE', #11324, #7112, #1974, .T. ) ;
#13230=CARTESIAN_POINT ( 'NONE',  ( -41.02113223168485234, 7.230835263863471418, 34.54930799450052348 ) ) ;
#13243=FACE_OUTER_BOUND ( 'NONE', #5897, .T. ) ;
#13244=CARTESIAN_POINT ( 'NONE',  ( -40.18454328187963398, 7.548069831825862330, 60.54930799450051637 ) ) ;
#13246=EDGE_CURVE ( 'NONE', #23906, #10175, #14621, .T. ) ;
#13248=ORIENTED_EDGE ( 'NONE', *, *, #6557, .T. ) ;
#13250=EDGE_LOOP ( 'NONE', ( #12571, #19731, #13379, #7417 ) ) ;
#13253=DIRECTION ( 'NONE',  ( -0.8746197071393790878, 0.4848096202463673676, 1.277302113040196197E-17 ) ) ;
#13254=VERTEX_POINT ( 'NONE', #12327 ) ;
#13255=CARTESIAN_POINT ( 'NONE',  ( -40.49096175631598271, 7.521145078229855230, 60.14930799450051779 ) ) ;
#13256=ORIENTED_EDGE ( 'NONE', *, *, #31584, .F. ) ;
#13259=ORIENTED_EDGE ( 'NONE', *, *, #30953, .F. ) ;
#13262=FACE_OUTER_BOUND ( 'NONE', #3462, .T. ) ;
#13278=EDGE_CURVE ( 'NONE', #1764, #5962, #12162, .T. ) ;
#13282=EDGE_LOOP ( 'NONE', ( #8188, #31002, #31817, #16248 ) ) ;
#13293=ORIENTED_EDGE ( 'NONE', *, *, #16110, .F. ) ;
#13294=EDGE_LOOP ( 'NONE', ( #28424, #18880, #31670, #15195 ) ) ;
#13299=CARTESIAN_POINT ( 'NONE',  ( -41.88090303775678080, 13.82677487427665675, 59.54930799450050927 ) ) ;
#13300=CARTESIAN_POINT ( 'NONE',  ( -40.48129536610376533, 8.613360132207176889, 39.44930799450052206 ) ) ;
#13307=FACE_OUTER_BOUND ( 'NONE', #20543, .T. ) ;
#13308=AXIS2_PLACEMENT_3D ( 'NONE', #5450, #2335, #7589 ) ;
#13318=CARTESIAN_POINT ( 'NONE',  ( -40.65487266620045403, 9.475231293617264683, 38.63717596014456035 ) ) ;
#13325=DIRECTION ( 'NONE',  ( 0.2756373558169954441, -0.9612616959383198934, 5.348665517716782531E-31 ) ) ;
#13331=CARTESIAN_POINT ( 'NONE',  ( -40.80097511801616150, 8.246641009394465982, 54.44930799450051495 ) ) ;
#13332=AXIS2_PLACEMENT_3D ( 'NONE', #10800, #13573, #28354 ) ;
#13334=CYLINDRICAL_SURFACE ( 'NONE', #2661, 2.000000000000001776 ) ;
#13335=DIRECTION ( 'NONE',  ( -0.8746197071393858602, 0.4848096202463547666, 0.000000000000000000 ) ) ;
#13342=CARTESIAN_POINT ( 'NONE',  ( -40.16503835899720087, 7.510440877657823755, 38.80028690913361800 ) ) ;
#13344=CARTESIAN_POINT ( 'NONE',  ( -40.02540636251513462, 2.839176264122873050, 35.04930799450051637 ) ) ;
#13348=AXIS2_PLACEMENT_3D ( 'NONE', #6276, #16597, #3975 ) ;
#13352=DIRECTION ( 'NONE',  ( 0.2756373558170140403, -0.9612616959383146753, -1.315048337272768740E-17 ) ) ;
#13354=EDGE_CURVE ( 'NONE', #23633, #23532, #20340, .T. ) ;
#13360=FACE_OUTER_BOUND ( 'NONE', #15184, .T. ) ;
#13362=EDGE_CURVE ( 'NONE', #21602, #90, #10444, .T. ) ;
#13365=DIRECTION ( 'NONE',  ( -0.9612616959383207815, -0.2756373558169926685, -8.795445018804291370E-19 ) ) ;
#13369=AXIS2_PLACEMENT_3D ( 'NONE', #28099, #507, #2968 ) ;
#13377=CIRCLE ( 'NONE', #20688, 1.042135311067126979 ) ;
#13379=ORIENTED_EDGE ( 'NONE', *, *, #25567, .T. ) ;
#13382=DIRECTION ( 'NONE',  ( 0.9612616959383250004, 0.2756373558169784577, -1.660411357259259765E-16 ) ) ;
#13384=CARTESIAN_POINT ( 'NONE',  ( -41.02687597405218156, 7.220473278338834788, 60.54930799450051637 ) ) ;
#13389=LINE ( 'NONE', #413, #12549 ) ;
#13390=ORIENTED_EDGE ( 'NONE', *, *, #15164, .T. ) ;
#13391=EDGE_CURVE ( 'NONE', #32074, #5664, #8352, .T. ) ;
#13393=CIRCLE ( 'NONE', #6047, 0.09999999999999795164 ) ;
#13397=AXIS2_PLACEMENT_3D ( 'NONE', #17128, #9270, #1879 ) ;
#13400=CARTESIAN_POINT ( 'NONE',  ( -40.64704422177600662, 9.403915785377417791, 34.54930799450051637 ) ) ;
#13409=ORIENTED_EDGE ( 'NONE', *, *, #30737, .F. ) ;
#13410=CYLINDRICAL_SURFACE ( 'NONE', #17026, 0.1000000000000018235 ) ;
#13411=ORIENTED_EDGE ( 'NONE', *, *, #29160, .T. ) ;
#13414=VERTEX_POINT ( 'NONE', #31335 ) ;
#13415=CARTESIAN_POINT ( 'NONE',  ( -40.47970302497625994, 7.463434137431150361, 60.44930799450051495 ) ) ;
#13417=CARTESIAN_POINT ( 'NONE',  ( -40.52064562223811350, 7.631811404637807605, 53.92244792118258090 ) ) ;
#13423=ORIENTED_EDGE ( 'NONE', *, *, #26387, .F. ) ;
#13429=ORIENTED_EDGE ( 'NONE', *, *, #19622, .T. ) ;
#13430=ORIENTED_EDGE ( 'NONE', *, *, #8532, .F. ) ;
#13434=EDGE_CURVE ( 'NONE', #3392, #21636, #21633, .T. ) ;
#13437=ORIENTED_EDGE ( 'NONE', *, *, #19817, .T. ) ;
#13455=DIRECTION ( 'NONE',  ( -0.4848096202463430537, -0.8746197071393926326, -9.920727850371701658E-18 ) ) ;
#13461=EDGE_CURVE ( 'NONE', #28053, #16797, #25647, .T. ) ;
#13465=CARTESIAN_POINT ( 'NONE',  ( -42.22138300640814634, 14.68176690255379491, 35.90717268343339441 ) ) ;
#13466=CARTESIAN_POINT ( 'NONE',  ( -40.57832940339287831, 7.446916344587784842, 53.80788663826320573 ) ) ;
#13478=CARTESIAN_POINT ( 'NONE',  ( -40.23672901771082877, 7.760455916344220384, 34.54930799450052348 ) ) ;
#13480=CARTESIAN_POINT ( 'NONE',  ( -40.09211399732166115, 9.667069410243959382, 39.44930799450052206 ) ) ;
#13482=CYLINDRICAL_SURFACE ( 'NONE', #24493, 0.09999999999999945044 ) ;
#13484=DIRECTION ( 'NONE',  ( 0.4848096202463424431, 0.8746197071393927436, -2.220446049250312588E-16 ) ) ;
#13485=LINE ( 'NONE', #23486, #11792 ) ;
#13492=DIRECTION ( 'NONE',  ( 0.2756373558169954441, -0.9612616959383198934, 1.479773560108263204E-16 ) ) ;
#13496=VERTEX_POINT ( 'NONE', #26074 ) ;
#13497=( BOUNDED_CURVE ( )  B_SPLINE_CURVE ( 3, ( #6533, #11942, #21936, #29673 ),
 .UNSPECIFIED., .F., .F. ) 
 B_SPLINE_CURVE_WITH_KNOTS ( ( 4, 4 ),
 ( 1.558993681807626333E-14, 1.570796326794877240 ),
 .UNSPECIFIED. ) 
 CURVE ( )  GEOMETRIC_REPRESENTATION_ITEM ( )  RATIONAL_B_SPLINE_CURVE ( ( 1.000000000000000000, 0.8047378541243732641, 0.8047378541243732641, 1.000000000000000000 ) ) 
 REPRESENTATION_ITEM ( '' )  );
#13501=FACE_OUTER_BOUND ( 'NONE', #9494, .T. ) ;
#13508=ORIENTED_EDGE ( 'NONE', *, *, #1216, .T. ) ;
#13509=VECTOR ( 'NONE', #24327, 1000.000000000000000 ) ;
#13513=ORIENTED_EDGE ( 'NONE', *, *, #21783, .F. ) ;
#13515=CARTESIAN_POINT ( 'NONE',  ( -40.18454328187963398, 7.548069831825863218, 53.64930799450051779 ) ) ;
#13517=VERTEX_POINT ( 'NONE', #1614 ) ;
#13519=CARTESIAN_POINT ( 'NONE',  ( -42.73182147790732444, -0.8057266458565844891, 32.14930799450051779 ) ) ;
#13528=DIRECTION ( 'NONE',  ( -2.779292025043186357E-18, 1.288349127009862211E-17, -1.000000000000000000 ) ) ;
#13529=VERTEX_POINT ( 'NONE', #11637 ) ;
#13535=CARTESIAN_POINT ( 'NONE',  ( -40.44437521412185532, 7.396217677353669195, 39.44930799450052206 ) ) ;
#13537=EDGE_CURVE ( 'NONE', #14722, #6401, #8527, .T. ) ;
#13545=TOROIDAL_SURFACE ( 'NONE', #15115, 0.8928932188134564019, 0.1000000000000000056 ) ;
#13549=FACE_OUTER_BOUND ( 'NONE', #6575, .T. ) ;
#13550=CARTESIAN_POINT ( 'NONE',  ( -40.60249826926477823, 9.398840415180675478, 34.59072935073783128 ) ) ;
#13556=LINE ( 'NONE', #22013, #9135 ) ;
#13567=DIRECTION ( 'NONE',  ( 0.2756373558170082672, -0.9612616959383162296, 0.000000000000000000 ) ) ;
#13569=CARTESIAN_POINT ( 'NONE',  ( -41.04685960816998147, 9.497330455345890599, 35.54930799450052348 ) ) ;
#13573=DIRECTION ( 'NONE',  ( 0.2756373558169932236, -0.9612616959383205595, 1.479773560108267395E-16 ) ) ;
#13575=CARTESIAN_POINT ( 'NONE',  ( -41.24971778908466291, 11.62557032131817181, 56.04611646155296256 ) ) ;
#13576=CIRCLE ( 'NONE', #30346, 0.1000000000000007272 ) ;
#13581=EDGE_CURVE ( 'NONE', #28526, #30980, #21950, .T. ) ;
#13582=VERTEX_POINT ( 'NONE', #29354 ) ;
#13583=EDGE_CURVE ( 'NONE', #31727, #1328, #21948, .T. ) ;
#13584=VERTEX_POINT ( 'NONE', #32313 ) ;
#13600=CARTESIAN_POINT ( 'NONE',  ( -43.64647580959332629, 1.256990871545142774, 60.54930799450051637 ) ) ;
#13601=EDGE_CURVE ( 'NONE', #1187, #18622, #7030, .T. ) ;
#13606=DIRECTION ( 'NONE',  ( 0.1949050434465282866, -0.6797146636928672603, 0.7071067811865469066 ) ) ;
#13609=DIRECTION ( 'NONE',  ( -0.8746197071393823075, 0.4848096202463614279, 0.000000000000000000 ) ) ;
#13621=EDGE_CURVE ( 'NONE', #3661, #13254, #14634, .T. ) ;
#13622=AXIS2_PLACEMENT_3D ( 'NONE', #8113, #20895, #20737 ) ;
#13627=ORIENTED_EDGE ( 'NONE', *, *, #1926, .F. ) ;
#13629=DIRECTION ( 'NONE',  ( 0.1949050434465268156, -0.6797146636928667052, 0.7071067811865480168 ) ) ;
#13638=EDGE_CURVE ( 'NONE', #2431, #13895, #3676, .T. ) ;
#13640=DIRECTION ( 'NONE',  ( 0.4848096202463489934, 0.8746197071393893019, 9.920727850371641569E-18 ) ) ;
#13645=EDGE_CURVE ( 'NONE', #9452, #12114, #3509, .T. ) ;
#13646=CARTESIAN_POINT ( 'NONE',  ( -42.03703168893574116, 3.954238390689462257, 45.14930799450051779 ) ) ;
#13648=DIRECTION ( 'NONE',  ( 0.2756373558169954441, -0.9612616959383198934, -1.163221239882716147E-31 ) ) ;
#13664=ADVANCED_FACE ( 'NONE', ( #27989 ), #20428, .T. ) ;
#13667=CIRCLE ( 'NONE', #16790, 0.9031915329475502796 ) ;
#13671=CARTESIAN_POINT ( 'NONE',  ( -40.21210701746133509, 7.644196001419694575, 53.80788663826320573 ) ) ;
#13675=VERTEX_POINT ( 'NONE', #8286 ) ;
#13677=DIRECTION ( 'NONE',  ( -0.4848096202463636484, -0.8746197071393810862, 0.000000000000000000 ) ) ;
#13691=AXIS2_PLACEMENT_3D ( 'NONE', #32136, #29177, #4719 ) ;
#13695=ORIENTED_EDGE ( 'NONE', *, *, #21668, .F. ) ;
#13717=EDGE_LOOP ( 'NONE', ( #2056, #22609, #7930, #20815 ) ) ;
#13718=CARTESIAN_POINT ( 'NONE',  ( -40.11286833322908052, 2.887657226147511302, 57.04930799450051637 ) ) ;
#13723=DIRECTION ( 'NONE',  ( 0.4848096202463636484, 0.8746197071393810862, 0.000000000000000000 ) ) ;
#13725=VECTOR ( 'NONE', #7265, 1000.000000000000000 ) ;
#13728=CARTESIAN_POINT ( 'NONE',  ( -40.11286833322907341, 2.887657226147505973, 35.04930799450051637 ) ) ;
#13732=DIRECTION ( 'NONE',  ( -0.4848096202463430537, -0.8746197071393926326, -9.920727850371701658E-18 ) ) ;
#13733=CYLINDRICAL_SURFACE ( 'NONE', #7913, 0.1000000000000004774 ) ;
#13737=ORIENTED_EDGE ( 'NONE', *, *, #12546, .T. ) ;
#13739=CARTESIAN_POINT ( 'NONE',  ( -40.56960242289638074, 7.470141326141484406, 35.42729059962400839 ) ) ;
#13740=ORIENTED_EDGE ( 'NONE', *, *, #29020, .T. ) ;
#13743=CARTESIAN_POINT ( 'NONE',  ( -44.16550389150962985, 1.558238629217585380, 39.44930799450052916 ) ) ;
#13752=ORIENTED_EDGE ( 'NONE', *, *, #10572, .T. ) ;
#13758=DIRECTION ( 'NONE',  ( 0.8746197071393926326, -0.4848096202463430537, -8.676864087101709653E-18 ) ) ;
#13763=ORIENTED_EDGE ( 'NONE', *, *, #19817, .F. ) ;
#13764=VERTEX_POINT ( 'NONE', #6303 ) ;
#13775=VERTEX_POINT ( 'NONE', #6953 ) ;
#13776=LINE ( 'NONE', #21298, #2965 ) ;
#13784=CARTESIAN_POINT ( 'NONE',  ( -40.37748943095153464, 8.220953018982690708, 59.50788663826320146 ) ) ;
#13785=VERTEX_POINT ( 'NONE', #21715 ) ;
#13791=CYLINDRICAL_SURFACE ( 'NONE', #3401, 0.1000000000000008243 ) ;
#13793=CARTESIAN_POINT ( 'NONE',  ( -40.60722745863126448, 9.415333058485025219, 39.54930799450052348 ) ) ;
#13798=EDGE_CURVE ( 'NONE', #17347, #18870, #1698, .T. ) ;
#13800=DIRECTION ( 'NONE',  ( -2.779292025043186357E-18, 1.288349127009862211E-17, -1.000000000000000000 ) ) ;
#13801=ORIENTED_EDGE ( 'NONE', *, *, #20650, .F. ) ;
#13802=CARTESIAN_POINT ( 'NONE',  ( -40.68997348041997952, 6.796928795907699161, 53.64930799450051779 ) ) ;
#13807=( NAMED_UNIT ( * ) SI_UNIT ( $, .STERADIAN. ) SOLID_ANGLE_UNIT ( ) );
#13814=ORIENTED_EDGE ( 'NONE', *, *, #10351, .F. ) ;
#13818=CIRCLE ( 'NONE', #20085, 0.09999999999999795164 ) ;
#13819=ADVANCED_FACE ( 'NONE', ( #11388 ), #14345, .T. ) ;
#13823=ADVANCED_FACE ( 'NONE', ( #31583 ), #11878, .F. ) ;
#13836=CARTESIAN_POINT ( 'NONE',  ( -41.08312911723392347, 9.261021737272178811, 34.59072935073783128 ) ) ;
#13841=FACE_OUTER_BOUND ( 'NONE', #12789, .T. ) ;
#13849=CIRCLE ( 'NONE', #32196, 0.1000000000000006301 ) ;
#13853=DIRECTION ( 'NONE',  ( 0.1949050434465282033, -0.6797146636928673713, -0.7071067811865469066 ) ) ;
#13856=CYLINDRICAL_SURFACE ( 'NONE', #24093, 0.1000000000000018235 ) ;
#13857=DIRECTION ( 'NONE',  ( -0.2756373558169959437, 0.9612616959383197823, 0.000000000000000000 ) ) ;
#13860=EDGE_CURVE ( 'NONE', #14722, #5569, #20951, .T. ) ;
#13862=AXIS2_PLACEMENT_3D ( 'NONE', #22171, #17084, #21842 ) ;
#13863=ORIENTED_EDGE ( 'NONE', *, *, #2310, .T. ) ;
#13867=EDGE_CURVE ( 'NONE', #20511, #17141, #29115, .T. ) ;
#13868=AXIS2_PLACEMENT_3D ( 'NONE', #20691, #5926, #28413 ) ;
#13870=AXIS2_PLACEMENT_3D ( 'NONE', #20852, #29708, #24122 ) ;
#13873=AXIS2_PLACEMENT_3D ( 'NONE', #25540, #18467, #32045 ) ;
#13882=DIRECTION ( 'NONE',  ( 0.8746197071393926326, -0.4848096202463430537, -8.676864087101709653E-18 ) ) ;
#13893=PLANE ( 'NONE',  #14882 ) ;
#13895=VERTEX_POINT ( 'NONE', #18921 ) ;
#13897=CARTESIAN_POINT ( 'NONE',  ( -40.23971823762673239, 6.784144620117123381, 60.44930799450051495 ) ) ;
#13914=DIRECTION ( 'NONE',  ( 0.9612616959383205595, 0.2756373558169930571, -1.660411357259282199E-16 ) ) ;
#13923=ORIENTED_EDGE ( 'NONE', *, *, #2442, .T. ) ;
#13927=ORIENTED_EDGE ( 'NONE', *, *, #11827, .T. ) ;
#13929=CARTESIAN_POINT ( 'NONE',  ( -40.60023598829667435, 7.576973264584798251, 38.76008276981544753 ) ) ;
#13931=CARTESIAN_POINT ( 'NONE',  ( -42.38263560350583248, 14.61917486843862868, 60.54930799450051637 ) ) ;
#13934=CYLINDRICAL_SURFACE ( 'NONE', #22046, 1.199999999999999734 ) ;
#13936=ORIENTED_EDGE ( 'NONE', *, *, #31395, .F. ) ;
#13942=CARTESIAN_POINT ( 'NONE',  ( -41.08785830660041682, 9.277514380576530328, 39.54930799450052348 ) ) ;
#13944=DIRECTION ( 'NONE',  ( 0.8746197071393926326, -0.4848096202463430537, -8.676864087101709653E-18 ) ) ;
#13952=EDGE_CURVE ( 'NONE', #18438, #24996, #6266, .T. ) ;
#13953=VECTOR ( 'NONE', #10715, 1000.000000000000000 ) ;
#13958=LINE ( 'NONE', #23949, #28322 ) ;
#13962=PLANE ( 'NONE',  #25925 ) ;
#13963=CARTESIAN_POINT ( 'NONE',  ( -40.06503689199337259, 6.934220188908800431, 39.11858639832014717 ) ) ;
#13967=ORIENTED_EDGE ( 'NONE', *, *, #9944, .T. ) ;
#13970=DIRECTION ( 'NONE',  ( -0.8746197071393805311, 0.4848096202463645921, 1.277302113040265530E-17 ) ) ;
#13976=CARTESIAN_POINT ( 'NONE',  ( -41.51232591312490428, 10.75780884251261682, 36.23067884439899444 ) ) ;
#13992=FACE_BOUND ( 'NONE', #11984, .T. ) ;
#14001=LINE ( 'NONE', #23836, #23619 ) ;
#14005=EDGE_CURVE ( 'NONE', #8819, #7068, #4205, .T. ) ;
#14020=DIRECTION ( 'NONE',  ( 0.4848096202463673676, 0.8746197071393789768, 0.000000000000000000 ) ) ;
#14032=TOROIDAL_SURFACE ( 'NONE', #4069, 1.299999999999999822, 0.1000000000000000056 ) ;
#14035=EDGE_LOOP ( 'NONE', ( #6779, #31463, #10869, #8348 ) ) ;
#14046=EDGE_CURVE ( 'NONE', #16322, #30017, #27470, .T. ) ;
#14049=DIRECTION ( 'NONE',  ( -0.6184495258776595561, 0.3428121700606653888, -0.7071067811865444641 ) ) ;
#14055=ORIENTED_EDGE ( 'NONE', *, *, #21700, .T. ) ;
#14057=CARTESIAN_POINT ( 'NONE',  ( -40.89289694005993425, 10.41158093418393094, 36.52712545380572351 ) ) ;
#14058=ORIENTED_EDGE ( 'NONE', *, *, #21689, .F. ) ;
#14059=CARTESIAN_POINT ( 'NONE',  ( -43.68921302925062378, 1.179890886355840163, 39.44930799450052916 ) ) ;
#14060=DIRECTION ( 'NONE',  ( 0.8746197071393925215, -0.4848096202463429982, -8.676864087101708112E-18 ) ) ;
#14071=ADVANCED_FACE ( 'NONE', ( #2682 ), #372, .T. ) ;
#14072=DIRECTION ( 'NONE',  ( -1.188208965918164993E-16, -1.880121038077813132E-16, -1.000000000000000000 ) ) ;
#14078=CARTESIAN_POINT ( 'NONE',  ( -40.50800117262852496, 7.569618128341433660, 53.85120749494056724 ) ) ;
#14080=ORIENTED_EDGE ( 'NONE', *, *, #20200, .F. ) ;
#14081=VERTEX_POINT ( 'NONE', #32201 ) ;
#14085=CARTESIAN_POINT ( 'NONE',  ( -43.86882709718853590, -0.1754741395363378920, 32.14930799450051779 ) ) ;
#14086=DIRECTION ( 'NONE',  ( 0.2756373558170082672, -0.9612616959383162296, 0.000000000000000000 ) ) ;
#14088=CARTESIAN_POINT ( 'NONE',  ( -40.55615437192444261, 7.233232712785302887, 38.86959707880754422 ) ) ;
#14093=CIRCLE ( 'NONE', #4123, 0.1000000000000008243 ) ;
#14100=AXIS2_PLACEMENT_3D ( 'NONE', #16907, #17399, #24957 ) ;
#14103=ORIENTED_EDGE ( 'NONE', *, *, #12216, .F. ) ;
#14105=VERTEX_POINT ( 'NONE', #7251 ) ;
#14108=ORIENTED_EDGE ( 'NONE', *, *, #29621, .T. ) ;
#14119=DIRECTION ( 'NONE',  ( 0.000000000000000000, 0.000000000000000000, 1.000000000000000000 ) ) ;
#14127=CARTESIAN_POINT ( 'NONE',  ( -40.32034427004700916, 8.384459687302960873, 59.64930799450051779 ) ) ;
#14130=ORIENTED_EDGE ( 'NONE', *, *, #10654, .F. ) ;
#14140=ORIENTED_EDGE ( 'NONE', *, *, #29399, .F. ) ;
#14147=AXIS2_PLACEMENT_3D ( 'NONE', #1204, #3506, #16465 ) ;
#14150=FACE_OUTER_BOUND ( 'NONE', #2947, .T. ) ;
#14151=DIRECTION ( 'NONE',  ( -0.8746197071393926326, 0.4848096202463430537, 8.676864087101709653E-18 ) ) ;
#14155=ORIENTED_EDGE ( 'NONE', *, *, #14163, .T. ) ;
#14156=DIRECTION ( 'NONE',  ( 0.9612616959383193382, 0.2756373558169973870, 8.795445018804928853E-19 ) ) ;
#14158=DIRECTION ( 'NONE',  ( 0.3428121700606596711, 0.6184495258776487869, 0.7071067811865565655 ) ) ;
#14163=EDGE_CURVE ( 'NONE', #4559, #5569, #22984, .T. ) ;
#14173=ORIENTED_EDGE ( 'NONE', *, *, #25092, .T. ) ;
#14176=CARTESIAN_POINT ( 'NONE',  ( -41.02687597405218156, 7.220473278338834788, 53.54930799450051637 ) ) ;
#14184=DIRECTION ( 'NONE',  ( -0.8746197071393810862, 0.4848096202463637039, 8.676864087101942305E-18 ) ) ;
#14192=AXIS2_PLACEMENT_3D ( 'NONE', #26842, #9777, #19605 ) ;
#14204=ORIENTED_EDGE ( 'NONE', *, *, #16036, .T. ) ;
#14212=CARTESIAN_POINT ( 'NONE',  ( -42.66751614955960292, 15.14923148629343430, 38.44930799450052916 ) ) ;
#14213=CARTESIAN_POINT ( 'NONE',  ( -40.57832940339291383, 7.446916344587776848, 53.80788663826320573 ) ) ;
#14219=EDGE_LOOP ( 'NONE', ( #12708, #4671, #26368 ) ) ;
#14221=CARTESIAN_POINT ( 'NONE',  ( -40.06118906035626281, 6.942907937678607588, 34.99292058590180687 ) ) ;
#14226=LINE ( 'NONE', #24224, #3282 ) ;
#14231=EDGE_CURVE ( 'NONE', #28351, #10451, #25457, .T. ) ;
#14237=CARTESIAN_POINT ( 'NONE',  ( -41.73034863705382946, 11.48775164340967336, 56.04611646155296256 ) ) ;
#14240=CARTESIAN_POINT ( 'NONE',  ( -43.73393778030726509, 1.305471833569777695, 53.64930799450051779 ) ) ;
#14242=CARTESIAN_POINT ( 'NONE',  ( -40.50918210725697577, 7.581244431903962244, 53.87068005425620498 ) ) ;
#14248=CARTESIAN_POINT ( 'NONE',  ( -41.56848915456957627, 9.139695702668031885, 34.54930799450052348 ) ) ;
#14250=ORIENTED_EDGE ( 'NONE', *, *, #16847, .F. ) ;
#14253=FACE_OUTER_BOUND ( 'NONE', #17070, .T. ) ;
#14254=DIRECTION ( 'NONE',  ( 0.9612616959383200044, 0.2756373558169954996, -1.660411357259285896E-16 ) ) ;
#14255=DIRECTION ( 'NONE',  ( 0.000000000000000000, 0.000000000000000000, -1.000000000000000000 ) ) ;
#14266=AXIS2_PLACEMENT_3D ( 'NONE', #31954, #31789, #3893 ) ;
#14268=CARTESIAN_POINT ( 'NONE',  ( -43.86882709718853590, -0.1754741395363378920, 32.04930799450052348 ) ) ;
#14286=DIRECTION ( 'NONE',  ( 0.4848096202463424986, 0.8746197071393928546, -2.220446049250312834E-16 ) ) ;
#14292=CARTESIAN_POINT ( 'NONE',  ( -40.21210701746133509, 7.644196001419694575, 60.24930799450051211 ) ) ;
#14295=ORIENTED_EDGE ( 'NONE', *, *, #2271, .T. ) ;
#14302=DIRECTION ( 'NONE',  ( 0.3958453973320081309, 0.7141240004913237405, 0.5773502691896250649 ) ) ;
#14312=EDGE_CURVE ( 'NONE', #7978, #1764, #13958, .T. ) ;
#14321=LINE ( 'NONE', #1998, #10400 ) ;
#14324=DIRECTION ( 'NONE',  ( -0.4848096202463655358, -0.8746197071393799760, 0.000000000000000000 ) ) ;
#14325=CARTESIAN_POINT ( 'NONE',  ( -39.44363481821952178, 3.888719912690143499, 37.04930799450052348 ) ) ;
#14334=FACE_OUTER_BOUND ( 'NONE', #15152, .T. ) ;
#14336=FACE_OUTER_BOUND ( 'NONE', #7025, .T. ) ;
#14339=DIRECTION ( 'NONE',  ( -0.9612616959383221138, -0.2756373558169876170, 0.000000000000000000 ) ) ;
#14345=SPHERICAL_SURFACE ( 'NONE', #9951, 0.1000000000000000056 ) ;
#14352=EDGE_LOOP ( 'NONE', ( #19500, #32151, #29005 ) ) ;
#14369=CARTESIAN_POINT ( 'NONE',  ( -40.64500813507293486, 6.819128862114092193, 39.51928662074344345 ) ) ;
#14370=ORIENTED_EDGE ( 'NONE', *, *, #11216, .T. ) ;
#14371=FACE_BOUND ( 'NONE', #15996, .T. ) ;
#14374=CARTESIAN_POINT ( 'NONE',  ( -38.05567176388107242, 15.54312433976834740, 59.54930799450050927 ) ) ;
#14380=ORIENTED_EDGE ( 'NONE', *, *, #2358, .F. ) ;
#14382=EDGE_CURVE ( 'NONE', #23429, #4508, #31518, .T. ) ;
#14384=ORIENTED_EDGE ( 'NONE', *, *, #17453, .F. ) ;
#14389=CIRCLE ( 'NONE', #10198, 1.003191532947550701 ) ;
#14392=ADVANCED_FACE ( 'NONE', ( #26744 ), #16559, .T. ) ;
#14393=TOROIDAL_SURFACE ( 'NONE', #753, 0.2000000000000000111, 0.1000000000000000056 ) ;
#14397=ORIENTED_EDGE ( 'NONE', *, *, #28675, .F. ) ;
#14411=LINE ( 'NONE', #24412, #27256 ) ;
#14415=CARTESIAN_POINT ( 'NONE',  ( -40.02540636251514172, 2.839176264122877047, 57.04930799450051637 ) ) ;
#14420=FACE_OUTER_BOUND ( 'NONE', #11982, .T. ) ;
#14423=CARTESIAN_POINT ( 'NONE',  ( -40.61178118339597631, 9.038025460530262123, 56.14611646155296398 ) ) ;
#14430=ORIENTED_EDGE ( 'NONE', *, *, #18409, .T. ) ;
#14439=CARTESIAN_POINT ( 'NONE',  ( -39.31817303416426768, 4.733858564475560193, 37.04930799450052348 ) ) ;
#14454=EDGE_CURVE ( 'NONE', #22782, #4744, #12085, .T. ) ;
#14455=CARTESIAN_POINT ( 'NONE',  ( -40.64160980462626327, 6.824069488939677797, 34.67994969264233163 ) ) ;
#14457=DIRECTION ( 'NONE',  ( 0.9612616959383207815, 0.2756373558169927240, 8.795445018804291370E-19 ) ) ;
#14460=VERTEX_POINT ( 'NONE', #5364 ) ;
#14463=DIRECTION ( 'NONE',  ( 0.2756373558170018279, -0.9612616959383181170, 0.000000000000000000 ) ) ;
#14470=DIRECTION ( 'NONE',  ( -0.4848096202463673121, -0.8746197071393789768, 0.000000000000000000 ) ) ;
#14477=EDGE_LOOP ( 'NONE', ( #21349, #18113, #77, #9555, #26898, #615, #30788 ) ) ;
#14479=FACE_OUTER_BOUND ( 'NONE', #1648, .T. ) ;
#14480=DIRECTION ( 'NONE',  ( -0.1949050434465282311, 0.6797146636928673713, -0.7071067811865470176 ) ) ;
#14482=ORIENTED_EDGE ( 'NONE', *, *, #8992, .F. ) ;
#14483=CARTESIAN_POINT ( 'NONE',  ( -40.11286833322907341, 2.887657226147507306, 37.04930799450052348 ) ) ;
#14484=CARTESIAN_POINT ( 'NONE',  ( -43.37834615508418068, 1.121909970995876193, 34.64930799450052490 ) ) ;
#14485=ADVANCED_FACE ( 'NONE', ( #19508 ), #29540, .T. ) ;
#14493=FACE_OUTER_BOUND ( 'NONE', #1897, .T. ) ;
#14498=ADVANCED_FACE ( 'NONE', ( #7043 ), #17048, .T. ) ;
#14500=VECTOR ( 'NONE', #1715, 1000.000000000000114 ) ;
#14501=CARTESIAN_POINT ( 'NONE',  ( -41.02687597405218156, 7.220473278338834788, 53.64930799450051779 ) ) ;
#14504=CARTESIAN_POINT ( 'NONE',  ( -40.11967773290336226, 9.763195579837789850, 38.54930799450052348 ) ) ;
#14507=VERTEX_POINT ( 'NONE', #17653 ) ;
#14508=FACE_OUTER_BOUND ( 'NONE', #21913, .T. ) ;
#14510=DIRECTION ( 'NONE',  ( -0.4848096202463429427, -0.8746197071393925215, 2.352477780477436787E-16 ) ) ;
#14522=DIRECTION ( 'NONE',  ( -0.8746197071393790878, 0.4848096202463673676, 1.277302113040196197E-17 ) ) ;
#14528=PLANE ( 'NONE',  #20718 ) ;
#14530=CARTESIAN_POINT ( 'NONE',  ( -43.82034613516389498, -0.08801216882239806805, 62.04930799450052348 ) ) ;
#14533=DIRECTION ( 'NONE',  ( 1.188208965918165239E-16, 1.880121038077813132E-16, 1.000000000000000000 ) ) ;
#14535=EDGE_CURVE ( 'NONE', #1830, #25211, #101, .T. ) ;
#14538=CARTESIAN_POINT ( 'NONE',  ( -40.73091736380679606, 9.483895492497156354, 35.44930799450052206 ) ) ;
#14540=CARTESIAN_POINT ( 'NONE',  ( -40.02327307428360115, 7.071123406434916880, 34.89423478111014276 ) ) ;
#14542=ORIENTED_EDGE ( 'NONE', *, *, #3362, .T. ) ;
#14546=PRODUCT ( 'Terminals', 'Terminals', '', ( #12486 ) ) ;
#14547=( BOUNDED_CURVE ( )  B_SPLINE_CURVE ( 3, ( #9646, #14567, #24571, #4718 ),
 .UNSPECIFIED., .F., .F. ) 
 B_SPLINE_CURVE_WITH_KNOTS ( ( 4, 4 ),
 ( 5.497787143782102426, 6.283185307179586232 ),
 .UNSPECIFIED. ) 
 CURVE ( )  GEOMETRIC_REPRESENTATION_ITEM ( )  RATIONAL_B_SPLINE_CURVE ( ( 1.000000000000000000, 0.9492530216741865701, 0.9492530216741865701, 1.000000000000000000 ) ) 
 REPRESENTATION_ITEM ( '' )  );
#14548=EDGE_LOOP ( 'NONE', ( #30499, #22704, #7629, #31981, #14103, #8647 ) ) ;
#14553=DIRECTION ( 'NONE',  ( -0.4848096202463431648, -0.8746197071393924105, 0.000000000000000000 ) ) ;
#14555=AXIS2_PLACEMENT_3D ( 'NONE', #18296, #23550, #20922 ) ;
#14556=VERTEX_POINT ( 'NONE', #27841 ) ;
#14560=DIRECTION ( 'NONE',  ( 0.4848096202463489934, 0.8746197071393893019, 9.920727850367968435E-18 ) ) ;
#14567=CARTESIAN_POINT ( 'NONE',  ( -40.67837904183829068, 9.488261090400161635, 34.65356819842892833 ) ) ;
#14568=CARTESIAN_POINT ( 'NONE',  ( -40.11286833322908052, 2.887657226147511302, 57.04930799450051637 ) ) ;
#14578=ADVANCED_FACE ( 'NONE', ( #13549 ), #28640, .T. ) ;
#14581=CARTESIAN_POINT ( 'NONE',  ( -40.12405407910454613, 7.699914440225940737, 60.22001867261916885 ) ) ;
#14584=FACE_OUTER_BOUND ( 'NONE', #20323, .T. ) ;
#14586=VERTEX_POINT ( 'NONE', #26010 ) ;
#14587=AXIS2_PLACEMENT_3D ( 'NONE', #21136, #11632, #16540 ) ;
#14596=LINE ( 'NONE', #22451, #16541 ) ;
#14605=DIRECTION ( 'NONE',  ( 0.2756373558169954441, -0.9612616959383198934, 1.479773560108263204E-16 ) ) ;
#14618=ORIENTED_EDGE ( 'NONE', *, *, #25398, .F. ) ;
#14621=LINE ( 'NONE', #21986, #1521 ) ;
#14622=ORIENTED_EDGE ( 'NONE', *, *, #7011, .T. ) ;
#14625=ORIENTED_EDGE ( 'NONE', *, *, #30850, .F. ) ;
#14634=CIRCLE ( 'NONE', #29865, 0.1000000000000006301 ) ;
#14637=DIRECTION ( 'NONE',  ( 0.8746197071393925215, -0.4848096202463429982, -8.676864087101708112E-18 ) ) ;
#14641=ADVANCED_FACE ( 'NONE', ( #15681 ), #6171, .T. ) ;
#14645=CARTESIAN_POINT ( 'NONE',  ( -40.58856461370174884, 7.499380836222963254, 60.14930799450051779 ) ) ;
#14646=CARTESIAN_POINT ( 'NONE',  ( -40.09211399732166115, 9.667069410243957606, 35.44930799450052206 ) ) ;
#14651=CYLINDRICAL_SURFACE ( 'NONE', #18456, 2.000000000000001776 ) ;
#14655=DIRECTION ( 'NONE',  ( 0.4848096202463429982, 0.8746197071393925215, 9.920727850371698576E-18 ) ) ;
#14658=CARTESIAN_POINT ( 'NONE',  ( -40.59783130604490253, 7.538194345349025660, 53.99315859930123906 ) ) ;
#14678=VECTOR ( 'NONE', #23202, 1000.000000000000000 ) ;
#14685=ORIENTED_EDGE ( 'NONE', *, *, #2230, .F. ) ;
#14687=AXIS2_PLACEMENT_3D ( 'NONE', #27606, #12692, #10374 ) ;
#14688=DIRECTION ( 'NONE',  ( -0.2756373558169973870, 0.9612616959383193382, 1.315048337272770280E-17 ) ) ;
#14692=CARTESIAN_POINT ( 'NONE',  ( -40.75223430975736960, 8.437483520745759691, 34.54930799450052348 ) ) ;
#14694=CARTESIAN_POINT ( 'NONE',  ( -41.01929587258828747, 9.401204285752060130, 35.44930799450052206 ) ) ;
#14698=DIRECTION ( 'NONE',  ( 0.2756373558169828430, -0.9612616959383236681, 1.479773560108285391E-16 ) ) ;
#14702=CARTESIAN_POINT ( 'NONE',  ( -40.15599670534037102, 7.478908884098768084, 39.44930799450052206 ) ) ;
#14705=CARTESIAN_POINT ( 'NONE',  ( -40.62123369608615775, 7.650200974017423938, 39.54930799450052348 ) ) ;
#14706=ORIENTED_EDGE ( 'NONE', *, *, #18728, .F. ) ;
#14713=ORIENTED_EDGE ( 'NONE', *, *, #2586, .T. ) ;
#14715=CIRCLE ( 'NONE', #5735, 0.1000000000000018235 ) ;
#14716=AXIS2_PLACEMENT_3D ( 'NONE', #12693, #27607, #13335 ) ;
#14722=VERTEX_POINT ( 'NONE', #21887 ) ;
#14729=AXIS2_PLACEMENT_3D ( 'NONE', #14646, #31717, #7257 ) ;
#14732=ORIENTED_EDGE ( 'NONE', *, *, #10087, .T. ) ;
#14737=DIRECTION ( 'NONE',  ( 0.2756373558170128191, -0.9612616959383148973, 0.000000000000000000 ) ) ;
#14738=DIRECTION ( 'NONE',  ( 0.4848096202463430537, 0.8746197071393926326, 9.920727850371700117E-18 ) ) ;
#14741=CARTESIAN_POINT ( 'NONE',  ( -41.74593813222361405, 15.43463958587387808, 38.54930799450052348 ) ) ;
#14747=B_SPLINE_CURVE_WITH_KNOTS ( 'NONE', 3,
 ( #18739, #26144, #21361, #31245 ),
 .UNSPECIFIED., .F., .F.,
 ( 4, 4 ),
 ( 0.000000000000000000, 0.0001556073905087536054 ),
 .UNSPECIFIED. ) ;
#14752=CARTESIAN_POINT ( 'NONE',  ( -40.50726676055796105, 7.559560307024983494, 53.54930799450051637 ) ) ;
#14753=VERTEX_POINT ( 'NONE', #29458 ) ;
#14756=ORIENTED_EDGE ( 'NONE', *, *, #28648, .F. ) ;
#14761=EDGE_CURVE ( 'NONE', #28974, #11047, #27661, .T. ) ;
#14762=ORIENTED_EDGE ( 'NONE', *, *, #28637, .F. ) ;
#14763=EDGE_CURVE ( 'NONE', #22939, #5375, #18725, .T. ) ;
#14765=DIRECTION ( 'NONE',  ( 0.8746197071393858602, -0.4848096202463547666, 0.000000000000000000 ) ) ;
#14770=CARTESIAN_POINT ( 'NONE',  ( -42.21195563036362586, 4.051200314738734320, 57.04930799450051637 ) ) ;
#14773=ORIENTED_EDGE ( 'NONE', *, *, #22337, .F. ) ;
#14776=EDGE_LOOP ( 'NONE', ( #4498, #18876, #9023, #29202 ) ) ;
#14780=CARTESIAN_POINT ( 'NONE',  ( -40.69503817910143084, 6.787791837620303248, 34.66137507890927338 ) ) ;
#14781=AXIS2_PLACEMENT_3D ( 'NONE', #24174, #28781, #6782 ) ;
#14782=CYLINDRICAL_SURFACE ( 'NONE', #3159, 0.1000000000000006301 ) ;
#14786=EDGE_LOOP ( 'NONE', ( #20954, #8324, #24460, #24185 ) ) ;
#14787=CARTESIAN_POINT ( 'NONE',  ( -36.59542768321662720, 12.56771722797891400, 37.04930799450052348 ) ) ;
#14795=FACE_OUTER_BOUND ( 'NONE', #11356, .T. ) ;
#14803=AXIS2_PLACEMENT_3D ( 'NONE', #12128, #19496, #24586 ) ;
#14804=VERTEX_POINT ( 'NONE', #12723 ) ;
#14816=FACE_BOUND ( 'NONE', #27753, .T. ) ;
#14828=CARTESIAN_POINT ( 'NONE',  ( -40.17244512953781310, 6.931285263614340053, 34.54930799450052348 ) ) ;
#14833=DIRECTION ( 'NONE',  ( -2.779292025043186357E-18, 1.288349127009862211E-17, -1.000000000000000000 ) ) ;
#14835=ORIENTED_EDGE ( 'NONE', *, *, #10656, .F. ) ;
#14837=DIRECTION ( 'NONE',  ( 0.000000000000000000, 0.000000000000000000, -1.000000000000000000 ) ) ;
#14838=CARTESIAN_POINT ( 'NONE',  ( -42.37913764077812573, 15.23192269303853053, 35.64930799450052490 ) ) ;
#14840=ADVANCED_FACE ( 'NONE', ( #9763 ), #5327, .T. ) ;
#14848=FACE_OUTER_BOUND ( 'NONE', #12601, .T. ) ;
#14849=ORIENTED_EDGE ( 'NONE', *, *, #3204, .T. ) ;
#14853=DIRECTION ( 'NONE',  ( -0.8746197071393925215, 0.4848096202463429982, 8.676864087101708112E-18 ) ) ;
#14862=CARTESIAN_POINT ( 'NONE',  ( -42.22510282758591416, 14.66434666503944051, 60.54930799450051637 ) ) ;
#14864=EDGE_CURVE ( 'NONE', #28859, #32358, #20401, .T. ) ;
#14865=DIRECTION ( 'NONE',  ( 0.9612616959383221138, 0.2756373558169876170, 0.000000000000000000 ) ) ;
#14875=EDGE_CURVE ( 'NONE', #3250, #16822, #28198, .T. ) ;
#14877=VERTEX_POINT ( 'NONE', #21196 ) ;
#14878=VECTOR ( 'NONE', #4290, 1000.000000000000114 ) ;
#14882=AXIS2_PLACEMENT_3D ( 'NONE', #23893, #1404, #1179 ) ;
#14885=EDGE_LOOP ( 'NONE', ( #23888, #11907, #16811 ) ) ;
#14887=AXIS2_PLACEMENT_3D ( 'NONE', #13897, #11421, #21415 ) ;
#14902=CARTESIAN_POINT ( 'NONE',  ( -41.55884944519204538, 7.292100401678685451, 39.54930799450052348 ) ) ;
#14903=CARTESIAN_POINT ( 'NONE',  ( -40.58856461370174884, 7.499380836222963254, 60.14930799450051779 ) ) ;
#14906=CARTESIAN_POINT ( 'NONE',  ( -40.11729073372970333, 6.802967823440400075, 34.64930799450051779 ) ) ;
#14912=EDGE_CURVE ( 'NONE', #16822, #5228, #22446, .T. ) ;
#14916=ORIENTED_EDGE ( 'NONE', *, *, #5190, .F. ) ;
#14926=( BOUNDED_SURFACE ( )  B_SPLINE_SURFACE ( 3, 2, ( 
 ( #23227, #15841, #20761 ),
 ( #5839, #25844, #21383 ),
 ( #31746, #26648, #23542 ),
 ( #3512, #4004, #6791 ) ),
 .UNSPECIFIED., .F., .F., .F. ) 
 B_SPLINE_SURFACE_WITH_KNOTS ( ( 4, 4 ),
 ( 3, 3 ),
 ( 1.570796326794896558, 1.630650672327996542 ),
 ( 0.000000000000000000, 1.000000000000000000 ),
 .UNSPECIFIED. ) 
 GEOMETRIC_REPRESENTATION_ITEM ( )  RATIONAL_B_SPLINE_SURFACE ( (
 ( 1.000000000000000000, 0.7071067811865515695, 1.000000000000000000),
 ( 1.000000000000000000, 0.7120946502353932006, 1.000000000000000000),
 ( 1.000000000000000000, 0.7170297040967722468, 1.000000000000000000),
 ( 1.000000000000000000, 0.7219065546282052992, 1.000000000000000000) ) ) 
 REPRESENTATION_ITEM ( '' )  SURFACE ( )  );
#14933=DIRECTION ( 'NONE',  ( 0.2756373558169974980, -0.9612616959383193382, -1.315048337272770589E-17 ) ) ;
#14934=AXIS2_PLACEMENT_3D ( 'NONE', #7570, #20192, #32026 ) ;
#14936=DIRECTION ( 'NONE',  ( 0.4848096202463429427, 0.8746197071393925215, -2.352477780477436787E-16 ) ) ;
#14939=DIRECTION ( 'NONE',  ( 0.7848668881104262640, 0.2250569586005336520, -0.5773502691896258421 ) ) ;
#14948=EDGE_CURVE ( 'NONE', #1830, #12799, #22487, .T. ) ;
#14951=ADVANCED_FACE ( 'NONE', ( #8735 ), #30754, .T. ) ;
#14959=AXIS2_PLACEMENT_3D ( 'NONE', #15571, #20660, #30529 ) ;
#14962=VECTOR ( 'NONE', #14853, 1000.000000000000114 ) ;
#14972=LINE ( 'NONE', #24974, #384 ) ;
#14975=DIRECTION ( 'NONE',  ( -0.2756373558169961102, 0.9612616959383197823, 0.000000000000000000 ) ) ;
#14977=DIRECTION ( 'NONE',  ( -0.8746197071393925215, 0.4848096202463429982, 8.676864087101709653E-18 ) ) ;
#14980=LINE ( 'NONE', #12024, #13725 ) ;
#14981=ORIENTED_EDGE ( 'NONE', *, *, #1582, .T. ) ;
#14986=CIRCLE ( 'NONE', #3368, 0.1000000000000018235 ) ;
#14995=ORIENTED_EDGE ( 'NONE', *, *, #26483, .F. ) ;
#14997=CARTESIAN_POINT ( 'NONE',  ( -40.13633318854532916, 6.906174383240057502, 39.54018667097405171 ) ) ;
#15012=EDGE_CURVE ( 'NONE', #10259, #1803, #17196, .T. ) ;
#15014=AXIS2_PLACEMENT_3D ( 'NONE', #22377, #19919, #17463 ) ;
#15021=LINE ( 'NONE', #25509, #8698 ) ;
#15024=SPHERICAL_SURFACE ( 'NONE', #7423, 0.1000000000000000056 ) ;
#15030=CARTESIAN_POINT ( 'NONE',  ( -48.25869185997735400, 10.94158050198885590, 54.56265170360538264 ) ) ;
#15035=FACE_OUTER_BOUND ( 'NONE', #6950, .T. ) ;
#15037=CARTESIAN_POINT ( 'NONE',  ( -40.73728033978215990, 8.177846351970792682, 54.53299432381886191 ) ) ;
#15039=VECTOR ( 'NONE', #14480, 1000.000000000000000 ) ;
#15043=DIRECTION ( 'NONE',  ( 0.8746197071393926326, -0.4848096202463430537, -8.676864087101709653E-18 ) ) ;
#15044=EDGE_CURVE ( 'NONE', #12276, #27773, #1994, .T. ) ;
#15045=EDGE_CURVE ( 'NONE', #29138, #11711, #9359, .T. ) ;
#15046=ORIENTED_EDGE ( 'NONE', *, *, #26449, .F. ) ;
#15049=DIRECTION ( 'NONE',  ( -0.8746197071393858602, 0.4848096202463547666, 0.000000000000000000 ) ) ;
#15057=DIRECTION ( 'NONE',  ( -0.3428121700606640565, -0.6184495258776567805, 0.7071067811865474617 ) ) ;
#15060=CARTESIAN_POINT ( 'NONE',  ( -40.50146157965988891, 7.595301493077381672, 35.43807061034478778 ) ) ;
#15066=CARTESIAN_POINT ( 'NONE',  ( -42.22138300640814634, 14.68176690255378425, 38.09144330556765112 ) ) ;
#15069=EDGE_CURVE ( 'NONE', #21033, #1586, #14321, .T. ) ;
#15080=EDGE_CURVE ( 'NONE', #19002, #25278, #1673, .T. ) ;
#15084=EDGE_CURVE ( 'NONE', #16834, #14804, #16598, .T. ) ;
#15085=ORIENTED_EDGE ( 'NONE', *, *, #11095, .F. ) ;
#15096=CARTESIAN_POINT ( 'NONE',  ( -40.47579404106498657, 7.230063580211345986, 35.21320777407684233 ) ) ;
#15100=CARTESIAN_POINT ( 'NONE',  ( -40.80097511801616150, 8.246641009394465982, 54.64930799450051779 ) ) ;
#15105=CARTESIAN_POINT ( 'NONE',  ( -40.67837904183828357, 9.488261090400158082, 38.64504779057212147 ) ) ;
#15115=AXIS2_PLACEMENT_3D ( 'NONE', #13478, #1308, #13325 ) ;
#15116=CIRCLE ( 'NONE', #25605, 0.7928932188134565351 ) ;
#15119=( BOUNDED_CURVE ( )  B_SPLINE_CURVE ( 3, ( #23414, #23090, #13417, #2748 ),
 .UNSPECIFIED., .F., .F. ) 
 B_SPLINE_CURVE_WITH_KNOTS ( ( 4, 4 ),
 ( 1.510941981261797462, 1.570796326794904774 ),
 .UNSPECIFIED. ) 
 CURVE ( )  GEOMETRIC_REPRESENTATION_ITEM ( )  RATIONAL_B_SPLINE_CURVE ( ( 1.000000000000000000, 0.9997014770583808607, 0.9997014770583808607, 1.000000000000000000 ) ) 
 REPRESENTATION_ITEM ( '' )  );
#15122=DIRECTION ( 'NONE',  ( 0.2756373558169974980, -0.9612616959383193382, -1.315048337272770589E-17 ) ) ;
#15131=CARTESIAN_POINT ( 'NONE',  ( -42.48853158357926674, 14.65761848575743898, 55.12990477204974837 ) ) ;
#15135=DIRECTION ( 'NONE',  ( 1.188208965918164993E-16, 1.880121038077812639E-16, 1.000000000000000000 ) ) ;
#15136=CARTESIAN_POINT ( 'NONE',  ( -43.95628906790246759, -0.1269931775117038586, 32.14930799450051779 ) ) ;
#15141=ORIENTED_EDGE ( 'NONE', *, *, #1074, .F. ) ;
#15142=CYLINDRICAL_SURFACE ( 'NONE', #10301, 2.000000000000001776 ) ;
#15152=EDGE_LOOP ( 'NONE', ( #30000, #23019, #28234, #10389 ) ) ;
#15157=VECTOR ( 'NONE', #31853, 1000.000000000000114 ) ;
#15164=EDGE_CURVE ( 'NONE', #6754, #20995, #9335, .T. ) ;
#15165=EDGE_CURVE ( 'NONE', #12276, #32106, #9875, .T. ) ;
#15173=CARTESIAN_POINT ( 'NONE',  ( -48.34557642001920641, 3.861744873591483440, 60.54930799450051637 ) ) ;
#15176=LINE ( 'NONE', #6973, #5860 ) ;
#15178=EDGE_LOOP ( 'NONE', ( #18122, #12462, #22930, #22560 ) ) ;
#15181=DIRECTION ( 'NONE',  ( -0.9612616959383206705, -0.2756373558169934457, 1.660411357259282938E-16 ) ) ;
#15182=CARTESIAN_POINT ( 'NONE',  ( -40.60333149162104860, 7.557375771971046596, 59.44930799450051495 ) ) ;
#15184=EDGE_LOOP ( 'NONE', ( #13513, #14995, #10388, #20521 ) ) ;
#15186=DIRECTION ( 'NONE',  ( 0.2756373558169942228, -0.9612616959383203374, 0.000000000000000000 ) ) ;
#15188=CYLINDRICAL_SURFACE ( 'NONE', #18330, 0.9999999999999998890 ) ;
#15191=VECTOR ( 'NONE', #26486, 1000.000000000000114 ) ;
#15192=DIRECTION ( 'NONE',  ( -0.8746197071393926326, 0.4848096202463430537, 8.676864087101709653E-18 ) ) ;
#15195=ORIENTED_EDGE ( 'NONE', *, *, #9078, .F. ) ;
#15204=EDGE_CURVE ( 'NONE', #24463, #21157, #12254, .T. ) ;
#15205=AXIS2_PLACEMENT_3D ( 'NONE', #13212, #17951, #2852 ) ;
#15209=CARTESIAN_POINT ( 'NONE',  ( -40.59758774925371938, 7.567737757495683226, 38.66054537865625917 ) ) ;
#15219=AXIS2_PLACEMENT_3D ( 'NONE', #959, #18351, #28381 ) ;
#15224=VECTOR ( 'NONE', #26141, 1000.000000000000000 ) ;
#15225=CARTESIAN_POINT ( 'NONE',  ( -41.77464577679392477, 3.808795504615562155, 47.04930799450051637 ) ) ;
#15226=DIRECTION ( 'NONE',  ( -0.9612616959383204485, -0.2756373558169933347, 1.660411357259282692E-16 ) ) ;
#15227=EDGE_CURVE ( 'NONE', #1884, #286, #3562, .T. ) ;
#15235=DIRECTION ( 'NONE',  ( 0.000000000000000000, 0.000000000000000000, 1.000000000000000000 ) ) ;
#15236=ORIENTED_EDGE ( 'NONE', *, *, #16443, .T. ) ;
#15237=VERTEX_POINT ( 'NONE', #14645 ) ;
#15242=AXIS2_PLACEMENT_3D ( 'NONE', #21096, #3542, #13567 ) ;
#15245=CIRCLE ( 'NONE', #2153, 1.142135311067127512 ) ;
#15249=VERTEX_POINT ( 'NONE', #2810 ) ;
#15266=CYLINDRICAL_SURFACE ( 'NONE', #27587, 1.042135311067126979 ) ;
#15272=TOROIDAL_SURFACE ( 'NONE', #1101, 1.299999999999999822, 0.1000000000000000056 ) ;
#15274=DIRECTION ( 'NONE',  ( -0.8746197071393926326, 0.4848096202463430537, 8.676864087101709653E-18 ) ) ;
#15280=LINE ( 'NONE', #8061, #29606 ) ;
#15282=AXIS2_PLACEMENT_3D ( 'NONE', #21777, #31484, #26230 ) ;
#15291=DIRECTION ( 'NONE',  ( 0.8746197071393926326, -0.4848096202463430537, -8.676864087101709653E-18 ) ) ;
#15295=FACE_OUTER_BOUND ( 'NONE', #26872, .T. ) ;
#15296=PLANE ( 'NONE',  #7465 ) ;
#15299=LINE ( 'NONE', #17590, #28835 ) ;
#15300=ADVANCED_FACE ( 'NONE', ( #17419 ), #5285, .T. ) ;
#15303=ORIENTED_EDGE ( 'NONE', *, *, #15080, .T. ) ;
#15306=AXIS2_PLACEMENT_3D ( 'NONE', #3054, #15868, #17835 ) ;
#15310=ORIENTED_EDGE ( 'NONE', *, *, #848, .T. ) ;
#15314=ORIENTED_EDGE ( 'NONE', *, *, #26002, .T. ) ;
#15315=ORIENTED_EDGE ( 'NONE', *, *, #21512, .F. ) ;
#15320=AXIS2_PLACEMENT_3D ( 'NONE', #877, #8438, #18431 ) ;
#15323=ORIENTED_EDGE ( 'NONE', *, *, #28209, .F. ) ;
#15324=CIRCLE ( 'NONE', #30516, 1.003191532947550701 ) ;
#15329=DIRECTION ( 'NONE',  ( 0.2756373558170082672, -0.9612616959383162296, 6.938893903907184201E-14 ) ) ;
#15332=VERTEX_POINT ( 'NONE', #32205 ) ;
#15333=EDGE_LOOP ( 'NONE', ( #4421, #17829, #13183, #29276 ) ) ;
#15339=VERTEX_POINT ( 'NONE', #9721 ) ;
#15342=DIRECTION ( 'NONE',  ( 0.9612616959383200044, 0.2756373558169954996, -1.660411357259285896E-16 ) ) ;
#15343=LINE ( 'NONE', #23213, #18894 ) ;
#15348=CARTESIAN_POINT ( 'NONE',  ( -43.38408989745150990, 1.111547985471240674, 53.54930799450051637 ) ) ;
#15353=ADVANCED_FACE ( 'NONE', ( #27271 ), #19876, .T. ) ;
#15358=EDGE_CURVE ( 'NONE', #10259, #11316, #9878, .T. ) ;
#15359=DIRECTION ( 'NONE',  ( -0.1949050434465282311, 0.6797146636928673713, -0.7071067811865470176 ) ) ;
#15369=AXIS2_PLACEMENT_3D ( 'NONE', #16653, #1238, #9119 ) ;
#15371=LINE ( 'NONE', #25379, #18565 ) ;
#15374=DIRECTION ( 'NONE',  ( 0.03087013654144268177, -0.1076569600579695002, -0.9937087166876366062 ) ) ;
#15384=DIRECTION ( 'NONE',  ( -0.8746197071393926326, 0.4848096202463430537, 8.676864087101709653E-18 ) ) ;
#15389=DIRECTION ( 'NONE',  ( 7.588956326749211550E-18, -4.206627182996911684E-18, 1.000000000000000000 ) ) ;
#15394=CARTESIAN_POINT ( 'NONE',  ( -43.69495677161796010, 1.169528900831203311, 60.54930799450051637 ) ) ;
#15396=VERTEX_POINT ( 'NONE', #12998 ) ;
#15401=ORIENTED_EDGE ( 'NONE', *, *, #5389, .F. ) ;
#15406=DIRECTION ( 'NONE',  ( 2.779292025043186357E-18, -1.288349127009862211E-17, 1.000000000000000000 ) ) ;
#15407=ORIENTED_EDGE ( 'NONE', *, *, #20700, .T. ) ;
#15408=DIRECTION ( 'NONE',  ( 0.1949050434465268156, -0.6797146636928678154, -0.7071067811865469066 ) ) ;
#15409=DIRECTION ( 'NONE',  ( 0.2756373558169973870, -0.9612616959383193382, -1.315048337272770435E-17 ) ) ;
#15419=CARTESIAN_POINT ( 'NONE',  ( -40.68879370032182408, 6.799057175545497600, 34.73625888416037810 ) ) ;
#15428=ORIENTED_EDGE ( 'NONE', *, *, #25972, .T. ) ;
#15431=EDGE_CURVE ( 'NONE', #110, #32358, #10535, .T. ) ;
#15432=DIRECTION ( 'NONE',  ( 0.2756373558169973870, -0.9612616959383193382, -1.315048337272770280E-17 ) ) ;
#15437=EDGE_CURVE ( 'NONE', #13254, #31739, #16911, .T. ) ;
#15438=AXIS2_PLACEMENT_3D ( 'NONE', #17825, #5198, #12597 ) ;
#15439=DIRECTION ( 'NONE',  ( 0.4848096202463430537, 0.8746197071393926326, -1.125439520643636483E-16 ) ) ;
#15440=CARTESIAN_POINT ( 'NONE',  ( -40.65487266620045403, 9.475231293617264683, 35.46144002885649371 ) ) ;
#15443=AXIS2_PLACEMENT_3D ( 'NONE', #25445, #2798, #12824 ) ;
#15445=AXIS2_PLACEMENT_3D ( 'NONE', #30553, #15439, #17733 ) ;
#15446=ORIENTED_EDGE ( 'NONE', *, *, #6155, .T. ) ;
#15455=DIRECTION ( 'NONE',  ( 0.4848096202463424431, 0.8746197071393927436, -2.220446049250312588E-16 ) ) ;
#15462=DIRECTION ( 'NONE',  ( 0.2756373558169961102, -0.9612616959383197823, 0.000000000000000000 ) ) ;
#15468=CARTESIAN_POINT ( 'NONE',  ( -40.22853490217745076, 6.951940700334886536, 39.38237851325574468 ) ) ;
#15476=AXIS2_PLACEMENT_3D ( 'NONE', #2701, #23036, #724 ) ;
#15481=EDGE_CURVE ( 'NONE', #29530, #20511, #6425, .T. ) ;
#15484=ORIENTED_EDGE ( 'NONE', *, *, #3031, .F. ) ;
#15486=LINE ( 'NONE', #28448, #20147 ) ;
#15487=DIRECTION ( 'NONE',  ( 0.9612616959383194493, 0.2756373558169974980, 8.795445018804946186E-19 ) ) ;
#15493=CYLINDRICAL_SURFACE ( 'NONE', #19081, 0.1000000000000006301 ) ;
#15495=EDGE_CURVE ( 'NONE', #28351, #16288, #16158, .T. ) ;
#15496=DIRECTION ( 'NONE',  ( -0.2756373558169973870, 0.9612616959383193382, 1.315048337272770280E-17 ) ) ;
#15499=CARTESIAN_POINT ( 'NONE',  ( -40.69234404896523216, 6.790679892791737338, 39.46310372540604305 ) ) ;
#15500=ORIENTED_EDGE ( 'NONE', *, *, #3631, .F. ) ;
#15507=ORIENTED_EDGE ( 'NONE', *, *, #9440, .F. ) ;
#15512=CARTESIAN_POINT ( 'NONE',  ( -38.41701585771487260, 6.978388747684010518, 62.04930799450052348 ) ) ;
#15517=ORIENTED_EDGE ( 'NONE', *, *, #27838, .T. ) ;
#15521=CARTESIAN_POINT ( 'NONE',  ( -41.02113223168485234, 7.230835263863471418, 34.64930799450051779 ) ) ;
#15537=ORIENTED_EDGE ( 'NONE', *, *, #8224, .T. ) ;
#15540=FACE_OUTER_BOUND ( 'NONE', #11273, .T. ) ;
#15544=CARTESIAN_POINT ( 'NONE',  ( -41.77464577679392477, 3.808795504615560379, 47.04930799450051637 ) ) ;
#15545=EDGE_LOOP ( 'NONE', ( #9380, #12514, #14706, #23313 ) ) ;
#15549=VERTEX_POINT ( 'NONE', #26748 ) ;
#15550=VERTEX_POINT ( 'NONE', #19349 ) ;
#15569=EDGE_LOOP ( 'NONE', ( #18185, #13390, #31367, #32172 ) ) ;
#15570=FACE_OUTER_BOUND ( 'NONE', #17794, .T. ) ;
#15571=CARTESIAN_POINT ( 'NONE',  ( -41.63422246745999189, 11.51531537899137447, 57.04930799450051637 ) ) ;
#15577=AXIS2_PLACEMENT_3D ( 'NONE', #25675, #31094, #18915 ) ;
#15587=EDGE_CURVE ( 'NONE', #1567, #9952, #31592, .T. ) ;
#15589=ORIENTED_EDGE ( 'NONE', *, *, #26204, .F. ) ;
#15594=CARTESIAN_POINT ( 'NONE',  ( -40.57832940339291383, 7.446916344587776848, 60.54930799450051637 ) ) ;
#15595=VECTOR ( 'NONE', #24420, 1000.000000000000114 ) ;
#15611=CARTESIAN_POINT ( 'NONE',  ( -41.10400476907452116, 9.333823787025618657, 34.66646528202590360 ) ) ;
#15614=DIRECTION ( 'NONE',  ( -0.9612616959383194493, -0.2756373558169974980, -8.795445018804946186E-19 ) ) ;
#15619=FACE_OUTER_BOUND ( 'NONE', #25504, .T. ) ;
#15622=ORIENTED_EDGE ( 'NONE', *, *, #10686, .T. ) ;
#15629=CARTESIAN_POINT ( 'NONE',  ( -43.90780810587784089, -0.03953120679776617880, 61.94930799450052206 ) ) ;
#15632=EDGE_CURVE ( 'NONE', #17901, #7171, #9591, .T. ) ;
#15637=DIRECTION ( 'NONE',  ( 0.000000000000000000, 0.000000000000000000, 1.000000000000000000 ) ) ;
#15643=VECTOR ( 'NONE', #16891, 1000.000000000000114 ) ;
#15646=LINE ( 'NONE', #20734, #10260 ) ;
#15649=DIRECTION ( 'NONE',  ( 0.2756373558169973870, -0.9612616959383193382, -1.315048337272770280E-17 ) ) ;
#15651=CARTESIAN_POINT ( 'NONE',  ( -40.69549116917064424, 6.786800228906571419, 39.45362111768539393 ) ) ;
#15652=ORIENTED_EDGE ( 'NONE', *, *, #9627, .F. ) ;
#15653=CARTESIAN_POINT ( 'NONE',  ( -42.11634311166133671, 14.67824478428857660, 37.04930799450052348 ) ) ;
#15657=VECTOR ( 'NONE', #30411, 1000.000000000000227 ) ;
#15658=CARTESIAN_POINT ( 'NONE',  ( -40.62017490690358557, 6.854514378931026997, 39.32186498431286026 ) ) ;
#15668=EDGE_CURVE ( 'NONE', #14556, #9452, #15878, .T. ) ;
#15678=VECTOR ( 'NONE', #12661, 1000.000000000000114 ) ;
#15680=DIRECTION ( 'NONE',  ( -2.779292025043186357E-18, 1.288349127009862057E-17, -1.000000000000000000 ) ) ;
#15681=FACE_OUTER_BOUND ( 'NONE', #9219, .T. ) ;
#15690=ORIENTED_EDGE ( 'NONE', *, *, #24466, .F. ) ;
#15692=EDGE_LOOP ( 'NONE', ( #21541, #24629, #2781, #1978 ) ) ;
#15693=DIRECTION ( 'NONE',  ( -0.9862637841664554372, -0.1651779284337450415, 0.000000000000000000 ) ) ;
#15694=CARTESIAN_POINT ( 'NONE',  ( -40.68535844407768565, 8.206233278606879011, 59.57859731638185963 ) ) ;
#15703=CARTESIAN_POINT ( 'NONE',  ( -42.38687957179149635, 4.148162238788000167, 35.84930799450052064 ) ) ;
#15706=ORIENTED_EDGE ( 'NONE', *, *, #15843, .T. ) ;
#15707=DIRECTION ( 'NONE',  ( 0.000000000000000000, 0.000000000000000000, -1.000000000000000000 ) ) ;
#15708=ORIENTED_EDGE ( 'NONE', *, *, #15165, .T. ) ;
#15709=AXIS2_PLACEMENT_3D ( 'NONE', #16100, #7933, #18404 ) ;
#15712=ORIENTED_EDGE ( 'NONE', *, *, #6801, .F. ) ;
#15714=EDGE_LOOP ( 'NONE', ( #32065, #12108, #23663, #7656 ) ) ;
#15717=ORIENTED_EDGE ( 'NONE', *, *, #18845, .T. ) ;
#15723=LINE ( 'NONE', #3247, #15983 ) ;
#15728=VECTOR ( 'NONE', #5641, 1000.000000000000114 ) ;
#15729=CARTESIAN_POINT ( 'NONE',  ( -40.21210701746133509, 7.644196001419694575, 60.44930799450051495 ) ) ;
#15730=CARTESIAN_POINT ( 'NONE',  ( -40.05313298863235616, 9.531126477505384997, 39.44930799450052206 ) ) ;
#15733=VECTOR ( 'NONE', #23342, 1000.000000000000114 ) ;
#15737=DIRECTION ( 'NONE',  ( 0.4848096202463365034, 0.8746197071393960742, -2.220446049250311602E-16 ) ) ;
#15742=DIRECTION ( 'NONE',  ( 0.8746197071393858602, -0.4848096202463547666, 0.000000000000000000 ) ) ;
#15744=ORIENTED_EDGE ( 'NONE', *, *, #2034, .T. ) ;
#15755=ADVANCED_FACE ( 'NONE', ( #3082 ), #948, .T. ) ;
#15757=ADVANCED_FACE ( 'NONE', ( #28533 ), #6049, .T. ) ;
#15761=AXIS2_PLACEMENT_3D ( 'NONE', #1087, #18479, #28507 ) ;
#15764=ORIENTED_EDGE ( 'NONE', *, *, #28316, .T. ) ;
#15766=DIRECTION ( 'NONE',  ( 0.4848096202463430537, 0.8746197071393926326, 1.323854077651070671E-16 ) ) ;
#15773=CARTESIAN_POINT ( 'NONE',  ( -40.98031486389898248, 9.265261353013489298, 39.44930799450052206 ) ) ;
#15778=CARTESIAN_POINT ( 'NONE',  ( -42.41019933908752648, 14.71530103803245915, 55.14139656020049785 ) ) ;
#15780=DIRECTION ( 'NONE',  ( -0.9612616959383200044, -0.2756373558169954996, 1.660411357259285896E-16 ) ) ;
#15784=VERTEX_POINT ( 'NONE', #8037 ) ;
#15787=FACE_OUTER_BOUND ( 'NONE', #16774, .T. ) ;
#15788=AXIS2_PLACEMENT_3D ( 'NONE', #23045, #2866, #25359 ) ;
#15789=DIRECTION ( 'NONE',  ( 0.000000000000000000, 0.000000000000000000, -1.000000000000000000 ) ) ;
#15792=( BOUNDED_CURVE ( )  B_SPLINE_CURVE ( 3, ( #841, #6414, #10866, #18393 ),
 .UNSPECIFIED., .F., .F. ) 
 B_SPLINE_CURVE_WITH_KNOTS ( ( 4, 4 ),
 ( 4.712388980384698556, 5.497787143782109531 ),
 .UNSPECIFIED. ) 
 CURVE ( )  GEOMETRIC_REPRESENTATION_ITEM ( )  RATIONAL_B_SPLINE_CURVE ( ( 1.000000000000000000, 0.9492530216741960070, 0.9492530216741960070, 1.000000000000000000 ) ) 
 REPRESENTATION_ITEM ( '' )  );
#15794=CARTESIAN_POINT ( 'NONE',  ( -40.02353495526242710, 6.996741961792354303, 39.54930799450052348 ) ) ;
#15796=PLANE ( 'NONE',  #9985 ) ;
#15807=CARTESIAN_POINT ( 'NONE',  ( -42.41019933908752648, 14.71530103803245915, 60.54930799450051637 ) ) ;
#15811=LINE ( 'NONE', #10890, #24329 ) ;
#15815=ORIENTED_EDGE ( 'NONE', *, *, #13461, .F. ) ;
#15816=CARTESIAN_POINT ( 'NONE',  ( -42.47434154250544225, 4.196643200812637531, 57.04930799450051637 ) ) ;
#15819=FACE_OUTER_BOUND ( 'NONE', #3324, .T. ) ;
#15823=DIRECTION ( 'NONE',  ( -7.588956326749211550E-18, 4.206627182996911684E-18, -1.000000000000000000 ) ) ;
#15827=AXIS2_PLACEMENT_3D ( 'NONE', #25111, #22805, #10508 ) ;
#15828=CARTESIAN_POINT ( 'NONE',  ( -40.54018958231235814, 7.005332542891154368, 39.07553933734813967 ) ) ;
#15829=CIRCLE ( 'NONE', #14266, 2.000000000000001776 ) ;
#15831=CIRCLE ( 'NONE', #14781, 0.09999999999999753530 ) ;
#15840=ORIENTED_EDGE ( 'NONE', *, *, #2358, .T. ) ;
#15841=CARTESIAN_POINT ( 'NONE',  ( -40.62282199596570109, 7.625347238340324907, 60.15421819779515289 ) ) ;
#15842=ORIENTED_EDGE ( 'NONE', *, *, #15866, .F. ) ;
#15843=EDGE_CURVE ( 'NONE', #21286, #6401, #24353, .T. ) ;
#15845=ORIENTED_EDGE ( 'NONE', *, *, #4117, .T. ) ;
#15846=VECTOR ( 'NONE', #10784, 1000.000000000000000 ) ;
#15848=AXIS2_PLACEMENT_3D ( 'NONE', #2758, #9988, #2914 ) ;
#15850=DIRECTION ( 'NONE',  ( 0.4848096202463427762, 0.8746197071393926326, 0.000000000000000000 ) ) ;
#15861=ORIENTED_EDGE ( 'NONE', *, *, #1422, .T. ) ;
#15865=CARTESIAN_POINT ( 'NONE',  ( -40.99173213700658636, 9.305078116158226109, 34.54930799450052348 ) ) ;
#15866=EDGE_CURVE ( 'NONE', #23684, #31307, #25336, .T. ) ;
#15868=DIRECTION ( 'NONE',  ( 0.8746197071393926326, -0.4848096202463430537, -8.676864087101709653E-18 ) ) ;
#15878=CIRCLE ( 'NONE', #1710, 0.9999999999999998890 ) ;
#15890=EDGE_CURVE ( 'NONE', #1774, #16834, #8816, .T. ) ;
#15901=ORIENTED_EDGE ( 'NONE', *, *, #1617, .T. ) ;
#15903=ADVANCED_FACE ( 'NONE', ( #26543 ), #1213, .T. ) ;
#15908=EDGE_LOOP ( 'NONE', ( #376, #18847, #31658, #907 ) ) ;
#15910=DIRECTION ( 'NONE',  ( -0.7141240004913248507, 0.3958453973319954744, 0.5773502691896323924 ) ) ;
#15915=DIRECTION ( 'NONE',  ( 0.9612616959383221138, 0.2756373558169876170, 0.000000000000000000 ) ) ;
#15923=DIRECTION ( 'NONE',  ( 0.9612616959383207815, 0.2756373558169927240, 8.795445018804291370E-19 ) ) ;
#15933=CARTESIAN_POINT ( 'NONE',  ( -42.25266656316760105, 14.76047283463325321, 59.54930799450050927 ) ) ;
#15939=CARTESIAN_POINT ( 'NONE',  ( -40.65740519188835123, 6.815948303523045482, 34.58882370767772585 ) ) ;
#15940=( NAMED_UNIT ( * ) SI_UNIT ( $, .STERADIAN. ) SOLID_ANGLE_UNIT ( ) );
#15941=ORIENTED_EDGE ( 'NONE', *, *, #2586, .F. ) ;
#15946=ORIENTED_EDGE ( 'NONE', *, *, #10129, .T. ) ;
#15953=TOROIDAL_SURFACE ( 'NONE', #25912, 1.899999999999999467, 0.1000000000000000056 ) ;
#15957=FACE_OUTER_BOUND ( 'NONE', #23808, .T. ) ;
#15960=ORIENTED_EDGE ( 'NONE', *, *, #8451, .F. ) ;
#15961=CARTESIAN_POINT ( 'NONE',  ( -40.74365851677129768, 8.439942589813741236, 39.54930799450052348 ) ) ;
#15965=CARTESIAN_POINT ( 'NONE',  ( -41.96544240928614755, 13.75880317176705603, 54.54930799450051637 ) ) ;
#15966=EDGE_CURVE ( 'NONE', #9355, #25738, #20080, .T. ) ;
#15967=CARTESIAN_POINT ( 'NONE',  ( -48.25869185997735400, 10.94158050198885590, 59.53596428539564300 ) ) ;
#15973=DIRECTION ( 'NONE',  ( -0.8746197071393925215, 0.4848096202463429982, 8.676864087101709653E-18 ) ) ;
#15975=EDGE_CURVE ( 'NONE', #13582, #22782, #23229, .T. ) ;
#15979=CIRCLE ( 'NONE', #3398, 0.7928932188134565351 ) ;
#15983=VECTOR ( 'NONE', #10816, 1000.000000000000000 ) ;
#15986=DIRECTION ( 'NONE',  ( 0.000000000000000000, 0.000000000000000000, -1.000000000000000000 ) ) ;
#15989=DIRECTION ( 'NONE',  ( -0.7141240004912712269, 0.3958453973320736341, 0.5773502691896451600 ) ) ;
#15990=CARTESIAN_POINT ( 'NONE',  ( -40.18454328187963398, 7.548069831825862330, 53.64930799450051779 ) ) ;
#15993=EDGE_LOOP ( 'NONE', ( #25983, #2955, #27596, #9466 ) ) ;
#15996=EDGE_LOOP ( 'NONE', ( #19124, #9127 ) ) ;
#15999=EDGE_CURVE ( 'NONE', #27032, #2499, #2414, .T. ) ;
#16001=ADVANCED_FACE ( 'NONE', ( #4710 ), #1913, .F. ) ;
#16007=ORIENTED_EDGE ( 'NONE', *, *, #24800, .F. ) ;
#16009=ORIENTED_EDGE ( 'NONE', *, *, #21183, .T. ) ;
#16021=DIRECTION ( 'NONE',  ( -0.8746197071393926326, 0.4848096202463430537, 8.676864087101709653E-18 ) ) ;
#16027=CARTESIAN_POINT ( 'NONE',  ( -40.61337426079494151, 6.957937756950597574, 35.07960045310107233 ) ) ;
#16030=AXIS2_PLACEMENT_3D ( 'NONE', #3173, #28772, #20582 ) ;
#16032=EDGE_LOOP ( 'NONE', ( #20526, #28107, #19180, #22738, #3898 ) ) ;
#16036=EDGE_CURVE ( 'NONE', #26371, #22928, #5937, .T. ) ;
#16037=TOROIDAL_SURFACE ( 'NONE', #28089, 0.2000000000000000111, 0.1000000000000000056 ) ;
#16041=EDGE_CURVE ( 'NONE', #19917, #8660, #4363, .T. ) ;
#16042=ORIENTED_EDGE ( 'NONE', *, *, #26386, .T. ) ;
#16044=CIRCLE ( 'NONE', #19700, 0.1000000000000018235 ) ;
#16046=ORIENTED_EDGE ( 'NONE', *, *, #31584, .T. ) ;
#16057=CARTESIAN_POINT ( 'NONE',  ( -40.69332644341266558, 6.790879890547247832, 39.41319887685486378 ) ) ;
#16062=CARTESIAN_POINT ( 'NONE',  ( -40.02540636251514172, 2.839176264122877047, 55.74930799450051211 ) ) ;
#16063=CARTESIAN_POINT ( 'NONE',  ( -40.15599670534037102, 7.478908884098772525, 34.64930799450051779 ) ) ;
#16068=VERTEX_POINT ( 'NONE', #7336 ) ;
#16072=EDGE_CURVE ( 'NONE', #4922, #9470, #23245, .T. ) ;
#16088=ORIENTED_EDGE ( 'NONE', *, *, #21689, .T. ) ;
#16096=CARTESIAN_POINT ( 'NONE',  ( -42.76364231915344050, 15.12166775071173852, 38.44930799450052206 ) ) ;
#16100=CARTESIAN_POINT ( 'NONE',  ( -40.11286833322907341, 2.887657226147507306, 37.04930799450052348 ) ) ;
#16110=EDGE_CURVE ( 'NONE', #19824, #8349, #30793, .T. ) ;
#16113=VECTOR ( 'NONE', #17636, 1000.000000000000000 ) ;
#16115=CARTESIAN_POINT ( 'NONE',  ( -40.50146157965988891, 7.595301493077382560, 38.66054537865625917 ) ) ;
#16117=AXIS2_PLACEMENT_3D ( 'NONE', #13244, #10928, #23873 ) ;
#16121=DIRECTION ( 'NONE',  ( 0.4848096202463673676, 0.8746197071393789768, 0.000000000000000000 ) ) ;
#16124=LINE ( 'NONE', #15967, #15224 ) ;
#16138=DIRECTION ( 'NONE',  ( 0.4848096202463424986, 0.8746197071393928546, -2.220446049250312834E-16 ) ) ;
#16151=ADVANCED_FACE ( 'NONE', ( #25863 ), #14651, .T. ) ;
#16155=AXIS2_PLACEMENT_3D ( 'NONE', #4281, #16577, #19529 ) ;
#16158=B_SPLINE_CURVE_WITH_KNOTS ( 'NONE', 3,
 ( #24441, #1310, #26581, #11332, #13963, #9027, #9193, #31358 ),
 .UNSPECIFIED., .F., .F.,
 ( 4, 2, 2, 4 ),
 ( 0.000000000000000000, 0.0005384193795069787359, 0.0008076290692604753138, 0.001076838759013972000 ),
 .UNSPECIFIED. ) ;
#16161=DIRECTION ( 'NONE',  ( 0.9612616959383221138, 0.2756373558169876170, 0.000000000000000000 ) ) ;
#16163=CYLINDRICAL_SURFACE ( 'NONE', #6184, 0.1000000000000008243 ) ;
#16168=DIRECTION ( 'NONE',  ( -2.779292025043186357E-18, 1.288349127009862211E-17, -1.000000000000000000 ) ) ;
#16170=FACE_OUTER_BOUND ( 'NONE', #29956, .T. ) ;
#16171=CARTESIAN_POINT ( 'NONE',  ( -40.28779227465695811, 2.984619150196779369, 55.04930799450051637 ) ) ;
#16172=DIRECTION ( 'NONE',  ( -0.4848096202463429427, -0.8746197071393925215, 2.352477780477436787E-16 ) ) ;
#16187=PLANE ( 'NONE',  #23205 ) ;
#16190=ORIENTED_EDGE ( 'NONE', *, *, #25532, .F. ) ;
#16192=ORIENTED_EDGE ( 'NONE', *, *, #6933, .T. ) ;
#16195=CYLINDRICAL_SURFACE ( 'NONE', #12315, 0.09999999999999945044 ) ;
#16204=EDGE_LOOP ( 'NONE', ( #7733, #4685 ) ) ;
#16206=DIRECTION ( 'NONE',  ( 0.8746197071393925215, -0.4848096202463429982, -8.676864087101708112E-18 ) ) ;
#16210=VECTOR ( 'NONE', #10764, 1000.000000000000114 ) ;
#16211=CARTESIAN_POINT ( 'NONE',  ( -40.70323106273436053, 6.774493230553227718, 39.52357759537398607 ) ) ;
#16222=EDGE_CURVE ( 'NONE', #27140, #31848, #27440, .T. ) ;
#16224=DIRECTION ( 'NONE',  ( -1.188208965918165239E-16, -1.880121038077813132E-16, -1.000000000000000000 ) ) ;
#16225=ORIENTED_EDGE ( 'NONE', *, *, #3298, .F. ) ;
#16228=CARTESIAN_POINT ( 'NONE',  ( -40.73091736380679606, 9.483895492497156354, 35.44930799450052206 ) ) ;
#16230=AXIS2_PLACEMENT_3D ( 'NONE', #12210, #16947, #9905 ) ;
#16232=EDGE_CURVE ( 'NONE', #17298, #4462, #29091, .T. ) ;
#16233=AXIS2_PLACEMENT_3D ( 'NONE', #9248, #26807, #31579 ) ;
#16237=AXIS2_PLACEMENT_3D ( 'NONE', #21293, #14254, #24249 ) ;
#16238=CARTESIAN_POINT ( 'NONE',  ( -41.13825658839732569, 9.453274076459845077, 38.50788663826321567 ) ) ;
#16240=CYLINDRICAL_SURFACE ( 'NONE', #19681, 0.1000000000000020595 ) ;
#16242=ORIENTED_EDGE ( 'NONE', *, *, #9066, .T. ) ;
#16244=DIRECTION ( 'NONE',  ( -0.8746197071393926326, 0.4848096202463430537, 8.676864087101709653E-18 ) ) ;
#16246=ORIENTED_EDGE ( 'NONE', *, *, #15431, .F. ) ;
#16248=ORIENTED_EDGE ( 'NONE', *, *, #13354, .F. ) ;
#16252=DIRECTION ( 'NONE',  ( 0.9612616959383194493, 0.2756373558169974980, 8.795445018804946186E-19 ) ) ;
#16253=VERTEX_POINT ( 'NONE', #19394 ) ;
#16255=LINE ( 'NONE', #26594, #3977 ) ;
#16266=ORIENTED_EDGE ( 'NONE', *, *, #16890, .F. ) ;
#16267=FACE_OUTER_BOUND ( 'NONE', #31598, .T. ) ;
#16270=VECTOR ( 'NONE', #2356, 1000.000000000000114 ) ;
#16276=DIRECTION ( 'NONE',  ( -2.779292025043186357E-18, 1.288349127009862211E-17, -1.000000000000000000 ) ) ;
#16284=EDGE_CURVE ( 'NONE', #1905, #11711, #21693, .T. ) ;
#16288=VERTEX_POINT ( 'NONE', #17094 ) ;
#16291=CARTESIAN_POINT ( 'NONE',  ( -39.64148344771002286, 7.657122216028890982, 62.04930799450052348 ) ) ;
#16294=DIRECTION ( 'NONE',  ( 0.000000000000000000, 0.000000000000000000, -1.000000000000000000 ) ) ;
#16296=CIRCLE ( 'NONE', #6889, 1.003191532947548925 ) ;
#16299=CARTESIAN_POINT ( 'NONE',  ( -40.12425944110432852, 6.890664497466326033, 34.56792418805707712 ) ) ;
#16301=ORIENTED_EDGE ( 'NONE', *, *, #19208, .T. ) ;
#16302=FACE_OUTER_BOUND ( 'NONE', #1288, .T. ) ;
#16310=ORIENTED_EDGE ( 'NONE', *, *, #31702, .T. ) ;
#16321=DIRECTION ( 'NONE',  ( -0.9612616959383207815, -0.2756373558169927240, 3.618802040241776925E-17 ) ) ;
#16322=VERTEX_POINT ( 'NONE', #27112 ) ;
#16325=CYLINDRICAL_SURFACE ( 'NONE', #17022, 1.199999999999999734 ) ;
#16329=DIRECTION ( 'NONE',  ( -0.4848096202463484938, -0.8746197071393896350, 2.220446049250314067E-16 ) ) ;
#16330=DIRECTION ( 'NONE',  ( -0.8746197071393926326, 0.4848096202463430537, 8.676864087101709653E-18 ) ) ;
#16335=DIRECTION ( 'NONE',  ( 0.4848096202463637039, 0.8746197071393810862, 0.000000000000000000 ) ) ;
#16338=ADVANCED_FACE ( 'NONE', ( #25467 ), #2493, .T. ) ;
#16339=ADVANCED_FACE ( 'NONE', ( #508 ), #26851, .F. ) ;
#16341=ORIENTED_EDGE ( 'NONE', *, *, #28209, .T. ) ;
#16342=CARTESIAN_POINT ( 'NONE',  ( -40.23397449525940317, 6.794506605641760011, 34.54930799450052348 ) ) ;
#16343=CARTESIAN_POINT ( 'NONE',  ( -40.47677217214081224, 7.509199159541737778, 35.32896003352318814 ) ) ;
#16344=ORIENTED_EDGE ( 'NONE', *, *, #22060, .F. ) ;
#16347=AXIS2_PLACEMENT_3D ( 'NONE', #6496, #16021, #26026 ) ;
#16350=ORIENTED_EDGE ( 'NONE', *, *, #15975, .F. ) ;
#16356=ADVANCED_FACE ( 'NONE', ( #17587 ), #15296, .T. ) ;
#16357=VERTEX_POINT ( 'NONE', #20049 ) ;
#16359=AXIS2_PLACEMENT_3D ( 'NONE', #22677, #17745, #7747 ) ;
#16360=CARTESIAN_POINT ( 'NONE',  ( -42.47434154250544225, 4.196643200812637531, 58.94930799450051495 ) ) ;
#16368=ORIENTED_EDGE ( 'NONE', *, *, #22373, .F. ) ;
#16371=DIRECTION ( 'NONE',  ( -0.8746197071393925215, 0.4848096202463429982, 8.676864087101708112E-18 ) ) ;
#16374=ADVANCED_FACE ( 'NONE', ( #5120 ), #6965, .T. ) ;
#16378=LINE ( 'NONE', #18672, #22585 ) ;
#16379=LINE ( 'NONE', #23929, #1742 ) ;
#16381=VERTEX_POINT ( 'NONE', #10214 ) ;
#16386=CARTESIAN_POINT ( 'NONE',  ( -40.66586793973302605, 8.138261812237592707, 59.50788663826320146 ) ) ;
#16387=VERTEX_POINT ( 'NONE', #195 ) ;
#16389=ORIENTED_EDGE ( 'NONE', *, *, #11216, .F. ) ;
#16392=ORIENTED_EDGE ( 'NONE', *, *, #25760, .F. ) ;
#16395=CIRCLE ( 'NONE', #28997, 1.199999999999999734 ) ;
#16398=PLANE ( 'NONE',  #29077 ) ;
#16399=ADVANCED_FACE ( 'NONE', ( #12689 ), #30079, .T. ) ;
#16408=CARTESIAN_POINT ( 'NONE',  ( -43.43257085947613660, 1.024086014757300989, 53.64930799450051779 ) ) ;
#16409=ORIENTED_EDGE ( 'NONE', *, *, #8767, .T. ) ;
#16414=ADVANCED_FACE ( 'NONE', ( #24819 ), #3789, .T. ) ;
#16415=ORIENTED_EDGE ( 'NONE', *, *, #3935, .F. ) ;
#16416=ORIENTED_EDGE ( 'NONE', *, *, #11647, .T. ) ;
#16426=DIRECTION ( 'NONE',  ( 0.4848096202463424431, 0.8746197071393927436, -2.220446049250312588E-16 ) ) ;
#16429=CARTESIAN_POINT ( 'NONE',  ( -40.50726676055796105, 7.559560307024983494, 60.29072935073781991 ) ) ;
#16433=ADVANCED_FACE ( 'NONE', ( #23800 ), #1315, .T. ) ;
#16443=EDGE_CURVE ( 'NONE', #27795, #2831, #30563, .T. ) ;
#16448=DIRECTION ( 'NONE',  ( 0.9612616959383221138, 0.2756373558169876170, 0.000000000000000000 ) ) ;
#16459=CIRCLE ( 'NONE', #24860, 0.1000000000000012962 ) ;
#16460=ORIENTED_EDGE ( 'NONE', *, *, #13434, .T. ) ;
#16462=CARTESIAN_POINT ( 'NONE',  ( -40.22836982583548604, 6.952244300597152815, 39.38126462244056114 ) ) ;
#16465=DIRECTION ( 'NONE',  ( 0.000000000000000000, 0.000000000000000000, -1.000000000000000000 ) ) ;
#16470=DIRECTION ( 'NONE',  ( 0.2530443915476854322, -0.8824706660164470806, 0.3965022818682764627 ) ) ;
#16476=EDGE_CURVE ( 'NONE', #5096, #23253, #26103, .T. ) ;
#16483=AXIS2_PLACEMENT_3D ( 'NONE', #5856, #909, #13723 ) ;
#16485=ADVANCED_FACE ( 'NONE', ( #8712 ), #28255, .T. ) ;
#16487=AXIS2_PLACEMENT_3D ( 'NONE', #10459, #22916, #23251 ) ;
#16495=CARTESIAN_POINT ( 'NONE',  ( -40.73091736380679606, 9.483895492497158131, 39.44930799450052206 ) ) ;
#16497=CARTESIAN_POINT ( 'NONE',  ( -40.57832940339291383, 7.446916344587776848, 53.85980283506936672 ) ) ;
#16498=ORIENTED_EDGE ( 'NONE', *, *, #18518, .F. ) ;
#16500=SPHERICAL_SURFACE ( 'NONE', #17315, 0.1000000000000000056 ) ;
#16503=ORIENTED_EDGE ( 'NONE', *, *, #11132, .F. ) ;
#16504=CARTESIAN_POINT ( 'NONE',  ( -40.00476266209307852, 7.314288625132040700, 35.33031476312594066 ) ) ;
#16517=EDGE_CURVE ( 'NONE', #655, #2291, #8536, .T. ) ;
#16525=VERTEX_POINT ( 'NONE', #10864 ) ;
#16533=CARTESIAN_POINT ( 'NONE',  ( -40.57495275781087685, 7.492308784444112746, 38.76861099430816893 ) ) ;
#16538=ORIENTED_EDGE ( 'NONE', *, *, #30062, .F. ) ;
#16540=DIRECTION ( 'NONE',  ( 1.431146867680865853E-17, 2.558717127065790464E-17, 1.000000000000000000 ) ) ;
#16541=VECTOR ( 'NONE', #2285, 999.9999999999998863 ) ;
#16544=ORIENTED_EDGE ( 'NONE', *, *, #15999, .T. ) ;
#16545=CARTESIAN_POINT ( 'NONE',  ( -40.02540636251514172, 2.839176264122877047, 55.54930799450051637 ) ) ;
#16550=AXIS2_PLACEMENT_3D ( 'NONE', #18706, #23656, #28261 ) ;
#16554=EDGE_LOOP ( 'NONE', ( #3713, #28498, #6502, #9148 ) ) ;
#16559=CYLINDRICAL_SURFACE ( 'NONE', #4742, 0.09999999999999945044 ) ;
#16561=ORIENTED_EDGE ( 'NONE', *, *, #28676, .F. ) ;
#16572=ORIENTED_EDGE ( 'NONE', *, *, #10044, .F. ) ;
#16577=DIRECTION ( 'NONE',  ( -0.4848096202463430537, -0.8746197071393926326, -9.920727850371701658E-18 ) ) ;
#16579=ORIENTED_EDGE ( 'NONE', *, *, #10669, .F. ) ;
#16582=EDGE_LOOP ( 'NONE', ( #20342, #32169, #15744, #15310, #13927, #3359, #8666 ) ) ;
#16587=VECTOR ( 'NONE', #10178, 1000.000000000000000 ) ;
#16589=ORIENTED_EDGE ( 'NONE', *, *, #31702, .F. ) ;
#16594=CARTESIAN_POINT ( 'NONE',  ( -40.55202315603388286, 7.223587105649684759, 35.33283365102737861 ) ) ;
#16596=ORIENTED_EDGE ( 'NONE', *, *, #8807, .T. ) ;
#16597=DIRECTION ( 'NONE',  ( -0.8746197071393926326, 0.4848096202463430537, 8.676864087101709653E-18 ) ) ;
#16598=LINE ( 'NONE', #24318, #31871 ) ;
#16599=DIRECTION ( 'NONE',  ( 0.000000000000000000, -8.673617379884027583E-16, -1.000000000000000000 ) ) ;
#16613=ORIENTED_EDGE ( 'NONE', *, *, #17891, .F. ) ;
#16640=CARTESIAN_POINT ( 'NONE',  ( -42.21195563036361875, 4.051200314738730768, 39.04930799450052348 ) ) ;
#16641=AXIS2_PLACEMENT_3D ( 'NONE', #4068, #1610, #21459 ) ;
#16644=ORIENTED_EDGE ( 'NONE', *, *, #13278, .T. ) ;
#16645=DIRECTION ( 'NONE',  ( -2.779292025043186357E-18, 1.288349127009862211E-17, -1.000000000000000000 ) ) ;
#16646=DIRECTION ( 'NONE',  ( 0.2756373558169932236, -0.9612616959383206705, -2.918609477355926788E-15 ) ) ;
#16648=VERTEX_POINT ( 'NONE', #11492 ) ;
#16651=AXIS2_PLACEMENT_3D ( 'NONE', #19753, #7467, #28287 ) ;
#16652=FACE_OUTER_BOUND ( 'NONE', #18048, .T. ) ;
#16653=CARTESIAN_POINT ( 'NONE',  ( -42.26497471389478733, 14.66834543456874940, 60.54930799450051637 ) ) ;
#16656=DIRECTION ( 'NONE',  ( -0.1949050434465267878, 0.6797146636928675933, 0.7071067811865471286 ) ) ;
#16662=VERTEX_POINT ( 'NONE', #21659 ) ;
#16669=CIRCLE ( 'NONE', #29266, 1.899999999999999023 ) ;
#16671=CARTESIAN_POINT ( 'NONE',  ( -40.09211399732166115, 9.667069410243957606, 38.64930799450052490 ) ) ;
#16676=CARTESIAN_POINT ( 'NONE',  ( -40.50844712113364920, 7.574537053903299899, 53.86130065048124038 ) ) ;
#16677=EDGE_CURVE ( 'NONE', #9196, #18541, #19190, .T. ) ;
#16679=EDGE_LOOP ( 'NONE', ( #13437, #26922, #17775, #11804 ) ) ;
#16691=AXIS2_PLACEMENT_3D ( 'NONE', #11343, #18399, #15789 ) ;
#16698=CARTESIAN_POINT ( 'NONE',  ( -40.60251150970604073, 6.748447833883064462, 60.44930799450051495 ) ) ;
#16706=CARTESIAN_POINT ( 'NONE',  ( -42.34864001897648933, 13.69590355195401266, 54.59258074835306473 ) ) ;
#16710=VECTOR ( 'NONE', #10767, 1000.000000000000114 ) ;
#16712=CARTESIAN_POINT ( 'NONE',  ( -40.50146157965988891, 7.595301493077382560, 38.44930799450052916 ) ) ;
#16718=DIRECTION ( 'NONE',  ( 0.4848096202460961957, 0.8746197071395293010, 0.000000000000000000 ) ) ;
#16723=DIRECTION ( 'NONE',  ( -0.9612616959383194493, -0.2756373558169974980, -8.795445018804946186E-19 ) ) ;
#16727=ORIENTED_EDGE ( 'NONE', *, *, #24638, .F. ) ;
#16734=EDGE_CURVE ( 'NONE', #5667, #17822, #27868, .T. ) ;
#16735=LINE ( 'NONE', #29225, #30872 ) ;
#16736=ADVANCED_FACE ( 'NONE', ( #20013 ), #10337, .T. ) ;
#16738=ORIENTED_EDGE ( 'NONE', *, *, #28985, .F. ) ;
#16742=EDGE_LOOP ( 'NONE', ( #14482, #10955, #31127 ) ) ;
#16746=CIRCLE ( 'NONE', #16233, 0.09999999999999864553 ) ;
#16754=DIRECTION ( 'NONE',  ( -0.8746197071393926326, 0.4848096202463430537, 8.676864087101709653E-18 ) ) ;
#16755=CARTESIAN_POINT ( 'NONE',  ( -40.54770213959441350, 7.393765961829920741, 35.41885462099428139 ) ) ;
#16758=CIRCLE ( 'NONE', #1557, 0.09999999999999753530 ) ;
#16760=CARTESIAN_POINT ( 'NONE',  ( -41.94956971822180947, 3.905757428664828890, 45.74930799450051211 ) ) ;
#16761=CARTESIAN_POINT ( 'NONE',  ( -43.37834615508418068, 1.121909970995876416, 34.64930799450052490 ) ) ;
#16762=EDGE_CURVE ( 'NONE', #1546, #2789, #7880, .T. ) ;
#16763=DIRECTION ( 'NONE',  ( 0.4848096202463425541, 0.8746197071393929656, -2.220446049250313081E-16 ) ) ;
#16764=VECTOR ( 'NONE', #29674, 1000.000000000000000 ) ;
#16766=DIRECTION ( 'NONE',  ( 0.000000000000000000, 0.000000000000000000, -1.000000000000000000 ) ) ;
#16767=CARTESIAN_POINT ( 'NONE',  ( -40.75848109938849717, 9.580021662090986823, 35.54930799450051637 ) ) ;
#16770=CIRCLE ( 'NONE', #14687, 2.000000000000001776 ) ;
#16774=EDGE_LOOP ( 'NONE', ( #29357, #13248, #12285, #22370, #6088 ) ) ;
#16777=CARTESIAN_POINT ( 'NONE',  ( -40.45528000798979917, 8.522633796558835684, 34.54930799450052348 ) ) ;
#16778=DIRECTION ( 'NONE',  ( 0.2756373558170013283, -0.9612616959383183390, 0.000000000000000000 ) ) ;
#16783=LINE ( 'NONE', #21705, #17655 ) ;
#16786=VERTEX_POINT ( 'NONE', #29879 ) ;
#16787=ORIENTED_EDGE ( 'NONE', *, *, #20700, .F. ) ;
#16788=CARTESIAN_POINT ( 'NONE',  ( -40.13135354151336998, 6.899777549362542395, 39.53627064559790938 ) ) ;
#16790=AXIS2_PLACEMENT_3D ( 'NONE', #12691, #197, #29424 ) ;
#16796=CIRCLE ( 'NONE', #1085, 1.500000000000001332 ) ;
#16797=VERTEX_POINT ( 'NONE', #158 ) ;
#16800=LINE ( 'NONE', #26821, #17358 ) ;
#16801=CIRCLE ( 'NONE', #14716, 0.09999999999999795164 ) ;
#16811=ORIENTED_EDGE ( 'NONE', *, *, #17817, .F. ) ;
#16818=DIRECTION ( 'NONE',  ( -0.4848096202463636484, -0.8746197071393810862, 0.000000000000000000 ) ) ;
#16822=VERTEX_POINT ( 'NONE', #25432 ) ;
#16823=AXIS2_PLACEMENT_3D ( 'NONE', #2265, #10147, #12781 ) ;
#16824=CARTESIAN_POINT ( 'NONE',  ( -40.23847960489091236, 6.935107575317839057, 34.54930799450050927 ) ) ;
#16833=( BOUNDED_CURVE ( )  B_SPLINE_CURVE ( 3, ( #30213, #12666, #27424, #4939 ),
 .UNSPECIFIED., .F., .F. ) 
 B_SPLINE_CURVE_WITH_KNOTS ( ( 4, 4 ),
 ( 3.141592653589793116, 3.493814887450676032 ),
 .UNSPECIFIED. ) 
 CURVE ( )  GEOMETRIC_REPRESENTATION_ITEM ( )  RATIONAL_B_SPLINE_CURVE ( ( 1.000000000000000000, 0.9896883177220923145, 0.9896883177220923145, 1.000000000000000000 ) ) 
 REPRESENTATION_ITEM ( '' )  );
#16834=VERTEX_POINT ( 'NONE', #5573 ) ;
#16841=DIRECTION ( 'NONE',  ( 0.2756373558169931126, -0.9612616959383206705, 1.479773560108267642E-16 ) ) ;
#16842=EDGE_CURVE ( 'NONE', #1328, #15339, #8202, .T. ) ;
#16846=DIRECTION ( 'NONE',  ( 0.000000000000000000, 1.000000000000000000, 0.000000000000000000 ) ) ;
#16847=EDGE_CURVE ( 'NONE', #21737, #14877, #25753, .T. ) ;
#16850=CARTESIAN_POINT ( 'NONE',  ( -40.51045226066063520, 7.589116544599140646, 53.87859731638185679 ) ) ;
#16856=AXIS2_PLACEMENT_3D ( 'NONE', #13415, #18152, #5693 ) ;
#16865=DIRECTION ( 'NONE',  ( 1.188208965918164993E-16, 1.880121038077812639E-16, 1.000000000000000000 ) ) ;
#16866=EDGE_LOOP ( 'NONE', ( #28712, #18996, #26244, #9275 ) ) ;
#16868=CARTESIAN_POINT ( 'NONE',  ( -42.03703168893574116, 3.954238390689463145, 47.04930799450051637 ) ) ;
#16869=CARTESIAN_POINT ( 'NONE',  ( -40.52510752649232728, 7.677764709599122384, 34.54930799450052348 ) ) ;
#16870=AXIS2_PLACEMENT_3D ( 'NONE', #25275, #479, #30693 ) ;
#16871=DIRECTION ( 'NONE',  ( 0.8746197071393926326, -0.4848096202463430537, -8.676864087101709653E-18 ) ) ;
#16875=ORIENTED_EDGE ( 'NONE', *, *, #15495, .F. ) ;
#16877=DIRECTION ( 'NONE',  ( 7.588956326749211550E-18, -4.206627182996912454E-18, 1.000000000000000000 ) ) ;
#16878=ORIENTED_EDGE ( 'NONE', *, *, #28439, .F. ) ;
#16887=EDGE_CURVE ( 'NONE', #28351, #13209, #23224, .T. ) ;
#16889=ORIENTED_EDGE ( 'NONE', *, *, #22403, .F. ) ;
#16890=EDGE_CURVE ( 'NONE', #9599, #6626, #5734, .T. ) ;
#16891=DIRECTION ( 'NONE',  ( 0.9612616959383205595, 0.2756373558169930016, -1.660411357259282199E-16 ) ) ;
#16898=ORIENTED_EDGE ( 'NONE', *, *, #21668, .T. ) ;
#16899=CARTESIAN_POINT ( 'NONE',  ( -40.51565501380215295, 9.065589196111961456, 57.04930799450051637 ) ) ;
#16907=CARTESIAN_POINT ( 'NONE',  ( -42.37913764077812573, 15.23192269303852875, 35.64930799450052490 ) ) ;
#16910=CARTESIAN_POINT ( 'NONE',  ( -40.60333149162104860, 7.557375771971046596, 54.01510846932454513 ) ) ;
#16911=CIRCLE ( 'NONE', #4862, 0.1000000000000018235 ) ;
#16914=CARTESIAN_POINT ( 'NONE',  ( -40.65487266620045403, 9.475231293617264683, 39.43717596014455040 ) ) ;
#16916=CIRCLE ( 'NONE', #6432, 0.09999999999999795164 ) ;
#16930=CYLINDRICAL_SURFACE ( 'NONE', #23363, 2.000000000000001776 ) ;
#16932=DIRECTION ( 'NONE',  ( 2.779292025043186357E-18, -1.288349127009862211E-17, 1.000000000000000000 ) ) ;
#16936=ORIENTED_EDGE ( 'NONE', *, *, #22431, .T. ) ;
#16940=DIRECTION ( 'NONE',  ( 0.2756373558169942228, -0.9612616959383203374, 0.000000000000000000 ) ) ;
#16947=DIRECTION ( 'NONE',  ( 0.8746197071393926326, -0.4848096202463430537, -8.676864087101709653E-18 ) ) ;
#16948=CARTESIAN_POINT ( 'NONE',  ( -40.02540636251513462, 2.839176264122873050, 38.24930799450051921 ) ) ;
#16957=DIRECTION ( 'NONE',  ( 0.2756373558169974980, -0.9612616959383194493, -1.315048337272770743E-17 ) ) ;
#16964=FACE_OUTER_BOUND ( 'NONE', #20553, .T. ) ;
#16965=EDGE_CURVE ( 'NONE', #5962, #16253, #3411, .T. ) ;
#16970=CIRCLE ( 'NONE', #16237, 1.042135311067126979 ) ;
#16989=ADVANCED_FACE ( 'NONE', ( #11945 ), #9155, .T. ) ;
#16990=ORIENTED_EDGE ( 'NONE', *, *, #10772, .T. ) ;
#17002=DIRECTION ( 'NONE',  ( -0.4848096202463429982, -0.8746197071393925215, -9.920727850371698576E-18 ) ) ;
#17007=LINE ( 'NONE', #27033, #9168 ) ;
#17011=DIRECTION ( 'NONE',  ( 0.2756373558169932236, -0.9612616959383204485, 1.479773560108267395E-16 ) ) ;
#17012=DIRECTION ( 'NONE',  ( 0.4848096202463673121, 0.8746197071393789768, 0.000000000000000000 ) ) ;
#17020=CARTESIAN_POINT ( 'NONE',  ( -40.21210701746132798, 7.644196001419686581, 53.84930799450049932 ) ) ;
#17022=AXIS2_PLACEMENT_3D ( 'NONE', #26343, #13882, #23880 ) ;
#17026=AXIS2_PLACEMENT_3D ( 'NONE', #23406, #915, #28815 ) ;
#17027=FACE_OUTER_BOUND ( 'NONE', #25538, .T. ) ;
#17030=AXIS2_PLACEMENT_3D ( 'NONE', #16712, #4572, #12140 ) ;
#17032=CARTESIAN_POINT ( 'NONE',  ( -36.76418579970419387, 10.14130568307076352, 56.14611646155296398 ) ) ;
#17034=VERTEX_POINT ( 'NONE', #23926 ) ;
#17039=ORIENTED_EDGE ( 'NONE', *, *, #29081, .F. ) ;
#17041=VECTOR ( 'NONE', #32330, 1000.000000000000000 ) ;
#17042=ORIENTED_EDGE ( 'NONE', *, *, #23838, .T. ) ;
#17043=VECTOR ( 'NONE', #27409, 1000.000000000000000 ) ;
#17045=EDGE_CURVE ( 'NONE', #30194, #607, #26355, .T. ) ;
#17048=CYLINDRICAL_SURFACE ( 'NONE', #8789, 0.1000000000000028644 ) ;
#17051=DIRECTION ( 'NONE',  ( 0.2756373558169958327, -0.9612616959383198934, 0.000000000000000000 ) ) ;
#17058=AXIS2_PLACEMENT_3D ( 'NONE', #23789, #6718, #31673 ) ;
#17064=EDGE_LOOP ( 'NONE', ( #17578, #11413, #31029, #8381, #12752, #8500 ) ) ;
#17067=CARTESIAN_POINT ( 'NONE',  ( -40.23397449525940317, 6.794506605641760899, 39.54930799450052348 ) ) ;
#17070=EDGE_LOOP ( 'NONE', ( #8408, #8611, #480, #1970 ) ) ;
#17074=DIRECTION ( 'NONE',  ( -0.2756373558169974980, 0.9612616959383193382, 1.315048337272770589E-17 ) ) ;
#17075=CARTESIAN_POINT ( 'NONE',  ( -40.32034427004700916, 8.384459687302960873, 59.44930799450051495 ) ) ;
#17080=ADVANCED_FACE ( 'NONE', ( #10307 ), #7349, .F. ) ;
#17082=ORIENTED_EDGE ( 'NONE', *, *, #21360, .T. ) ;
#17084=DIRECTION ( 'NONE',  ( -0.9612616959383193382, -0.2756373558169974980, -8.795445018804950038E-19 ) ) ;
#17087=ORIENTED_EDGE ( 'NONE', *, *, #19481, .T. ) ;
#17088=DIRECTION ( 'NONE',  ( 0.000000000000000000, 0.000000000000000000, -1.000000000000000000 ) ) ;
#17094=CARTESIAN_POINT ( 'NONE',  ( -40.11729073372970333, 6.802967823440400963, 39.44930799450052206 ) ) ;
#17105=VERTEX_POINT ( 'NONE', #2582 ) ;
#17115=DIRECTION ( 'NONE',  ( -0.1949050434465251780, 0.6797146636928671493, -0.7071067811865480168 ) ) ;
#17124=ORIENTED_EDGE ( 'NONE', *, *, #17668, .F. ) ;
#17128=CARTESIAN_POINT ( 'NONE',  ( -40.15599670534037102, 7.478908884098772525, 35.90717268343339441 ) ) ;
#17129=ORIENTED_EDGE ( 'NONE', *, *, #19523, .F. ) ;
#17134=CARTESIAN_POINT ( 'NONE',  ( -40.02540636251513462, 2.839176264122873050, 35.54930799450051637 ) ) ;
#17140=CARTESIAN_POINT ( 'NONE',  ( -40.18454328187963398, 7.548069831825862330, 60.44930799450051495 ) ) ;
#17141=VERTEX_POINT ( 'NONE', #7518 ) ;
#17150=ORIENTED_EDGE ( 'NONE', *, *, #21063, .F. ) ;
#17155=ORIENTED_EDGE ( 'NONE', *, *, #6591, .T. ) ;
#17164=DIRECTION ( 'NONE',  ( 0.4848096202463430537, 0.8746197071393926326, -1.125439520643636483E-16 ) ) ;
#17166=DIRECTION ( 'NONE',  ( 0.000000000000000000, -1.668003342285388297E-15, -1.000000000000000000 ) ) ;
#17170=DIRECTION ( 'NONE',  ( -0.8746197071393925215, 0.4848096202463429982, 8.676864087101708112E-18 ) ) ;
#17178=CARTESIAN_POINT ( 'NONE',  ( -43.72819403793993587, 1.315833819094413659, 34.64930799450052490 ) ) ;
#17182=DIRECTION ( 'NONE',  ( -0.1138751963119829791, 0.8685717160922530322, -0.4823024089401439785 ) ) ;
#17194=DIRECTION ( 'NONE',  ( 0.4848096202463673121, 0.8746197071393789768, 0.000000000000000000 ) ) ;
#17195=EDGE_CURVE ( 'NONE', #2754, #14753, #25357, .T. ) ;
#17196=CIRCLE ( 'NONE', #11963, 2.000000000000001776 ) ;
#17197=EDGE_LOOP ( 'NONE', ( #11630, #367, #3269, #19310 ) ) ;
#17206=AXIS2_PLACEMENT_3D ( 'NONE', #21666, #31537, #2143 ) ;
#17210=CARTESIAN_POINT ( 'NONE',  ( -41.52623485060432529, 12.58989991563029953, 57.04930799450051637 ) ) ;
#17220=LINE ( 'NONE', #22465, #16587 ) ;
#17222=CARTESIAN_POINT ( 'NONE',  ( -40.69114442294517175, 6.794816359673570894, 34.71217099316726973 ) ) ;
#17225=VERTEX_POINT ( 'NONE', #5214 ) ;
#17229=DIRECTION ( 'NONE',  ( 0.1949050434465281201, -0.6797146636928673713, 0.7071067811865470176 ) ) ;
#17234=CARTESIAN_POINT ( 'NONE',  ( -43.37834615508418068, 1.121909970995877304, 39.54930799450052348 ) ) ;
#17237=CIRCLE ( 'NONE', #3601, 0.9031915329475500576 ) ;
#17242=ORIENTED_EDGE ( 'NONE', *, *, #15481, .T. ) ;
#17245=EDGE_CURVE ( 'NONE', #25249, #26367, #13097, .T. ) ;
#17252=DIRECTION ( 'NONE',  ( 0.000000000000000000, 0.000000000000000000, -1.000000000000000000 ) ) ;
#17254=EDGE_CURVE ( 'NONE', #8280, #30637, #17840, .T. ) ;
#17256=EDGE_CURVE ( 'NONE', #15396, #6997, #24290, .T. ) ;
#17257=DIRECTION ( 'NONE',  ( 0.9612616959383205595, 0.2756373558169932236, -1.660411357259282445E-16 ) ) ;
#17259=PLANE ( 'NONE',  #25750 ) ;
#17260=DIRECTION ( 'NONE',  ( -0.9612616959383206705, -0.2756373558169931681, 1.660411357259282445E-16 ) ) ;
#17262=CARTESIAN_POINT ( 'NONE',  ( -43.29662792673757110, 1.063067023446604864, 60.44930799450051495 ) ) ;
#17263=EDGE_LOOP ( 'NONE', ( #11467, #21305, #32084, #27154 ) ) ;
#17269=AXIS2_PLACEMENT_3D ( 'NONE', #2024, #10239, #20235 ) ;
#17271=ORIENTED_EDGE ( 'NONE', *, *, #4813, .T. ) ;
#17275=ORIENTED_EDGE ( 'NONE', *, *, #14454, .F. ) ;
#17277=CARTESIAN_POINT ( 'NONE',  ( -40.10917099319649282, 6.845611892227015716, 39.49480556904257611 ) ) ;
#17280=LINE ( 'NONE', #10078, #20111 ) ;
#17293=DIRECTION ( 'NONE',  ( 0.8746197071393925215, -0.4848096202463429982, -8.676864087101708112E-18 ) ) ;
#17298=VERTEX_POINT ( 'NONE', #20788 ) ;
#17299=CARTESIAN_POINT ( 'NONE',  ( -40.86270455615213848, 8.492915053331742570, 34.63740864294511823 ) ) ;
#17302=DIRECTION ( 'NONE',  ( -2.779292025043186357E-18, 1.288349127009862211E-17, -1.000000000000000000 ) ) ;
#17308=VECTOR ( 'NONE', #23997, 999.9999999999998863 ) ;
#17309=CARTESIAN_POINT ( 'NONE',  ( -40.02540636251513462, 2.839176264122873050, 37.04930799450052348 ) ) ;
#17313=ORIENTED_EDGE ( 'NONE', *, *, #15165, .F. ) ;
#17315=AXIS2_PLACEMENT_3D ( 'NONE', #9117, #1402, #16335 ) ;
#17316=FACE_OUTER_BOUND ( 'NONE', #5325, .T. ) ;
#17319=EDGE_LOOP ( 'NONE', ( #8878, #15085, #9860, #21654, #17509 ) ) ;
#17336=CARTESIAN_POINT ( 'NONE',  ( -40.28779227465695101, 2.984619150196775816, 37.04930799450052348 ) ) ;
#17337=VECTOR ( 'NONE', #20534, 999.9999999999998863 ) ;
#17340=ORIENTED_EDGE ( 'NONE', *, *, #14912, .F. ) ;
#17341=LINE ( 'NONE', #12109, #10751 ) ;
#17343=ORIENTED_EDGE ( 'NONE', *, *, #30539, .F. ) ;
#17345=CARTESIAN_POINT ( 'NONE',  ( -40.02540636251513462, 2.839176264122873050, 37.04930799450052348 ) ) ;
#17346=VECTOR ( 'NONE', #10270, 1000.000000000000000 ) ;
#17347=VERTEX_POINT ( 'NONE', #6022 ) ;
#17357=VERTEX_POINT ( 'NONE', #18001 ) ;
#17358=VECTOR ( 'NONE', #19748, 999.9999999999998863 ) ;
#17374=ADVANCED_FACE ( 'NONE', ( #26029 ), #1747, .T. ) ;
#17382=ORIENTED_EDGE ( 'NONE', *, *, #29875, .F. ) ;
#17388=CARTESIAN_POINT ( 'NONE',  ( -40.15225626691278649, 6.735663658092487793, 60.54930799450051637 ) ) ;
#17391=TOROIDAL_SURFACE ( 'NONE', #32088, 1.142135311067127068, 0.1000000000000000056 ) ;
#17397=DIRECTION ( 'NONE',  ( 0.3597811455230787714, -0.7883456110718085608, -0.4990678559373643575 ) ) ;
#17399=DIRECTION ( 'NONE',  ( -0.2530443915477366690, 0.8824706660164322036, 0.3965022818682769623 ) ) ;
#17409=AXIS2_PLACEMENT_3D ( 'NONE', #28537, #3739, #1119 ) ;
#17419=FACE_OUTER_BOUND ( 'NONE', #22278, .T. ) ;
#17424=CARTESIAN_POINT ( 'NONE',  ( -40.50726676055796105, 7.559560307024983494, 60.29072935073781991 ) ) ;
#17429=CARTESIAN_POINT ( 'NONE',  ( -40.60086716196818202, 6.831234436378517572, 39.54151698899572409 ) ) ;
#17431=VERTEX_POINT ( 'NONE', #28659 ) ;
#17435=CIRCLE ( 'NONE', #3280, 0.1000000000000007272 ) ;
#17438=ORIENTED_EDGE ( 'NONE', *, *, #18599, .T. ) ;
#17440=CARTESIAN_POINT ( 'NONE',  ( -40.18454328187963398, 7.548069831825862330, 53.64930799450051779 ) ) ;
#17442=ADVANCED_FACE ( 'NONE', ( #23732 ), #28824, .F. ) ;
#17445=CARTESIAN_POINT ( 'NONE',  ( -42.50084779003665147, 14.56798984196178637, 37.04930799450052348 ) ) ;
#17446=DIRECTION ( 'NONE',  ( -0.2756373558169938898, 0.9612616959383203374, 4.550099067471054416E-15 ) ) ;
#17453=EDGE_CURVE ( 'NONE', #20511, #29530, #21140, .T. ) ;
#17457=AXIS2_PLACEMENT_3D ( 'NONE', #21452, #19316, #14255 ) ;
#17461=VECTOR ( 'NONE', #4330, 999.9999999999998863 ) ;
#17463=DIRECTION ( 'NONE',  ( 0.2756373558169954996, -0.9612616959383200044, 2.463803012461673974E-31 ) ) ;
#17468=ORIENTED_EDGE ( 'NONE', *, *, #19142, .T. ) ;
#17480=ORIENTED_EDGE ( 'NONE', *, *, #6155, .F. ) ;
#17481=CARTESIAN_POINT ( 'NONE',  ( -42.38351229602917414, 14.72295342448899191, 58.95959122802360497 ) ) ;
#17482=DIRECTION ( 'NONE',  ( 0.9612616959383221138, 0.2756373558169876170, 0.000000000000000000 ) ) ;
#17489=CARTESIAN_POINT ( 'NONE',  ( -40.65093765668705572, 9.567768634527945792, 38.44930799450052916 ) ) ;
#17493=DIRECTION ( 'NONE',  ( 0.000000000000000000, 0.000000000000000000, 1.000000000000000000 ) ) ;
#17496=ADVANCED_FACE ( 'NONE', ( #26354 ), #13893, .T. ) ;
#17501=EDGE_LOOP ( 'NONE', ( #25264, #27855, #17271, #16990 ) ) ;
#17502=ORIENTED_EDGE ( 'NONE', *, *, #19488, .F. ) ;
#17503=FACE_OUTER_BOUND ( 'NONE', #15178, .T. ) ;
#17509=ORIENTED_EDGE ( 'NONE', *, *, #4945, .T. ) ;
#17511=ORIENTED_EDGE ( 'NONE', *, *, #3804, .F. ) ;
#17516=DIRECTION ( 'NONE',  ( -0.8746197071393805311, 0.4848096202463645921, 8.676864087101954631E-18 ) ) ;
#17521=CARTESIAN_POINT ( 'NONE',  ( -40.02540636251514172, 2.839176264122877047, 55.84930799450052064 ) ) ;
#17522=DIRECTION ( 'NONE',  ( 0.8746197071393926326, -0.4848096202463430537, -8.676864087101709653E-18 ) ) ;
#17523=EDGE_LOOP ( 'NONE', ( #16787, #10151, #3790, #14140 ) ) ;
#17528=ORIENTED_EDGE ( 'NONE', *, *, #9078, .T. ) ;
#17530=ORIENTED_EDGE ( 'NONE', *, *, #16284, .F. ) ;
#17531=CARTESIAN_POINT ( 'NONE',  ( -40.59758774925371938, 7.567737757495683226, 38.19144330556764544 ) ) ;
#17534=VECTOR ( 'NONE', #15122, 1000.000000000000114 ) ;
#17535=ORIENTED_EDGE ( 'NONE', *, *, #16887, .T. ) ;
#17540=CIRCLE ( 'NONE', #24352, 0.1000000000000018235 ) ;
#17548=ORIENTED_EDGE ( 'NONE', *, *, #9944, .F. ) ;
#17553=CARTESIAN_POINT ( 'NONE',  ( -41.94956971822180947, 3.905757428664830222, 49.04930799450051637 ) ) ;
#17567=DIRECTION ( 'NONE',  ( 0.7141240004913198547, -0.3958453973320100738, 0.5773502691896283956 ) ) ;
#17568=EDGE_CURVE ( 'NONE', #21227, #13584, #26404, .T. ) ;
#17572=TOROIDAL_SURFACE ( 'NONE', #12810, 1.299999999999999822, 0.1000000000000000056 ) ;
#17578=ORIENTED_EDGE ( 'NONE', *, *, #12133, .T. ) ;
#17582=CARTESIAN_POINT ( 'NONE',  ( -42.50976151518963064, 14.59907569580870046, 38.09144330556765112 ) ) ;
#17587=FACE_OUTER_BOUND ( 'NONE', #29291, .T. ) ;
#17590=CARTESIAN_POINT ( 'NONE',  ( -40.21210701746133509, 7.644196001419694575, 53.54930799450051637 ) ) ;
#17593=ORIENTED_EDGE ( 'NONE', *, *, #14761, .T. ) ;
#17594=ADVANCED_FACE ( 'NONE', ( #23511 ), #21193, .T. ) ;
#17602=ORIENTED_EDGE ( 'NONE', *, *, #9764, .T. ) ;
#17604=PLANE ( 'NONE',  #22088 ) ;
#17605=LINE ( 'NONE', #7110, #23581 ) ;
#17606=ORIENTED_EDGE ( 'NONE', *, *, #23307, .T. ) ;
#17619=CARTESIAN_POINT ( 'NONE',  ( -39.64148344771002286, 7.657122216028890982, 32.04930799450052348 ) ) ;
#17625=ORIENTED_EDGE ( 'NONE', *, *, #14535, .T. ) ;
#17628=DIRECTION ( 'NONE',  ( -0.8746197071393858602, 0.4848096202463547666, 0.000000000000000000 ) ) ;
#17636=DIRECTION ( 'NONE',  ( -0.1949050434465251780, 0.6797146636928671493, -0.7071067811865480168 ) ) ;
#17638=ORIENTED_EDGE ( 'NONE', *, *, #27993, .F. ) ;
#17642=DIRECTION ( 'NONE',  ( 0.1949050434465268156, -0.6797146636928667052, 0.7071067811865480168 ) ) ;
#17643=DIRECTION ( 'NONE',  ( 0.2756373558169974980, -0.9612616959383193382, -1.315048337272770589E-17 ) ) ;
#17651=EDGE_LOOP ( 'NONE', ( #27430, #103, #15401, #17511 ) ) ;
#17653=CARTESIAN_POINT ( 'NONE',  ( -40.36282785745800794, 8.169822035811970196, 57.04930799450051637 ) ) ;
#17655=VECTOR ( 'NONE', #24173, 999.9999999999998863 ) ;
#17660=DIRECTION ( 'NONE',  ( 0.000000000000000000, 0.000000000000000000, 1.000000000000000000 ) ) ;
#17668=EDGE_CURVE ( 'NONE', #22338, #5664, #9189, .T. ) ;
#17671=DIRECTION ( 'NONE',  ( -0.9612616959383221138, -0.2756373558169876170, 0.000000000000000000 ) ) ;
#17673=CARTESIAN_POINT ( 'NONE',  ( -40.21091586930921125, 6.838981405724006812, 39.54930799450052348 ) ) ;
#17681=ORIENTED_EDGE ( 'NONE', *, *, #13798, .F. ) ;
#17688=VECTOR ( 'NONE', #22694, 1000.000000000000000 ) ;
#17689=ORIENTED_EDGE ( 'NONE', *, *, #12171, .F. ) ;
#17690=AXIS2_PLACEMENT_3D ( 'NONE', #14176, #24170, #4807 ) ;
#17710=CIRCLE ( 'NONE', #3560, 0.1000000000000028644 ) ;
#17711=DIRECTION ( 'NONE',  ( -0.2756373558169946114, 0.9612616959383201154, 2.956675082362952627E-15 ) ) ;
#17714=EDGE_LOOP ( 'NONE', ( #29822, #18099, #17854, #21248, #12878 ) ) ;
#17722=ORIENTED_EDGE ( 'NONE', *, *, #8573, .F. ) ;
#17733=DIRECTION ( 'NONE',  ( -0.8746197071393858602, 0.4848096202463547666, 0.000000000000000000 ) ) ;
#17744=CARTESIAN_POINT ( 'NONE',  ( -43.90780810587784089, -0.03953120679776488122, 61.94930799450052206 ) ) ;
#17745=DIRECTION ( 'NONE',  ( -0.9612616959383194493, -0.2756373558169974980, -8.795445018804946186E-19 ) ) ;
#17746=ADVANCED_FACE ( 'NONE', ( #4348 ), #7135, .T. ) ;
#17764=CARTESIAN_POINT ( 'NONE',  ( -42.38687957179149635, 4.148162238788000167, 38.24930799450051921 ) ) ;
#17765=CARTESIAN_POINT ( 'NONE',  ( -40.50726676055796105, 7.559560307024983494, 60.24930799450051211 ) ) ;
#17773=CARTESIAN_POINT ( 'NONE',  ( -42.66751614955961003, 15.14923148629343785, 38.44930799450052916 ) ) ;
#17775=ORIENTED_EDGE ( 'NONE', *, *, #13391, .F. ) ;
#17785=ORIENTED_EDGE ( 'NONE', *, *, #594, .F. ) ;
#17793=CARTESIAN_POINT ( 'NONE',  ( -40.69454725800886763, 6.788012290873795429, 39.45785194957959874 ) ) ;
#17794=EDGE_LOOP ( 'NONE', ( #8593, #26005, #29785, #15589 ) ) ;
#17798=LINE ( 'NONE', #7643, #16113 ) ;
#17799=DIRECTION ( 'NONE',  ( -0.8746197071393790878, 0.4848096202463673676, 1.277302113040196197E-17 ) ) ;
#17803=ORIENTED_EDGE ( 'NONE', *, *, #9238, .T. ) ;
#17804=CYLINDRICAL_SURFACE ( 'NONE', #29348, 0.1000000000000008243 ) ;
#17806=CIRCLE ( 'NONE', #15205, 2.000000000000001776 ) ;
#17817=EDGE_CURVE ( 'NONE', #28526, #7845, #21235, .T. ) ;
#17819=DIRECTION ( 'NONE',  ( -0.1949050434465252335, 0.6797146636928682595, 0.7071067811865469066 ) ) ;
#17822=VERTEX_POINT ( 'NONE', #19262 ) ;
#17825=CARTESIAN_POINT ( 'NONE',  ( -39.64148344771002286, 7.657122216028890982, 32.04930799450052348 ) ) ;
#17829=ORIENTED_EDGE ( 'NONE', *, *, #29432, .T. ) ;
#17835=DIRECTION ( 'NONE',  ( 0.4848096202463636484, 0.8746197071393810862, 0.000000000000000000 ) ) ;
#17839=PLANE ( 'NONE',  #27858 ) ;
#17840=LINE ( 'NONE', #27863, #19547 ) ;
#17842=AXIS2_PLACEMENT_3D ( 'NONE', #21491, #13970, #23961 ) ;
#17853=EDGE_CURVE ( 'NONE', #15550, #8613, #22717, .T. ) ;
#17854=ORIENTED_EDGE ( 'NONE', *, *, #10861, .F. ) ;
#17855=DIRECTION ( 'NONE',  ( 0.2756373558169932236, -0.9612616959383204485, 1.479773560108267395E-16 ) ) ;
#17856=AXIS2_PLACEMENT_3D ( 'NONE', #29837, #2425, #12441 ) ;
#17859=EDGE_CURVE ( 'NONE', #22591, #1546, #25016, .T. ) ;
#17864=ORIENTED_EDGE ( 'NONE', *, *, #12198, .F. ) ;
#17865=AXIS2_PLACEMENT_3D ( 'NONE', #4134, #19551, #27272 ) ;
#17867=CARTESIAN_POINT ( 'NONE',  ( -41.02687597405218156, 7.220473278338834788, 60.54930799450051637 ) ) ;
#17875=EDGE_LOOP ( 'NONE', ( #22980, #22557, #32294, #19724 ) ) ;
#17880=CYLINDRICAL_SURFACE ( 'NONE', #15219, 0.1000000000000028644 ) ;
#17891=EDGE_CURVE ( 'NONE', #19940, #28859, #383, .T. ) ;
#17898=( BOUNDED_CURVE ( )  B_SPLINE_CURVE ( 3, ( #12132, #6708, #16706, #7197 ),
 .UNSPECIFIED., .F., .F. ) 
 B_SPLINE_CURVE_WITH_KNOTS ( ( 4, 4 ),
 ( 0.4372979894901917186, 1.133349320028354423 ),
 .UNSPECIFIED. ) 
 CURVE ( )  GEOMETRIC_REPRESENTATION_ITEM ( )  RATIONAL_B_SPLINE_CURVE ( ( 1.000000000000000000, 0.9600319177481759780, 0.9600319177481759780, 1.000000000000000000 ) ) 
 REPRESENTATION_ITEM ( '' )  );
#17900=EDGE_CURVE ( 'NONE', #1639, #21428, #27796, .T. ) ;
#17901=VERTEX_POINT ( 'NONE', #20089 ) ;
#17902=VERTEX_POINT ( 'NONE', #4838 ) ;
#17906=ORIENTED_EDGE ( 'NONE', *, *, #2850, .T. ) ;
#17908=CARTESIAN_POINT ( 'NONE',  ( -41.24971778908466291, 11.62557032131817358, 57.04930799450051637 ) ) ;
#17909=DIRECTION ( 'NONE',  ( -0.9612616959383221138, -0.2756373558169876170, 0.000000000000000000 ) ) ;
#17922=CIRCLE ( 'NONE', #16856, 0.09999999999999700795 ) ;
#17932=CARTESIAN_POINT ( 'NONE',  ( -40.70217169293940884, 9.596168124565080504, 35.54930799450051637 ) ) ;
#17945=LINE ( 'NONE', #15961, #1797 ) ;
#17947=CIRCLE ( 'NONE', #20573, 1.300000000000002487 ) ;
#17948=ORIENTED_EDGE ( 'NONE', *, *, #16734, .T. ) ;
#17951=DIRECTION ( 'NONE',  ( 0.8746197071393926326, -0.4848096202463430537, -8.676864087101709653E-18 ) ) ;
#17957=CARTESIAN_POINT ( 'NONE',  ( -40.11286833322908052, 2.887657226147511302, 57.04930799450051637 ) ) ;
#17961=ORIENTED_EDGE ( 'NONE', *, *, #22025, .F. ) ;
#17962=CARTESIAN_POINT ( 'NONE',  ( -42.50976151518963064, 14.59907569580870046, 37.04930799450052348 ) ) ;
#17970=ORIENTED_EDGE ( 'NONE', *, *, #8532, .T. ) ;
#17971=CARTESIAN_POINT ( 'NONE',  ( -40.44300931641782171, 7.361061430353638357, 60.31640775708849844 ) ) ;
#17976=EDGE_CURVE ( 'NONE', #2645, #29624, #804, .T. ) ;
#17977=EDGE_CURVE ( 'NONE', #21227, #3106, #24925, .T. ) ;
#17979=CIRCLE ( 'NONE', #22712, 0.09999999999999945044 ) ;
#17988=CARTESIAN_POINT ( 'NONE',  ( -40.50720532202722524, 7.584939507552747706, 60.08350751967648762 ) ) ;
#18001=CARTESIAN_POINT ( 'NONE',  ( -40.46271621608484281, 3.081581074246047436, 45.54930799450051637 ) ) ;
#18011=EDGE_CURVE ( 'NONE', #1187, #13517, #15646, .T. ) ;
#18016=VERTEX_POINT ( 'NONE', #18579 ) ;
#18017=AXIS2_PLACEMENT_3D ( 'NONE', #18417, #864, #11205 ) ;
#18029=LINE ( 'NONE', #28055, #6399 ) ;
#18031=EDGE_CURVE ( 'NONE', #7358, #15249, #1111, .T. ) ;
#18046=DIRECTION ( 'NONE',  ( 0.2756373558169962767, -0.9612616959383197823, 1.479773560108262218E-16 ) ) ;
#18048=EDGE_LOOP ( 'NONE', ( #19955, #2274, #5850, #2084, #9310, #7016, #31758, #8149 ) ) ;
#18051=FACE_OUTER_BOUND ( 'NONE', #25560, .T. ) ;
#18058=FACE_BOUND ( 'NONE', #9179, .T. ) ;
#18066=ADVANCED_FACE ( 'NONE', ( #23685 ), #15493, .T. ) ;
#18068=EDGE_CURVE ( 'NONE', #28859, #16068, #26904, .T. ) ;
#18070=DIRECTION ( 'NONE',  ( -1.188208965918165239E-16, -1.880121038077813132E-16, -1.000000000000000000 ) ) ;
#18071=CARTESIAN_POINT ( 'NONE',  ( -39.58809650894544774, 2.596771453999702661, 45.14930799450051779 ) ) ;
#18078=DIRECTION ( 'NONE',  ( 0.9612616959383205595, 0.2756373558169932236, -1.660411357259282445E-16 ) ) ;
#18079=ADVANCED_FACE ( 'NONE', ( #23362 ), #10895, .T. ) ;
#18082=VECTOR ( 'NONE', #9677, 999.9999999999998863 ) ;
#18084=( BOUNDED_CURVE ( )  B_SPLINE_CURVE ( 3, ( #20641, #28193, #30665, #10810 ),
 .UNSPECIFIED., .F., .F. ) 
 B_SPLINE_CURVE_WITH_KNOTS ( ( 4, 4 ),
 ( 1.570796326794906994, 2.992702705980325284 ),
 .UNSPECIFIED. ) 
 CURVE ( )  GEOMETRIC_REPRESENTATION_ITEM ( )  RATIONAL_B_SPLINE_CURVE ( ( 1.000000000000000000, 0.8384934736035529745, 0.8384934736035529745, 1.000000000000000000 ) ) 
 REPRESENTATION_ITEM ( '' )  );
#18089=DIRECTION ( 'NONE',  ( 0.9612616959383205595, 0.2756373558169931681, -1.660411357259282445E-16 ) ) ;
#18099=ORIENTED_EDGE ( 'NONE', *, *, #7846, .T. ) ;
#18107=CARTESIAN_POINT ( 'NONE',  ( -41.93344242462055149, 13.82826554927148166, 54.56265170360538264 ) ) ;
#18113=ORIENTED_EDGE ( 'NONE', *, *, #11095, .T. ) ;
#18115=DIRECTION ( 'NONE',  ( -2.779292025043186357E-18, 1.288349127009862211E-17, -1.000000000000000000 ) ) ;
#18122=ORIENTED_EDGE ( 'NONE', *, *, #7421, .F. ) ;
#18123=CARTESIAN_POINT ( 'NONE',  ( -38.36853489569023168, 7.065850718397948427, 61.94930799450052206 ) ) ;
#18125=CARTESIAN_POINT ( 'NONE',  ( -40.62123369608615775, 7.650200974017423050, 34.54930799450052348 ) ) ;
#18135=ORIENTED_EDGE ( 'NONE', *, *, #6814, .T. ) ;
#18148=ORIENTED_EDGE ( 'NONE', *, *, #27282, .F. ) ;
#18151=ORIENTED_EDGE ( 'NONE', *, *, #11527, .T. ) ;
#18152=DIRECTION ( 'NONE',  ( -0.1651779284337324960, 0.9862637841664575467, -1.082442759285643960E-14 ) ) ;
#18153=EDGE_CURVE ( 'NONE', #5962, #8855, #7579, .T. ) ;
#18158=EDGE_CURVE ( 'NONE', #13775, #8613, #14986, .T. ) ;
#18162=CARTESIAN_POINT ( 'NONE',  ( -40.70484894842233103, 8.274204744976163539, 59.64930799450051779 ) ) ;
#18167=VECTOR ( 'NONE', #19383, 1000.000000000000114 ) ;
#18169=ORIENTED_EDGE ( 'NONE', *, *, #747, .F. ) ;
#18176=ADVANCED_FACE ( 'NONE', ( #23995 ), #16930, .T. ) ;
#18185=ORIENTED_EDGE ( 'NONE', *, *, #3404, .F. ) ;
#18188=DIRECTION ( 'NONE',  ( 0.8746197071393925215, -0.4848096202463429982, -8.676864087101708112E-18 ) ) ;
#18191=CARTESIAN_POINT ( 'NONE',  ( -40.11286833322907341, 2.887657226147507306, 37.04930799450052348 ) ) ;
#18193=ORIENTED_EDGE ( 'NONE', *, *, #4412, .F. ) ;
#18195=AXIS2_PLACEMENT_3D ( 'NONE', #23661, #20711, #26284 ) ;
#18201=CARTESIAN_POINT ( 'NONE',  ( -41.93344242462055149, 13.82826554927147988, 59.53596428539564300 ) ) ;
#18216=AXIS2_PLACEMENT_3D ( 'NONE', #8687, #28697, #1279 ) ;
#18222=CARTESIAN_POINT ( 'NONE',  ( -41.01929587258828747, 9.401204285752060130, 39.44930799450052206 ) ) ;
#18223=CARTESIAN_POINT ( 'NONE',  ( -40.59758774925371938, 7.567737757495682338, 35.64930799450052490 ) ) ;
#18226=DIRECTION ( 'NONE',  ( 0.9612616959383221138, 0.2756373558169876170, 0.000000000000000000 ) ) ;
#18229=ORIENTED_EDGE ( 'NONE', *, *, #26893, .T. ) ;
#18235=CARTESIAN_POINT ( 'NONE',  ( -40.23847961986563604, 6.935107571023907624, 39.46426056150422568 ) ) ;
#18236=ORIENTED_EDGE ( 'NONE', *, *, #29391, .T. ) ;
#18242=AXIS2_PLACEMENT_3D ( 'NONE', #5495, #23212, #728 ) ;
#18250=ADVANCED_FACE ( 'NONE', ( #24817 ), #27765, .T. ) ;
#18253=CARTESIAN_POINT ( 'NONE',  ( -43.64647580959332629, 1.256990871545142774, 60.44930799450051495 ) ) ;
#18259=CARTESIAN_POINT ( 'NONE',  ( -41.08785830660042393, 9.277514380576530328, 38.60788663826321709 ) ) ;
#18262=FACE_OUTER_BOUND ( 'NONE', #18972, .T. ) ;
#18273=FACE_OUTER_BOUND ( 'NONE', #32298, .T. ) ;
#18277=DIRECTION ( 'NONE',  ( 1.188208965918164993E-16, 1.880121038077812639E-16, 1.000000000000000000 ) ) ;
#18280=PLANE ( 'NONE',  #6795 ) ;
#18284=FACE_OUTER_BOUND ( 'NONE', #23199, .T. ) ;
#18286=ADVANCED_FACE ( 'NONE', ( #12687 ), #28551, .T. ) ;
#18296=CARTESIAN_POINT ( 'NONE',  ( -42.50084779003665147, 14.56798984196178637, 37.04930799450052348 ) ) ;
#18299=CARTESIAN_POINT ( 'NONE',  ( -40.54828680531408480, 6.846271790121642553, 34.54930799450052348 ) ) ;
#18307=VERTEX_POINT ( 'NONE', #9724 ) ;
#18309=CARTESIAN_POINT ( 'NONE',  ( -40.60722745863126448, 9.415333058485025219, 39.40788663826321425 ) ) ;
#18310=CIRCLE ( 'NONE', #9391, 0.09999999999999795164 ) ;
#18315=CYLINDRICAL_SURFACE ( 'NONE', #1576, 0.1000000000000014905 ) ;
#18317=CARTESIAN_POINT ( 'NONE',  ( -42.36153388572594736, 13.68895619636815653, 60.54930799450051637 ) ) ;
#18319=CARTESIAN_POINT ( 'NONE',  ( -42.47434154250543514, 4.196643200812633978, 38.34930799450052064 ) ) ;
#18320=CARTESIAN_POINT ( 'NONE',  ( -40.62190982259030392, 6.851786633711440366, 34.76984793051720857 ) ) ;
#18326=ORIENTED_EDGE ( 'NONE', *, *, #31424, .F. ) ;
#18330=AXIS2_PLACEMENT_3D ( 'NONE', #13384, #20909, #30457 ) ;
#18337=ORIENTED_EDGE ( 'NONE', *, *, #11222, .F. ) ;
#18338=FACE_OUTER_BOUND ( 'NONE', #12593, .T. ) ;
#18339=CIRCLE ( 'NONE', #29895, 1.199999999999999734 ) ;
#18340=VECTOR ( 'NONE', #28087, 1000.000000000000000 ) ;
#18351=DIRECTION ( 'NONE',  ( 0.8746197071393927436, -0.4848096202463423876, -1.277302113040827440E-17 ) ) ;
#18352=LINE ( 'NONE', #805, #21757 ) ;
#18356=ORIENTED_EDGE ( 'NONE', *, *, #27262, .T. ) ;
#18360=CARTESIAN_POINT ( 'NONE',  ( -40.23672901771082877, 7.760455916344221272, 39.54930799450052348 ) ) ;
#18366=ORIENTED_EDGE ( 'NONE', *, *, #14312, .T. ) ;
#18369=AXIS2_PLACEMENT_3D ( 'NONE', #2948, #27585, #28072 ) ;
#18373=ADVANCED_FACE ( 'NONE', ( #30880 ), #14393, .T. ) ;
#18376=EDGE_CURVE ( 'NONE', #14105, #13215, #4471, .T. ) ;
#18379=DIRECTION ( 'NONE',  ( -1.188208965918165239E-16, -1.880121038077813132E-16, -1.000000000000000000 ) ) ;
#18380=AXIS2_PLACEMENT_3D ( 'NONE', #7018, #11784, #17012 ) ;
#18382=CARTESIAN_POINT ( 'NONE',  ( -41.59479728461646175, 12.46621001045476973, 57.04930799450051637 ) ) ;
#18388=CARTESIAN_POINT ( 'NONE',  ( -41.94323192092819852, 13.80701548633532560, 59.54475713566544215 ) ) ;
#18393=CARTESIAN_POINT ( 'NONE',  ( -40.65487266620045403, 9.475231293617264683, 38.63717596014456035 ) ) ;
#18395=ORIENTED_EDGE ( 'NONE', *, *, #7539, .F. ) ;
#18396=ORIENTED_EDGE ( 'NONE', *, *, #30539, .T. ) ;
#18399=DIRECTION ( 'NONE',  ( 0.8746197071393926326, -0.4848096202463430537, -8.676864087101709653E-18 ) ) ;
#18404=DIRECTION ( 'NONE',  ( -7.588956326749211550E-18, 4.206627182996911684E-18, -1.000000000000000000 ) ) ;
#18405=VERTEX_POINT ( 'NONE', #27928 ) ;
#18409=EDGE_CURVE ( 'NONE', #28788, #14105, #5448, .T. ) ;
#18415=EDGE_CURVE ( 'NONE', #32106, #2831, #21009, .T. ) ;
#18416=DIRECTION ( 'NONE',  ( 0.4848096202463424431, 0.8746197071393927436, -2.220446049250312588E-16 ) ) ;
#18417=CARTESIAN_POINT ( 'NONE',  ( -42.38687957179150345, 4.148162238788003719, 58.34930799450052064 ) ) ;
#18419=DIRECTION ( 'NONE',  ( 0.2756373558169932236, -0.9612616959383204485, 1.479773560108267395E-16 ) ) ;
#18423=ORIENTED_EDGE ( 'NONE', *, *, #3933, .T. ) ;
#18431=DIRECTION ( 'NONE',  ( 0.8746197071393858602, -0.4848096202463547666, 0.000000000000000000 ) ) ;
#18435=AXIS2_PLACEMENT_3D ( 'NONE', #24952, #8047, #2464 ) ;
#18438=VERTEX_POINT ( 'NONE', #3619 ) ;
#18442=LINE ( 'NONE', #20750, #22737 ) ;
#18455=VERTEX_POINT ( 'NONE', #30561 ) ;
#18456=AXIS2_PLACEMENT_3D ( 'NONE', #24484, #1677, #31878 ) ;
#18458=AXIS2_PLACEMENT_3D ( 'NONE', #13600, #640, #10672 ) ;
#18463=ORIENTED_EDGE ( 'NONE', *, *, #11202, .T. ) ;
#18464=CARTESIAN_POINT ( 'NONE',  ( -42.59587854516874472, -0.7667456371672803916, 32.14930799450051779 ) ) ;
#18467=DIRECTION ( 'NONE',  ( 0.4848096202463430537, 0.8746197071393926326, 1.323854077651070671E-16 ) ) ;
#18478=DIRECTION ( 'NONE',  ( -7.588956326749211550E-18, 4.206627182996912454E-18, -1.000000000000000000 ) ) ;
#18479=DIRECTION ( 'NONE',  ( 0.9612616959383205595, 0.2756373558169932236, -1.660411357259282445E-16 ) ) ;
#18481=DIRECTION ( 'NONE',  ( -2.779292025043186357E-18, 1.288349127009862211E-17, -1.000000000000000000 ) ) ;
#18484=CARTESIAN_POINT ( 'NONE',  ( -40.59758774925372649, 7.567737757495682338, 35.43807061034478778 ) ) ;
#18488=EDGE_CURVE ( 'NONE', #25031, #20784, #23317, .T. ) ;
#18495=ORIENTED_EDGE ( 'NONE', *, *, #16036, .F. ) ;
#18496=VECTOR ( 'NONE', #13606, 1000.000000000000114 ) ;
#18499=CARTESIAN_POINT ( 'NONE',  ( -42.50976151518963064, 14.59907569580870046, 37.04930799450052348 ) ) ;
#18510=DIRECTION ( 'NONE',  ( -0.2756373558169932236, 0.9612616959383204485, -1.479773560108267395E-16 ) ) ;
#18513=CARTESIAN_POINT ( 'NONE',  ( -39.55402147699608406, 7.608641254004257171, 32.04930799450052348 ) ) ;
#18517=DIRECTION ( 'NONE',  ( 0.9612616959383193382, 0.2756373558169973870, 8.795445018804930779E-19 ) ) ;
#18518=EDGE_CURVE ( 'NONE', #30739, #13675, #17341, .T. ) ;
#18523=EDGE_CURVE ( 'NONE', #30888, #18712, #17007, .T. ) ;
#18524=DIRECTION ( 'NONE',  ( -0.9612616959383200044, -0.2756373558169954996, 1.660411357259285896E-16 ) ) ;
#18527=DIRECTION ( 'NONE',  ( -0.1949050434465271764, 0.6797146636928685925, -0.7071067811865460184 ) ) ;
#18528=AXIS2_PLACEMENT_3D ( 'NONE', #29971, #7484, #17482 ) ;
#18539=ORIENTED_EDGE ( 'NONE', *, *, #22018, .F. ) ;
#18540=DIRECTION ( 'NONE',  ( 0.1949050434465252335, -0.6797146636928682595, -0.7071067811865469066 ) ) ;
#18541=VERTEX_POINT ( 'NONE', #4385 ) ;
#18546=( LENGTH_UNIT ( ) NAMED_UNIT ( * ) SI_UNIT ( .MILLI., .METRE. ) );
#18556=CARTESIAN_POINT ( 'NONE',  ( -41.94956971822180947, 3.905757428664828890, 47.04930799450051637 ) ) ;
#18560=DIRECTION ( 'NONE',  ( -0.2756373558169932236, 0.9612616959383204485, -1.479773560108267395E-16 ) ) ;
#18564=TOROIDAL_SURFACE ( 'NONE', #3363, 0.8928932188134564019, 0.1000000000000000056 ) ;
#18565=VECTOR ( 'NONE', #30156, 1000.000000000000227 ) ;
#18568=CIRCLE ( 'NONE', #1283, 2.000000000000001776 ) ;
#18569=ORIENTED_EDGE ( 'NONE', *, *, #10821, .T. ) ;
#18571=CARTESIAN_POINT ( 'NONE',  ( -40.59758774925371938, 7.567737757495682338, 35.43807061034478778 ) ) ;
#18579=CARTESIAN_POINT ( 'NONE',  ( -42.48178708409979265, 14.60617548783703690, 58.99727659774876543 ) ) ;
#18580=DIRECTION ( 'NONE',  ( 0.4848096202463637039, 0.8746197071393810862, 0.000000000000000000 ) ) ;
#18582=VECTOR ( 'NONE', #11659, 1000.000000000000114 ) ;
#18586=EDGE_LOOP ( 'NONE', ( #13695, #12984, #21094, #12732 ) ) ;
#18596=DIRECTION ( 'NONE',  ( -0.1949050434465282311, 0.6797146636928672603, -0.7071067811865469066 ) ) ;
#18599=EDGE_CURVE ( 'NONE', #3050, #13764, #15979, .T. ) ;
#18614=DIRECTION ( 'NONE',  ( -0.4848096202463429982, -0.8746197071393925215, -9.920727850371698576E-18 ) ) ;
#18622=VERTEX_POINT ( 'NONE', #22756 ) ;
#18625=DIRECTION ( 'NONE',  ( 0.000000000000000000, 0.000000000000000000, -1.000000000000000000 ) ) ;
#18630=DIRECTION ( 'NONE',  ( -2.779292025043186357E-18, 1.288349127009862211E-17, -1.000000000000000000 ) ) ;
#18639=VERTEX_POINT ( 'NONE', #28014 ) ;
#18644=ORIENTED_EDGE ( 'NONE', *, *, #31395, .T. ) ;
#18645=ORIENTED_EDGE ( 'NONE', *, *, #8459, .T. ) ;
#18649=ADVANCED_BREP_SHAPE_REPRESENTATION ( '', ( #1854, #8172 ), #12388 ) ;
#18654=AXIS2_PLACEMENT_3D ( 'NONE', #24130, #29387, #28911 ) ;
#18656=ADVANCED_FACE ( 'NONE', ( #10298 ), #7053, .T. ) ;
#18669=CARTESIAN_POINT ( 'NONE',  ( -40.57420052961184354, 7.102220148652932608, 38.86693366820416884 ) ) ;
#18670=CARTESIAN_POINT ( 'NONE',  ( -40.69423955692156625, 6.789232590171205395, 39.42520008276828491 ) ) ;
#18672=CARTESIAN_POINT ( 'NONE',  ( -40.08841711228579641, 7.575633567407562552, 53.54930799450051637 ) ) ;
#18673=CARTESIAN_POINT ( 'NONE',  ( -40.16174044770769314, 7.468546898574135895, 53.54930799450051637 ) ) ;
#18676=CARTESIAN_POINT ( 'NONE',  ( -40.16174044770769314, 7.468546898574136783, 54.64930799450051779 ) ) ;
#18693=ORIENTED_EDGE ( 'NONE', *, *, #21076, .F. ) ;
#18702=CARTESIAN_POINT ( 'NONE',  ( -43.37834615508418068, 1.121909970995877082, 39.54930799450052348 ) ) ;
#18703=CARTESIAN_POINT ( 'NONE',  ( -40.69571722278732295, 6.786566810383045656, 34.64930799450051779 ) ) ;
#18706=CARTESIAN_POINT ( 'NONE',  ( -40.23397449525940317, 6.794506605641764452, 39.44930799450052206 ) ) ;
#18707=DIRECTION ( 'NONE',  ( 0.1949050434465252335, -0.6797146636928682595, -0.7071067811865469066 ) ) ;
#18709=DIRECTION ( 'NONE',  ( -0.6184495258776564475, 0.3428121700606708289, -0.7071067811865443531 ) ) ;
#18710=PLANE ( 'NONE',  #18820 ) ;
#18712=VERTEX_POINT ( 'NONE', #28500 ) ;
#18718=AXIS2_PLACEMENT_3D ( 'NONE', #4070, #9169, #19325 ) ;
#18725=CIRCLE ( 'NONE', #4599, 0.2000000000000012601 ) ;
#18726=ORIENTED_EDGE ( 'NONE', *, *, #24260, .F. ) ;
#18728=EDGE_CURVE ( 'NONE', #15237, #16253, #21209, .T. ) ;
#18735=EDGE_LOOP ( 'NONE', ( #12031, #1805, #9792, #10119 ) ) ;
#18736=FACE_OUTER_BOUND ( 'NONE', #30701, .T. ) ;
#18739=CARTESIAN_POINT ( 'NONE',  ( -40.58856461370174884, 7.499380836222963254, 60.14930799450051779 ) ) ;
#18746=CARTESIAN_POINT ( 'NONE',  ( -40.11553135844172147, 6.871094863070437597, 34.58253047105350220 ) ) ;
#18748=CARTESIAN_POINT ( 'NONE',  ( -39.58809650894544774, 2.596771453999702661, 47.04930799450051637 ) ) ;
#18753=VECTOR ( 'NONE', #12125, 999.9999999999998863 ) ;
#18759=ORIENTED_EDGE ( 'NONE', *, *, #15632, .T. ) ;
#18766=VECTOR ( 'NONE', #4105, 1000.000000000000114 ) ;
#18769=AXIS2_PLACEMENT_3D ( 'NONE', #28518, #25243, #15707 ) ;
#18770=CARTESIAN_POINT ( 'NONE',  ( -42.28293707589220674, 13.65198258188957148, 59.54475713566496609 ) ) ;
#18776=DIRECTION ( 'NONE',  ( 0.2756373558170082672, -0.9612616959383162296, 0.000000000000000000 ) ) ;
#18788=PLANE ( 'NONE',  #3685 ) ;
#18791=CARTESIAN_POINT ( 'NONE',  ( -40.12089182904525586, 6.795442088152954696, 34.54930799450050927 ) ) ;
#18792=CARTESIAN_POINT ( 'NONE',  ( -40.64264863745435719, 6.822556421824200967, 34.67218454412468986 ) ) ;
#18797=FACE_OUTER_BOUND ( 'NONE', #27187, .T. ) ;
#18798=CIRCLE ( 'NONE', #4071, 1.300000000000002487 ) ;
#18803=VECTOR ( 'NONE', #17229, 1000.000000000000000 ) ;
#18805=VERTEX_POINT ( 'NONE', #3377 ) ;
#18806=ADVANCED_FACE ( 'NONE', ( #16170 ), #13410, .T. ) ;
#18810=CARTESIAN_POINT ( 'NONE',  ( -42.30123736278718383, 13.66041317296246937, 59.53596428539564300 ) ) ;
#18812=DIRECTION ( 'NONE',  ( 0.000000000000000000, 0.000000000000000000, -1.000000000000000000 ) ) ;
#18820=AXIS2_PLACEMENT_3D ( 'NONE', #19367, #21501, #14302 ) ;
#18823=CARTESIAN_POINT ( 'NONE',  ( -40.68984688381694070, 6.797157182225249450, 39.37314909236572191 ) ) ;
#18828=DIRECTION ( 'NONE',  ( 0.4848096202463506588, 0.8746197071393884137, 9.920727850371624621E-18 ) ) ;
#18832=AXIS2_PLACEMENT_3D ( 'NONE', #1529, #8607, #24177 ) ;
#18835=ADVANCED_FACE ( 'NONE', ( #26181 ), #1394, .T. ) ;
#18836=DIRECTION ( 'NONE',  ( 0.2756373558169970539, -0.9612616959383194493, -1.315048337272770435E-17 ) ) ;
#18843=EDGE_CURVE ( 'NONE', #11316, #7874, #21758, .T. ) ;
#18845=EDGE_CURVE ( 'NONE', #5658, #17034, #25425, .T. ) ;
#18847=ORIENTED_EDGE ( 'NONE', *, *, #30138, .T. ) ;
#18849=VECTOR ( 'NONE', #9021, 1000.000000000000000 ) ;
#18862=DIRECTION ( 'NONE',  ( 0.8746197071393925215, -0.4848096202463429982, -8.676864087101708112E-18 ) ) ;
#18870=VERTEX_POINT ( 'NONE', #14530 ) ;
#18872=CARTESIAN_POINT ( 'NONE',  ( -42.38687957179150345, 4.148162238788003719, 57.04930799450051637 ) ) ;
#18876=ORIENTED_EDGE ( 'NONE', *, *, #1074, .T. ) ;
#18880=ORIENTED_EDGE ( 'NONE', *, *, #7815, .F. ) ;
#18888=CIRCLE ( 'NONE', #23104, 1.199999999999999734 ) ;
#18892=DIRECTION ( 'NONE',  ( 0.8746197071393926326, -0.4848096202463430537, -8.676864087101709653E-18 ) ) ;
#18894=VECTOR ( 'NONE', #12737, 1000.000000000000227 ) ;
#18895=ORIENTED_EDGE ( 'NONE', *, *, #3600, .F. ) ;
#18897=AXIS2_PLACEMENT_3D ( 'NONE', #4465, #31876, #16599 ) ;
#18904=CARTESIAN_POINT ( 'NONE',  ( -40.60333149162104860, 7.557375771971039491, 54.01510846932453092 ) ) ;
#18914=ORIENTED_EDGE ( 'NONE', *, *, #6801, .T. ) ;
#18915=DIRECTION ( 'NONE',  ( 0.4848096202463673121, 0.8746197071393789768, 0.000000000000000000 ) ) ;
#18916=DIRECTION ( 'NONE',  ( -0.2756373558169930016, 0.9612616959383205595, 1.315048337272770743E-17 ) ) ;
#18921=CARTESIAN_POINT ( 'NONE',  ( -43.64073206722599707, 1.267352857069779848, 39.54930799450052348 ) ) ;
#18923=DIRECTION ( 'NONE',  ( 0.000000000000000000, 0.000000000000000000, 1.000000000000000000 ) ) ;
#18929=VECTOR ( 'NONE', #4195, 1000.000000000000000 ) ;
#18931=( BOUNDED_CURVE ( )  B_SPLINE_CURVE ( 3, ( #22808, #2304, #4597, #25115 ),
 .UNSPECIFIED., .F., .F. ) 
 B_SPLINE_CURVE_WITH_KNOTS ( ( 4, 4 ),
 ( 0.1488899476094779073, 1.570796326794886344 ),
 .UNSPECIFIED. ) 
 CURVE ( )  GEOMETRIC_REPRESENTATION_ITEM ( )  RATIONAL_B_SPLINE_CURVE ( ( 1.000000000000000000, 0.8384934736035551950, 0.8384934736035551950, 1.000000000000000000 ) ) 
 REPRESENTATION_ITEM ( '' )  );
#18942=DIRECTION ( 'NONE',  ( -0.9612616959383200044, -0.2756373558169954996, 1.660411357259285896E-16 ) ) ;
#18947=( LENGTH_UNIT ( ) NAMED_UNIT ( * ) SI_UNIT ( .MILLI., .METRE. ) );
#18956=EDGE_LOOP ( 'NONE', ( #19459, #20999, #7855, #30466, #21271 ) ) ;
#18957=LINE ( 'NONE', #14059, #1467 ) ;
#18961=EDGE_CURVE ( 'NONE', #6997, #15396, #4476, .T. ) ;
#18963=ORIENTED_EDGE ( 'NONE', *, *, #10905, .T. ) ;
#18964=ADVANCED_FACE ( 'NONE', ( #14371, #31604 ), #29297, .F. ) ;
#18966=EDGE_CURVE ( 'NONE', #12082, #17901, #31926, .T. ) ;
#18972=EDGE_LOOP ( 'NONE', ( #13125, #32479, #8443 ) ) ;
#18973=CARTESIAN_POINT ( 'NONE',  ( -40.70484894842233103, 8.274204744976163539, 54.64930799450051779 ) ) ;
#18977=CARTESIAN_POINT ( 'NONE',  ( -40.31405849284424647, 8.392931372713462679, 40.47149053519531492 ) ) ;
#18996=ORIENTED_EDGE ( 'NONE', *, *, #11827, .F. ) ;
#18997=CARTESIAN_POINT ( 'NONE',  ( -40.38516919650994197, 8.640923867788874446, 39.54930799450052348 ) ) ;
#18999=DIRECTION ( 'NONE',  ( 0.2756373558169958327, -0.9612616959383198934, 0.000000000000000000 ) ) ;
#19002=VERTEX_POINT ( 'NONE', #24530 ) ;
#19003=CYLINDRICAL_SURFACE ( 'NONE', #12475, 2.000000000000001776 ) ;
#19005=FACE_OUTER_BOUND ( 'NONE', #10484, .T. ) ;
#19012=ORIENTED_EDGE ( 'NONE', *, *, #22578, .T. ) ;
#19019=DIRECTION ( 'NONE',  ( 0.3428121700606686084, 0.6184495258776648852, -0.7071067811865382469 ) ) ;
#19024=CARTESIAN_POINT ( 'NONE',  ( -43.86407712052087504, -0.06377168781008255016, 32.09930799450052064 ) ) ;
#19032=EDGE_LOOP ( 'NONE', ( #21470, #4066, #21934, #15046 ) ) ;
#19038=AXIS2_PLACEMENT_3D ( 'NONE', #17773, #27136, #20236 ) ;
#19043=CARTESIAN_POINT ( 'NONE',  ( -42.38687957179150345, 4.148162238788003719, 57.04930799450051637 ) ) ;
#19047=ORIENTED_EDGE ( 'NONE', *, *, #15045, .T. ) ;
#19051=CYLINDRICAL_SURFACE ( 'NONE', #13148, 2.000000000000001776 ) ;
#19057=DIRECTION ( 'NONE',  ( 0.8746197071393929656, -0.4848096202463424986, 7.034541100025353118E-15 ) ) ;
#19080=CARTESIAN_POINT ( 'NONE',  ( -42.60588768478345401, 14.57151196022700113, 37.04930799450052348 ) ) ;
#19081=AXIS2_PLACEMENT_3D ( 'NONE', #10580, #13365, #25505 ) ;
#19084=AXIS2_PLACEMENT_3D ( 'NONE', #25614, #15766, #3284 ) ;
#19088=ORIENTED_EDGE ( 'NONE', *, *, #24603, .T. ) ;
#19115=ORIENTED_EDGE ( 'NONE', *, *, #24865, .T. ) ;
#19121=ORIENTED_EDGE ( 'NONE', *, *, #28400, .F. ) ;
#19123=( BOUNDED_CURVE ( )  B_SPLINE_CURVE ( 3, ( #5921, #6077, #16238, #8068 ),
 .UNSPECIFIED., .F., .F. ) 
 B_SPLINE_CURVE_WITH_KNOTS ( ( 4, 4 ),
 ( -8.881784197001252323E-16, 1.570796326794894782 ),
 .UNSPECIFIED. ) 
 CURVE ( )  GEOMETRIC_REPRESENTATION_ITEM ( )  RATIONAL_B_SPLINE_CURVE ( ( 1.000000000000000000, 0.8047378541243652705, 0.8047378541243652705, 1.000000000000000000 ) ) 
 REPRESENTATION_ITEM ( '' )  );
#19124=ORIENTED_EDGE ( 'NONE', *, *, #9040, .T. ) ;
#19125=CIRCLE ( 'NONE', #14959, 0.9031915329475500576 ) ;
#19130=CARTESIAN_POINT ( 'NONE',  ( -40.18454328187963398, 7.548069831825862330, 60.54930799450051637 ) ) ;
#19137=LINE ( 'NONE', #14240, #27190 ) ;
#19138=ADVANCED_FACE ( 'NONE', ( #28462 ), #23841, .F. ) ;
#19141=ADVANCED_FACE ( 'NONE', ( #5646 ), #1043, .F. ) ;
#19142=EDGE_CURVE ( 'NONE', #32001, #28526, #24935, .T. ) ;
#19144=ORIENTED_EDGE ( 'NONE', *, *, #27599, .F. ) ;
#19148=DIRECTION ( 'NONE',  ( -0.9612616959383210036, -0.2756373558169918914, -9.967286752943808104E-15 ) ) ;
#19151=PLANE ( 'NONE',  #13691 ) ;
#19152=CARTESIAN_POINT ( 'NONE',  ( -40.64522151305494191, 6.818818762547858014, 39.52645928364133709 ) ) ;
#19153=AXIS2_PLACEMENT_3D ( 'NONE', #22674, #12842, #2333 ) ;
#19157=LINE ( 'NONE', #31809, #27309 ) ;
#19159=ORIENTED_EDGE ( 'NONE', *, *, #12988, .T. ) ;
#19161=LINE ( 'NONE', #21299, #1988 ) ;
#19162=FACE_OUTER_BOUND ( 'NONE', #23751, .T. ) ;
#19170=FACE_OUTER_BOUND ( 'NONE', #17875, .T. ) ;
#19173=VECTOR ( 'NONE', #17397, 1000.000000000000114 ) ;
#19175=ORIENTED_EDGE ( 'NONE', *, *, #14875, .T. ) ;
#19176=FACE_OUTER_BOUND ( 'NONE', #28779, .T. ) ;
#19177=DIRECTION ( 'NONE',  ( 0.2756373558169974980, -0.9612616959383193382, 8.979771562518858393E-33 ) ) ;
#19179=AXIS2_PLACEMENT_3D ( 'NONE', #22869, #2844, #30267 ) ;
#19180=ORIENTED_EDGE ( 'NONE', *, *, #3576, .T. ) ;
#19189=DIRECTION ( 'NONE',  ( 0.2756373558169961102, -0.9612616959383197823, 0.000000000000000000 ) ) ;
#19190=LINE ( 'NONE', #14292, #31591 ) ;
#19191=LINE ( 'NONE', #29219, #4743 ) ;
#19194=ORIENTED_EDGE ( 'NONE', *, *, #30953, .T. ) ;
#19204=CARTESIAN_POINT ( 'NONE',  ( -40.82286654448606811, 10.16735592115171549, 37.04930799450052348 ) ) ;
#19208=EDGE_CURVE ( 'NONE', #3764, #29013, #7842, .T. ) ;
#19209=ADVANCED_FACE ( 'NONE', ( #4635 ), #24490, .F. ) ;
#19214=DIRECTION ( 'NONE',  ( -0.9612616959383221138, -0.2756373558169876170, 0.000000000000000000 ) ) ;
#19217=DIRECTION ( 'NONE',  ( 0.4848096202463430537, 0.8746197071393926326, 1.323854077651070671E-16 ) ) ;
#19218=CARTESIAN_POINT ( 'NONE',  ( -43.64073206722599707, 1.267352857069778960, 34.64930799450052490 ) ) ;
#19224=DIRECTION ( 'NONE',  ( -0.9612616959383200044, -0.2756373558169954996, 1.660411357259285896E-16 ) ) ;
#19229=CARTESIAN_POINT ( 'NONE',  ( -42.38474149870877028, 15.25146566812707505, 35.54930799450051637 ) ) ;
#19231=CIRCLE ( 'NONE', #6148, 1.500000000000001332 ) ;
#19235=AXIS2_PLACEMENT_3D ( 'NONE', #31311, #31635, #23913 ) ;
#19242=FACE_OUTER_BOUND ( 'NONE', #12228, .T. ) ;
#19243=AXIS2_PLACEMENT_3D ( 'NONE', #2981, #209, #10228 ) ;
#19251=EDGE_CURVE ( 'NONE', #22420, #22576, #1871, .T. ) ;
#19256=CARTESIAN_POINT ( 'NONE',  ( -38.36853489569023168, 7.065850718397949315, 32.14930799450051779 ) ) ;
#19262=CARTESIAN_POINT ( 'NONE',  ( -40.69571722278732295, 6.786566810383045656, 34.64930799450051779 ) ) ;
#19266=FACE_OUTER_BOUND ( 'NONE', #28065, .T. ) ;
#19271=CARTESIAN_POINT ( 'NONE',  ( -40.58094809379417001, 7.465224162809761310, 53.91088180535781760 ) ) ;
#19276=CARTESIAN_POINT ( 'NONE',  ( -42.36153388572594736, 13.68895619636815653, 54.64930799450051779 ) ) ;
#19278=CARTESIAN_POINT ( 'NONE',  ( -40.01196617104008624, 7.363926680071349651, 35.23477324418088585 ) ) ;
#19279=CARTESIAN_POINT ( 'NONE',  ( -40.50146157965988891, 7.595301493077381672, 35.64930799450052490 ) ) ;
#19300=DIRECTION ( 'NONE',  ( -1.188208965918165239E-16, -1.880121038077812885E-16, -1.000000000000000000 ) ) ;
#19302=CARTESIAN_POINT ( 'NONE',  ( -40.28779227465695101, 2.984619150196775372, 39.04930799450052348 ) ) ;
#19303=CARTESIAN_POINT ( 'NONE',  ( -40.50726676055796105, 7.559560307024984382, 53.81156708294278701 ) ) ;
#19307=EDGE_LOOP ( 'NONE', ( #3678, #29155, #28999, #13293 ) ) ;
#19309=CIRCLE ( 'NONE', #26684, 0.1000000000000020595 ) ;
#19310=ORIENTED_EDGE ( 'NONE', *, *, #29461, .F. ) ;
#19312=DIRECTION ( 'NONE',  ( -0.9612616959383206705, -0.2756373558169931681, 1.660411357259282445E-16 ) ) ;
#19313=CIRCLE ( 'NONE', #25635, 1.524998423334080533 ) ;
#19316=DIRECTION ( 'NONE',  ( 0.8746197071393926326, -0.4848096202463430537, -8.676864087101709653E-18 ) ) ;
#19317=CONICAL_SURFACE ( 'NONE', #28750, 0.9031915329475502796, 0.7853981633974456145 ) ;
#19322=EDGE_LOOP ( 'NONE', ( #14756, #21789 ) ) ;
#19325=DIRECTION ( 'NONE',  ( -7.588956326749211550E-18, 4.206627182996912454E-18, -1.000000000000000000 ) ) ;
#19332=CARTESIAN_POINT ( 'NONE',  ( -40.73728033978215990, 8.177846351970792682, 59.56562166518216372 ) ) ;
#19334=EDGE_CURVE ( 'NONE', #7595, #5139, #4500, .T. ) ;
#19349=CARTESIAN_POINT ( 'NONE',  ( -41.52218637998914375, 11.15499190493234671, 38.09144330556765112 ) ) ;
#19358=EDGE_LOOP ( 'NONE', ( #15845, #5947, #7877, #25060, #22651, #10332 ) ) ;
#19360=ADVANCED_FACE ( 'NONE', ( #10064 ), #357, .T. ) ;
#19362=CARTESIAN_POINT ( 'NONE',  ( -39.59300248568538194, 7.744584186742829779, 32.04930799450052348 ) ) ;
#19367=CARTESIAN_POINT ( 'NONE',  ( -40.11967773290336226, 9.763195579837789850, 35.54930799450052348 ) ) ;
#19368=ORIENTED_EDGE ( 'NONE', *, *, #5163, .F. ) ;
#19382=CARTESIAN_POINT ( 'NONE',  ( -38.96025635604170390, 15.13029464144910108, 54.64930799450051779 ) ) ;
#19383=DIRECTION ( 'NONE',  ( -0.9612616959383205595, -0.2756373558169931681, 1.660411357259282445E-16 ) ) ;
#19386=ORIENTED_EDGE ( 'NONE', *, *, #28316, .F. ) ;
#19388=DIRECTION ( 'NONE',  ( -0.4848096202463746951, -0.8746197071393748690, 0.000000000000000000 ) ) ;
#19389=CARTESIAN_POINT ( 'NONE',  ( -40.23397449525940317, 6.794506605641760011, 34.64930799450051779 ) ) ;
#19394=CARTESIAN_POINT ( 'NONE',  ( -40.51045226066063520, 7.589116544599141534, 60.22001867261916885 ) ) ;
#19410=CARTESIAN_POINT ( 'NONE',  ( -41.47915246182644466, 10.76506190587095801, 57.22447320499356493 ) ) ;
#19417=ORIENTED_EDGE ( 'NONE', *, *, #21063, .T. ) ;
#19419=VERTEX_POINT ( 'NONE', #27456 ) ;
#19421=AXIS2_PLACEMENT_3D ( 'NONE', #30972, #14049, #24046 ) ;
#19423=CIRCLE ( 'NONE', #22017, 0.2000000000000012601 ) ;
#19425=DIRECTION ( 'NONE',  ( -2.779292025043186357E-18, 1.288349127009862057E-17, -1.000000000000000000 ) ) ;
#19428=ADVANCED_FACE ( 'NONE', ( #20060 ), #15142, .T. ) ;
#19429=CARTESIAN_POINT ( 'NONE',  ( -42.26253548098706858, 13.64258395852576911, 59.54930799450052348 ) ) ;
#19440=ORIENTED_EDGE ( 'NONE', *, *, #8220, .F. ) ;
#19443=DIRECTION ( 'NONE',  ( 0.8746197071393840838, -0.4848096202463581528, 0.000000000000000000 ) ) ;
#19445=ADVANCED_FACE ( 'NONE', ( #31050 ), #25947, .T. ) ;
#19450=VERTEX_POINT ( 'NONE', #688 ) ;
#19452=CARTESIAN_POINT ( 'NONE',  ( -40.12089184044746304, 6.795442064577187580, 34.64508164218045039 ) ) ;
#19459=ORIENTED_EDGE ( 'NONE', *, *, #28235, .T. ) ;
#19461=EDGE_CURVE ( 'NONE', #23152, #229, #20764, .T. ) ;
#19465=EDGE_CURVE ( 'NONE', #20784, #2889, #25474, .T. ) ;
#19467=DIRECTION ( 'NONE',  ( 2.779292025043186357E-18, -1.288349127009862211E-17, 1.000000000000000000 ) ) ;
#19474=DIRECTION ( 'NONE',  ( -0.8746197071393926326, 0.4848096202463430537, 8.676864087101709653E-18 ) ) ;
#19476=EDGE_LOOP ( 'NONE', ( #24839, #28260, #28644, #23689 ) ) ;
#19481=EDGE_CURVE ( 'NONE', #4922, #155, #2976, .T. ) ;
#19483=CARTESIAN_POINT ( 'NONE',  ( -42.50976151518962354, 14.59907569580870224, 36.00717268343339583 ) ) ;
#19484=CYLINDRICAL_SURFACE ( 'NONE', #29938, 0.1000000000000006301 ) ;
#19488=EDGE_CURVE ( 'NONE', #17225, #2185, #31265, .T. ) ;
#19493=DIRECTION ( 'NONE',  ( 0.4848096202463424431, 0.8746197071393928546, -2.220446049250313081E-16 ) ) ;
#19495=DIRECTION ( 'NONE',  ( -0.2756373558169932236, 0.9612616959383205595, 1.994417650674054674E-31 ) ) ;
#19496=DIRECTION ( 'NONE',  ( -0.9612616959383194493, -0.2756373558169972759, -8.795445018804907668E-19 ) ) ;
#19499=TOROIDAL_SURFACE ( 'NONE', #22640, 1.100000000000000089, 0.1000000000000000056 ) ;
#19500=ORIENTED_EDGE ( 'NONE', *, *, #8413, .F. ) ;
#19505=ORIENTED_EDGE ( 'NONE', *, *, #25528, .T. ) ;
#19508=FACE_OUTER_BOUND ( 'NONE', #13282, .T. ) ;
#19512=TOROIDAL_SURFACE ( 'NONE', #6945, 1.299999999999999822, 0.1000000000000000056 ) ;
#19513=DIRECTION ( 'NONE',  ( 0.000000000000000000, 0.000000000000000000, -1.000000000000000000 ) ) ;
#19518=ADVANCED_FACE ( 'NONE', ( #15787 ), #30889, .T. ) ;
#19520=CARTESIAN_POINT ( 'NONE',  ( -38.36853489569023168, 7.065850718397948427, 62.04930799450052348 ) ) ;
#19523=EDGE_CURVE ( 'NONE', #5852, #5096, #13176, .T. ) ;
#19529=DIRECTION ( 'NONE',  ( 0.8746197071393858602, -0.4848096202463547666, 0.000000000000000000 ) ) ;
#19537=CARTESIAN_POINT ( 'NONE',  ( -40.65487266620045403, 9.475231293617262907, 34.66144002885648945 ) ) ;
#19541=ORIENTED_EDGE ( 'NONE', *, *, #4705, .T. ) ;
#19547=VECTOR ( 'NONE', #10637, 1000.000000000000000 ) ;
#19551=DIRECTION ( 'NONE',  ( -0.8746197071393810862, 0.4848096202463637039, 8.676864087101942305E-18 ) ) ;
#19558=DIRECTION ( 'NONE',  ( -0.9612616959383204485, -0.2756373558169933347, 1.660411357259282692E-16 ) ) ;
#19564=CARTESIAN_POINT ( 'NONE',  ( -40.46271621608484281, 3.081581074246048768, 35.54930799450051637 ) ) ;
#19565=EDGE_CURVE ( 'NONE', #18541, #9695, #7674, .T. ) ;
#19567=ORIENTED_EDGE ( 'NONE', *, *, #1968, .F. ) ;
#19568=DIRECTION ( 'NONE',  ( -0.9612616959383206705, -0.2756373558169931681, 1.660411357259282445E-16 ) ) ;
#19571=DIRECTION ( 'NONE',  ( -0.4848096202463432203, -0.8746197071393924105, -9.920727850371698576E-18 ) ) ;
#19573=DIRECTION ( 'NONE',  ( 0.2756373558169956106, -0.9612616959383200044, -1.546443900056102631E-15 ) ) ;
#19576=EDGE_LOOP ( 'NONE', ( #6995, #9454, #27384, #24053 ) ) ;
#19578=CARTESIAN_POINT ( 'NONE',  ( -40.15611298324447631, 6.923081382651431248, 39.54802830809165215 ) ) ;
#19583=DIRECTION ( 'NONE',  ( 0.4848096202463673676, 0.8746197071393789768, 0.000000000000000000 ) ) ;
#19592=CARTESIAN_POINT ( 'NONE',  ( -40.14060284811700541, 7.788019651925920606, 39.54930799450052348 ) ) ;
#19598=DIRECTION ( 'NONE',  ( 0.000000000000000000, 0.000000000000000000, 1.000000000000000000 ) ) ;
#19603=DIRECTION ( 'NONE',  ( -0.2756373558169974980, 0.9612616959383193382, 1.315048337272770589E-17 ) ) ;
#19604=DIRECTION ( 'NONE',  ( 0.9612616959383221138, 0.2756373558169876170, 0.000000000000000000 ) ) ;
#19605=DIRECTION ( 'NONE',  ( -0.8746197071393895239, 0.4848096202463481053, 0.000000000000000000 ) ) ;
#19613=EDGE_LOOP ( 'NONE', ( #6634, #12817, #4749, #27405 ) ) ;
#19616=EDGE_CURVE ( 'NONE', #2499, #24828, #16044, .T. ) ;
#19622=EDGE_CURVE ( 'NONE', #2789, #20229, #16255, .T. ) ;
#19625=CARTESIAN_POINT ( 'NONE',  ( -40.65487266620045403, 9.475231293617264683, 39.54930799450052348 ) ) ;
#19628=CARTESIAN_POINT ( 'NONE',  ( -40.73091736380679606, 9.483895492497156354, 39.44930799450052916 ) ) ;
#19631=DIRECTION ( 'NONE',  ( 0.2756373558169942228, -0.9612616959383203374, 0.000000000000000000 ) ) ;
#19637=DIRECTION ( 'NONE',  ( 0.9612616959383205595, 0.2756373558169931681, -1.660411357259282445E-16 ) ) ;
#19638=EDGE_LOOP ( 'NONE', ( #31462, #15507, #11599, #13256 ) ) ;
#19647=CARTESIAN_POINT ( 'NONE',  ( -42.30426555199245797, 13.25214768565125034, 59.74914412770269934 ) ) ;
#19650=FACE_OUTER_BOUND ( 'NONE', #23786, .T. ) ;
#19654=AXIS2_PLACEMENT_3D ( 'NONE', #1554, #24824, #8951 ) ;
#19655=AXIS2_PLACEMENT_3D ( 'NONE', #2284, #22297, #22130 ) ;
#19657=ORIENTED_EDGE ( 'NONE', *, *, #25392, .T. ) ;
#19663=EDGE_CURVE ( 'NONE', #30888, #28530, #22320, .T. ) ;
#19681=AXIS2_PLACEMENT_3D ( 'NONE', #21313, #9020, #1461 ) ;
#19684=CARTESIAN_POINT ( 'NONE',  ( -40.68572042366847086, 6.804601513393308210, 34.76387516412972190 ) ) ;
#19700=AXIS2_PLACEMENT_3D ( 'NONE', #32013, #26436, #26924 ) ;
#19705=CIRCLE ( 'NONE', #5570, 0.8928932188134564019 ) ;
#19709=DIRECTION ( 'NONE',  ( 0.2756373558169927240, -0.9612616959383207815, 2.391708153157048402E-17 ) ) ;
#19724=ORIENTED_EDGE ( 'NONE', *, *, #8807, .F. ) ;
#19725=EDGE_LOOP ( 'NONE', ( #10789, #4016, #18423, #26781, #28196, #27432, #8332, #15446, #18914, #29706, #18644, #16460, #11996, #4785, #5067 ) ) ;
#19728=DIRECTION ( 'NONE',  ( 0.9612616959383191162, 0.2756373558169986082, 8.795445018805098335E-19 ) ) ;
#19731=ORIENTED_EDGE ( 'NONE', *, *, #2310, .F. ) ;
#19740=CARTESIAN_POINT ( 'NONE',  ( -41.73034863705382946, 11.48775164340967336, 58.05249952744806308 ) ) ;
#19741=ORIENTED_EDGE ( 'NONE', *, *, #28235, .F. ) ;
#19743=EDGE_CURVE ( 'NONE', #29734, #6626, #18931, .T. ) ;
#19748=DIRECTION ( 'NONE',  ( -0.9612616959383207815, -0.2756373558169926685, -8.795445018804289444E-19 ) ) ;
#19750=CIRCLE ( 'NONE', #11367, 0.09999999999999795164 ) ;
#19751=ORIENTED_EDGE ( 'NONE', *, *, #24105, .T. ) ;
#19753=CARTESIAN_POINT ( 'NONE',  ( -40.18454328187963398, 7.548069831825863218, 53.64930799450051779 ) ) ;
#19756=CARTESIAN_POINT ( 'NONE',  ( -40.86567715954772240, 8.502676639195792418, 34.64880948087299117 ) ) ;
#19759=DIRECTION ( 'NONE',  ( 0.9612616959383205595, 0.2756373558169932236, -1.660411357259282445E-16 ) ) ;
#19761=ORIENTED_EDGE ( 'NONE', *, *, #8134, .F. ) ;
#19763=CARTESIAN_POINT ( 'NONE',  ( -41.52623485060432529, 12.58989991563029598, 57.04930799450051637 ) ) ;
#19765=DIRECTION ( 'NONE',  ( -0.8746197071393805311, 0.4848096202463645921, 8.676864087101954631E-18 ) ) ;
#19775=ADVANCED_FACE ( 'NONE', ( #24956 ), #15266, .F. ) ;
#19777=PLANE ( 'NONE',  #6451 ) ;
#19780=VERTEX_POINT ( 'NONE', #4932 ) ;
#19782=EDGE_CURVE ( 'NONE', #25934, #18639, #7401, .T. ) ;
#19786=AXIS2_PLACEMENT_3D ( 'NONE', #18556, #25952, #28432 ) ;
#19795=CARTESIAN_POINT ( 'NONE',  ( -43.64647580959332629, 1.256990871545142774, 60.44930799450051495 ) ) ;
#19799=ORIENTED_EDGE ( 'NONE', *, *, #9440, .T. ) ;
#19802=ORIENTED_EDGE ( 'NONE', *, *, #10581, .F. ) ;
#19803=CARTESIAN_POINT ( 'NONE',  ( -41.74033427429298371, 15.41509661078533355, 35.64930799450052490 ) ) ;
#19804=CARTESIAN_POINT ( 'NONE',  ( -42.76364231915344050, 15.12166775071174030, 35.64930799450052490 ) ) ;
#19805=CYLINDRICAL_SURFACE ( 'NONE', #30460, 1.000000000000000666 ) ;
#19806=LINE ( 'NONE', #17178, #28837 ) ;
#19810=CARTESIAN_POINT ( 'NONE',  ( -43.72819403793993587, 1.315833819094414769, 39.44930799450052916 ) ) ;
#19817=EDGE_CURVE ( 'NONE', #27962, #21721, #21308, .T. ) ;
#19818=AXIS2_PLACEMENT_3D ( 'NONE', #8978, #4374, #1257 ) ;
#19824=VERTEX_POINT ( 'NONE', #811 ) ;
#19825=CARTESIAN_POINT ( 'NONE',  ( -42.66751614955960292, 15.14923148629343608, 35.64930799450052490 ) ) ;
#19835=CIRCLE ( 'NONE', #5707, 0.09999999999999795164 ) ;
#19841=EDGE_LOOP ( 'NONE', ( #14713, #22397, #9146, #3847 ) ) ;
#19846=CARTESIAN_POINT ( 'NONE',  ( -40.56956524039851075, 6.944624558150292337, 34.94636766356422442 ) ) ;
#19847=PLANE ( 'NONE',  #7032 ) ;
#19852=VERTEX_POINT ( 'NONE', #30535 ) ;
#19857=ADVANCED_FACE ( 'NONE', ( #20336, #967 ), #31013, .T. ) ;
#19858=DIRECTION ( 'NONE',  ( 0.000000000000000000, 1.334402673828310677E-15, 1.000000000000000000 ) ) ;
#19862=CYLINDRICAL_SURFACE ( 'NONE', #19, 0.1000000000000007272 ) ;
#19871=CARTESIAN_POINT ( 'NONE',  ( -42.60588768478345401, 14.57151196022700290, 35.90717268343339441 ) ) ;
#19872=LINE ( 'NONE', #2648, #18167 ) ;
#19874=ORIENTED_EDGE ( 'NONE', *, *, #3298, .T. ) ;
#19876=SPHERICAL_SURFACE ( 'NONE', #2235, 0.1000000000000000056 ) ;
#19883=CARTESIAN_POINT ( 'NONE',  ( -41.02113223168485234, 7.230835263863472306, 39.54930799450052348 ) ) ;
#19888=ORIENTED_EDGE ( 'NONE', *, *, #30138, .F. ) ;
#19899=AXIS2_PLACEMENT_3D ( 'NONE', #974, #10997, #20992 ) ;
#19902=ORIENTED_EDGE ( 'NONE', *, *, #13107, .F. ) ;
#19904=CARTESIAN_POINT ( 'NONE',  ( -40.14921103274695469, 6.917687794149812497, 39.54574681281872017 ) ) ;
#19913=ORIENTED_EDGE ( 'NONE', *, *, #6116, .F. ) ;
#19917=VERTEX_POINT ( 'NONE', #13135 ) ;
#19919=DIRECTION ( 'NONE',  ( -0.9612616959383200044, -0.2756373558169954996, 1.660411357259285896E-16 ) ) ;
#19923=DIRECTION ( 'NONE',  ( -0.2756373558169932236, 0.9612616959383204485, -1.479773560108267395E-16 ) ) ;
#19926=DIRECTION ( 'NONE',  ( 0.000000000000000000, 0.000000000000000000, -1.000000000000000000 ) ) ;
#19931=CARTESIAN_POINT ( 'NONE',  ( -43.64647580959332629, 1.256990871545142774, 53.64930799450051779 ) ) ;
#19940=VERTEX_POINT ( 'NONE', #25437 ) ;
#19942=CIRCLE ( 'NONE', #29980, 1.199999999999999734 ) ;
#19945=EDGE_LOOP ( 'NONE', ( #14295, #6143, #20542, #2788 ) ) ;
#19946=CARTESIAN_POINT ( 'NONE',  ( -37.68353499307994525, 12.01442086639228712, 60.44930799450051495 ) ) ;
#19948=ORIENTED_EDGE ( 'NONE', *, *, #21474, .T. ) ;
#19950=AXIS2_PLACEMENT_3D ( 'NONE', #29568, #7073, #17074 ) ;
#19953=CIRCLE ( 'NONE', #561, 0.1000000000000028644 ) ;
#19954=CARTESIAN_POINT ( 'NONE',  ( -41.56459318755936749, 7.281738416154046156, 53.64930799450051779 ) ) ;
#19955=ORIENTED_EDGE ( 'NONE', *, *, #19782, .T. ) ;
#19969=CIRCLE ( 'NONE', #12113, 1.899999999999999023 ) ;
#19971=FACE_OUTER_BOUND ( 'NONE', #17263, .T. ) ;
#19972=DIRECTION ( 'NONE',  ( -0.9612616959383205595, -0.2756373558169932236, 1.660411357259282445E-16 ) ) ;
#19984=ORIENTED_EDGE ( 'NONE', *, *, #27305, .T. ) ;
#19985=DIRECTION ( 'NONE',  ( 0.9612616959383194493, 0.2756373558169974980, 8.795445018804946186E-19 ) ) ;
#19996=ORIENTED_EDGE ( 'NONE', *, *, #29232, .F. ) ;
#20013=FACE_OUTER_BOUND ( 'NONE', #21177, .T. ) ;
#20016=LINE ( 'NONE', #5087, #6849 ) ;
#20032=ADVANCED_FACE ( 'NONE', ( #1278 ), #31172, .F. ) ;
#20033=ORIENTED_EDGE ( 'NONE', *, *, #15999, .F. ) ;
#20042=EDGE_LOOP ( 'NONE', ( #2590, #30012, #3932, #29550 ) ) ;
#20043=FACE_OUTER_BOUND ( 'NONE', #28270, .T. ) ;
#20048=CARTESIAN_POINT ( 'NONE',  ( -40.02540636251513462, 2.839176264122874382, 35.14930799450051779 ) ) ;
#20049=CARTESIAN_POINT ( 'NONE',  ( -40.02540636251513462, 2.839176264122874382, 38.94930799450052206 ) ) ;
#20050=FACE_OUTER_BOUND ( 'NONE', #12297, .T. ) ;
#20060=FACE_OUTER_BOUND ( 'NONE', #23742, .T. ) ;
#20068=CARTESIAN_POINT ( 'NONE',  ( -40.12057988072736237, 7.355395738388401661, 38.85629451012739111 ) ) ;
#20070=ORIENTED_EDGE ( 'NONE', *, *, #14231, .T. ) ;
#20080=CIRCLE ( 'NONE', #10132, 1.500000000000001332 ) ;
#20084=EDGE_CURVE ( 'NONE', #17431, #24463, #13776, .T. ) ;
#20085=AXIS2_PLACEMENT_3D ( 'NONE', #25911, #13455, #15742 ) ;
#20089=CARTESIAN_POINT ( 'NONE',  ( -40.28779227465695101, 2.984619150196775372, 35.54930799450051637 ) ) ;
#20093=CARTESIAN_POINT ( 'NONE',  ( -43.68921302925062378, 1.179890886355839275, 34.64930799450052490 ) ) ;
#20094=CARTESIAN_POINT ( 'NONE',  ( -40.69569484204229326, 6.786538238944499923, 39.45224069363045061 ) ) ;
#20099=DIRECTION ( 'NONE',  ( 0.000000000000000000, 0.000000000000000000, -1.000000000000000000 ) ) ;
#20102=ORIENTED_EDGE ( 'NONE', *, *, #9617, .F. ) ;
#20104=LINE ( 'NONE', #15030, #9120 ) ;
#20111=VECTOR ( 'NONE', #25005, 1000.000000000000114 ) ;
#20113=EDGE_LOOP ( 'NONE', ( #27564, #20863, #16415 ) ) ;
#20115=ORIENTED_EDGE ( 'NONE', *, *, #15843, .F. ) ;
#20116=EDGE_CURVE ( 'NONE', #5658, #1265, #9001, .T. ) ;
#20121=ORIENTED_EDGE ( 'NONE', *, *, #28985, .T. ) ;
#20132=DIRECTION ( 'NONE',  ( 0.8746197071393928546, -0.4848096202463424986, -1.277302113040826515E-17 ) ) ;
#20140=CARTESIAN_POINT ( 'NONE',  ( -40.01416947921581624, 7.179266651196238413, 35.24167910030048034 ) ) ;
#20147=VECTOR ( 'NONE', #13035, 1000.000000000000227 ) ;
#20148=EDGE_LOOP ( 'NONE', ( #9340, #28153, #21610 ) ) ;
#20161=EDGE_CURVE ( 'NONE', #17431, #29734, #12450, .T. ) ;
#20166=CARTESIAN_POINT ( 'NONE',  ( -40.28779227465695101, 2.984619150196775816, 37.04930799450052348 ) ) ;
#20175=VECTOR ( 'NONE', #6886, 1000.000000000000000 ) ;
#20176=CARTESIAN_POINT ( 'NONE',  ( -39.67555847965937943, 2.645252416024337361, 47.04930799450051637 ) ) ;
#20178=LINE ( 'NONE', #7556, #7896 ) ;
#20182=ORIENTED_EDGE ( 'NONE', *, *, #18158, .F. ) ;
#20183=DIRECTION ( 'NONE',  ( 0.2756373558169990523, -0.9612616959383188942, 1.479773560108257288E-16 ) ) ;
#20186=ORIENTED_EDGE ( 'NONE', *, *, #13601, .T. ) ;
#20188=ORIENTED_EDGE ( 'NONE', *, *, #29046, .T. ) ;
#20190=CARTESIAN_POINT ( 'NONE',  ( -40.50720532202722524, 7.584939507552746818, 59.44930799450051495 ) ) ;
#20192=DIRECTION ( 'NONE',  ( 0.4848096202463430537, 0.8746197071393926326, -1.125439520643636483E-16 ) ) ;
#20200=EDGE_CURVE ( 'NONE', #21395, #11200, #8758, .T. ) ;
#20211=DIRECTION ( 'NONE',  ( 7.588956326749211550E-18, -4.206627182996911684E-18, 1.000000000000000000 ) ) ;
#20213=CARTESIAN_POINT ( 'NONE',  ( -40.59307409811868439, 7.534955591098723815, 60.26126833232958546 ) ) ;
#20214=DIRECTION ( 'NONE',  ( 0.3428121700606640565, 0.6184495258776567805, 0.7071067811865474617 ) ) ;
#20223=DIRECTION ( 'NONE',  ( 2.779292025043186357E-18, -1.288349127009862211E-17, 1.000000000000000000 ) ) ;
#20228=CARTESIAN_POINT ( 'NONE',  ( -43.64647580959332629, 1.256990871545142774, 53.64930799450051779 ) ) ;
#20229=VERTEX_POINT ( 'NONE', #18123 ) ;
#20230=ORIENTED_EDGE ( 'NONE', *, *, #29455, .T. ) ;
#20231=CARTESIAN_POINT ( 'NONE',  ( -38.36853489569023168, 7.065850718397948427, 62.04930799450052348 ) ) ;
#20235=DIRECTION ( 'NONE',  ( 0.000000000000000000, 0.000000000000000000, -1.000000000000000000 ) ) ;
#20236=DIRECTION ( 'NONE',  ( -0.9612616959383221138, -0.2756373558169876170, 1.387778780781420432E-13 ) ) ;
#20249=ADVANCED_FACE ( 'NONE', ( #19650 ), #29196, .T. ) ;
#20261=ORIENTED_EDGE ( 'NONE', *, *, #25532, .T. ) ;
#20268=EDGE_CURVE ( 'NONE', #8613, #16662, #12974, .T. ) ;
#20269=ORIENTED_EDGE ( 'NONE', *, *, #2641, .F. ) ;
#20273=ORIENTED_EDGE ( 'NONE', *, *, #27122, .T. ) ;
#20276=CARTESIAN_POINT ( 'NONE',  ( -39.58809650894544774, 2.596771453999702661, 48.34930799450052064 ) ) ;
#20284=CARTESIAN_POINT ( 'NONE',  ( -41.63422246745999189, 11.51531537899137447, 57.95249952744806166 ) ) ;
#20286=EDGE_LOOP ( 'NONE', ( #13801, #6175, #24360, #19088 ) ) ;
#20289=ORIENTED_EDGE ( 'NONE', *, *, #26689, .T. ) ;
#20296=PLANE ( 'NONE',  #12664 ) ;
#20300=ADVANCED_FACE ( 'NONE', ( #30770 ), #28952, .T. ) ;
#20301=CIRCLE ( 'NONE', #23448, 0.09999999999999815981 ) ;
#20303=ADVANCED_FACE ( 'NONE', ( #16302 ), #3670, .T. ) ;
#20304=ORIENTED_EDGE ( 'NONE', *, *, #29480, .T. ) ;
#20317=CARTESIAN_POINT ( 'NONE',  ( -40.73091736380679606, 9.483895492497156354, 38.64930799450052490 ) ) ;
#20322=VECTOR ( 'NONE', #8055, 1000.000000000000000 ) ;
#20323=EDGE_LOOP ( 'NONE', ( #31483, #14204, #225, #22090, #4055 ) ) ;
#20329=CARTESIAN_POINT ( 'NONE',  ( -38.36853489569023168, 7.065850718397949315, 32.14930799450051779 ) ) ;
#20332=CARTESIAN_POINT ( 'NONE',  ( -36.18493864628602807, 8.798967949527998655, 60.44930799450051495 ) ) ;
#20336=FACE_OUTER_BOUND ( 'NONE', #22716, .T. ) ;
#20339=AXIS2_PLACEMENT_3D ( 'NONE', #14484, #31716, #24478 ) ;
#20340=LINE ( 'NONE', #3098, #15678 ) ;
#20342=ORIENTED_EDGE ( 'NONE', *, *, #13354, .T. ) ;
#20346=VECTOR ( 'NONE', #8104, 1000.000000000000114 ) ;
#20347=AXIS2_PLACEMENT_3D ( 'NONE', #21888, #6804, #31436 ) ;
#20358=FACE_OUTER_BOUND ( 'NONE', #29159, .T. ) ;
#20359=CARTESIAN_POINT ( 'NONE',  ( -40.16174044770769314, 7.468546898574135895, 60.54930799450051637 ) ) ;
#20370=ORIENTED_EDGE ( 'NONE', *, *, #26793, .F. ) ;
#20372=VECTOR ( 'NONE', #9837, 1000.000000000000000 ) ;
#20381=ORIENTED_EDGE ( 'NONE', *, *, #22484, .F. ) ;
#20392=VECTOR ( 'NONE', #29190, 1000.000000000000227 ) ;
#20401=LINE ( 'NONE', #30434, #30828 ) ;
#20402=ADVANCED_FACE ( 'NONE', ( #21060 ), #31412, .T. ) ;
#20404=CIRCLE ( 'NONE', #30916, 0.1000000000000014905 ) ;
#20405=ORIENTED_EDGE ( 'NONE', *, *, #7721, .F. ) ;
#20406=VECTOR ( 'NONE', #8922, 1000.000000000000114 ) ;
#20407=CARTESIAN_POINT ( 'NONE',  ( -40.09211399732166115, 9.667069410243957606, 38.64930799450052490 ) ) ;
#20408=DIRECTION ( 'NONE',  ( 0.6184495258776510074, -0.3428121700606679423, 0.7071067811865505703 ) ) ;
#20414=AXIS2_PLACEMENT_3D ( 'NONE', #5987, #8920, #3674 ) ;
#20418=LINE ( 'NONE', #15182, #12463 ) ;
#20422=DIRECTION ( 'NONE',  ( 0.2756373558169954996, -0.9612616959383200044, 2.463803012461673974E-31 ) ) ;
#20423=ORIENTED_EDGE ( 'NONE', *, *, #2408, .T. ) ;
#20424=DIRECTION ( 'NONE',  ( -0.4848096202463429982, -0.8746197071393925215, -9.920727850371698576E-18 ) ) ;
#20425=EDGE_CURVE ( 'NONE', #6336, #28788, #32346, .T. ) ;
#20428=CYLINDRICAL_SURFACE ( 'NONE', #25660, 0.1000000000000006301 ) ;
#20436=EDGE_CURVE ( 'NONE', #4732, #15249, #16783, .T. ) ;
#20437=AXIS2_PLACEMENT_3D ( 'NONE', #31324, #1123, #21130 ) ;
#20438=CIRCLE ( 'NONE', #14147, 1.899999999999999023 ) ;
#20451=CARTESIAN_POINT ( 'NONE',  ( -40.60722745863126448, 9.415333058485023443, 35.49072935073782986 ) ) ;
#20462=CARTESIAN_POINT ( 'NONE',  ( -43.64073206722599707, 1.267352857069779848, 39.54930799450052348 ) ) ;
#20466=DIRECTION ( 'NONE',  ( 0.8746197071393925215, -0.4848096202463429982, -8.676864087101708112E-18 ) ) ;
#20472=EDGE_LOOP ( 'NONE', ( #18193, #26129, #28963 ) ) ;
#20487=TOROIDAL_SURFACE ( 'NONE', #15788, 1.299999999999999822, 0.1000000000000000056 ) ;
#20495=VERTEX_POINT ( 'NONE', #7603 ) ;
#20497=CARTESIAN_POINT ( 'NONE',  ( -40.48129536610376533, 8.613360132207176889, 39.54930799450052348 ) ) ;
#20500=DIRECTION ( 'NONE',  ( 0.000000000000000000, 0.000000000000000000, -1.000000000000000000 ) ) ;
#20503=CARTESIAN_POINT ( 'NONE',  ( -41.13156850465621517, 9.429949956619452678, 38.44930799450052916 ) ) ;
#20504=CARTESIAN_POINT ( 'NONE',  ( -40.11286833322908052, 2.887657226147511302, 57.04930799450051637 ) ) ;
#20507=CARTESIAN_POINT ( 'NONE',  ( -42.47434154250543514, 4.196643200812633978, 37.04930799450052348 ) ) ;
#20509=LINE ( 'NONE', #6068, #20322 ) ;
#20511=VERTEX_POINT ( 'NONE', #17764 ) ;
#20514=DIRECTION ( 'NONE',  ( -0.2756373558169973870, 0.9612616959383193382, 1.315048337272770435E-17 ) ) ;
#20515=CIRCLE ( 'NONE', #20437, 0.7928932188134575343 ) ;
#20521=ORIENTED_EDGE ( 'NONE', *, *, #15481, .F. ) ;
#20525=EDGE_CURVE ( 'NONE', #28530, #6416, #22849, .T. ) ;
#20526=ORIENTED_EDGE ( 'NONE', *, *, #27389, .T. ) ;
#20529=EDGE_CURVE ( 'NONE', #19824, #5228, #8771, .T. ) ;
#20532=PLANE ( 'NONE',  #26985 ) ;
#20534=DIRECTION ( 'NONE',  ( -0.9612616959383207815, -0.2756373558169926685, -8.795445018804289444E-19 ) ) ;
#20538=CARTESIAN_POINT ( 'NONE',  ( -40.49096175631598271, 7.521145078229855230, 53.94930799450052206 ) ) ;
#20539=DIRECTION ( 'NONE',  ( 2.946248497964555786E-19, 3.001156285468303092E-19, 1.000000000000000000 ) ) ;
#20541=DIRECTION ( 'NONE',  ( 0.2530443915477140204, -0.8824706660164525207, 0.3965022818682459316 ) ) ;
#20542=ORIENTED_EDGE ( 'NONE', *, *, #1777, .F. ) ;
#20543=EDGE_LOOP ( 'NONE', ( #18151, #10124, #31556, #19440 ) ) ;
#20545=CIRCLE ( 'NONE', #12719, 0.09999999999999795164 ) ;
#20547=FACE_OUTER_BOUND ( 'NONE', #2379, .T. ) ;
#20553=EDGE_LOOP ( 'NONE', ( #24152, #18495, #27845, #16007 ) ) ;
#20573=AXIS2_PLACEMENT_3D ( 'NONE', #17345, #2574, #27364 ) ;
#20575=DIRECTION ( 'NONE',  ( 0.3428121700606595046, 0.6184495258776487869, 0.7071067811865566766 ) ) ;
#20582=DIRECTION ( 'NONE',  ( 0.4848096202463424986, 0.8746197071393928546, -2.220446049250312834E-16 ) ) ;
#20584=CARTESIAN_POINT ( 'NONE',  ( -38.41701585771487260, 6.978388747684010518, 62.04930799450052348 ) ) ;
#20585=DIRECTION ( 'NONE',  ( -0.2756373558169973870, 0.9612616959383193382, 1.315048337272770280E-17 ) ) ;
#20586=CARTESIAN_POINT ( 'NONE',  ( -40.50410981870283678, 7.604537000166497585, 38.76008276981544753 ) ) ;
#20592=LINE ( 'NONE', #15348, #3116 ) ;
#20593=PLANE ( 'NONE',  #9392 ) ;
#20609=EDGE_CURVE ( 'NONE', #2889, #16322, #20827, .T. ) ;
#20610=ORIENTED_EDGE ( 'NONE', *, *, #31312, .F. ) ;
#20611=FACE_OUTER_BOUND ( 'NONE', #12717, .T. ) ;
#20634=CARTESIAN_POINT ( 'NONE',  ( -40.68293647075807229, 6.808040729367104582, 34.57337564942579178 ) ) ;
#20639=ORIENTED_EDGE ( 'NONE', *, *, #8407, .F. ) ;
#20641=CARTESIAN_POINT ( 'NONE',  ( -42.26497471389478733, 14.66834543456875117, 55.08207028713757580 ) ) ;
#20643=UNCERTAINTY_MEASURE_WITH_UNIT (LENGTH_MEASURE( 1.000000000000000082E-05 ), #5776, 'distance_accuracy_value', 'NONE');
#20647=CIRCLE ( 'NONE', #14887, 0.09999999999999836797 ) ;
#20650=EDGE_CURVE ( 'NONE', #13584, #2858, #21022, .T. ) ;
#20659=DIRECTION ( 'NONE',  ( -0.8746197071393895239, 0.4848096202463481053, 0.000000000000000000 ) ) ;
#20660=DIRECTION ( 'NONE',  ( -0.9612616959383200044, -0.2756373558169956106, -8.795445018804684260E-19 ) ) ;
#20666=AXIS2_PLACEMENT_3D ( 'NONE', #10783, #20775, #17660 ) ;
#20671=AXIS2_PLACEMENT_3D ( 'NONE', #6756, #16754, #22 ) ;
#20675=CARTESIAN_POINT ( 'NONE',  ( -41.94956971822180947, 3.905757428664828890, 47.04930799450051637 ) ) ;
#20679=ADVANCED_FACE ( 'NONE', ( #11192 ), #11035, .F. ) ;
#20682=ORIENTED_EDGE ( 'NONE', *, *, #25696, .T. ) ;
#20683=FACE_OUTER_BOUND ( 'NONE', #28909, .T. ) ;
#20687=AXIS2_PLACEMENT_3D ( 'NONE', #22656, #7413, #17567 ) ;
#20688=AXIS2_PLACEMENT_3D ( 'NONE', #18499, #28371, #23112 ) ;
#20691=CARTESIAN_POINT ( 'NONE',  ( -39.67555847965937943, 2.645252416024337361, 47.04930799450051637 ) ) ;
#20692=CARTESIAN_POINT ( 'NONE',  ( -39.58809650894544774, 2.596771453999702661, 49.04930799450051637 ) ) ;
#20694=DIRECTION ( 'NONE',  ( -0.2756373558169974980, 0.9612616959383193382, 1.315048337272770589E-17 ) ) ;
#20695=CARTESIAN_POINT ( 'NONE',  ( -41.88090303775678080, 13.82677487427665497, 60.54930799450051637 ) ) ;
#20700=EDGE_CURVE ( 'NONE', #1803, #10259, #8255, .T. ) ;
#20701=CARTESIAN_POINT ( 'NONE',  ( -42.38687957179150345, 4.148162238788004608, 55.84930799450052064 ) ) ;
#20702=SURFACE_SIDE_STYLE ('',( #8714 ) ) ;
#20706=LINE ( 'NONE', #27776, #9870 ) ;
#20711=DIRECTION ( 'NONE',  ( 0.2756373558169926685, -0.9612616959383207815, -1.315048337272770743E-17 ) ) ;
#20718=AXIS2_PLACEMENT_3D ( 'NONE', #32418, #9442, #9603 ) ;
#20726=ORIENTED_EDGE ( 'NONE', *, *, #20425, .T. ) ;
#20728=DIRECTION ( 'NONE',  ( -0.4848096202463645921, -0.8746197071393805311, 0.000000000000000000 ) ) ;
#20731=LINE ( 'NONE', #2077, #27351 ) ;
#20733=ORIENTED_EDGE ( 'NONE', *, *, #437, .T. ) ;
#20734=CARTESIAN_POINT ( 'NONE',  ( -40.61178118339597631, 9.038025460530262123, 56.14611646155296398 ) ) ;
#20736=CARTESIAN_POINT ( 'NONE',  ( -40.20068974435373121, 7.604379238274955100, 60.14930799450051779 ) ) ;
#20737=DIRECTION ( 'NONE',  ( 0.4848096202463645921, 0.8746197071393805311, 0.000000000000000000 ) ) ;
#20740=EDGE_LOOP ( 'NONE', ( #16589, #12947, #10622, #24146 ) ) ;
#20742=CARTESIAN_POINT ( 'NONE',  ( -41.13156850465621517, 9.429949956619452678, 35.64930799450052490 ) ) ;
#20743=CYLINDRICAL_SURFACE ( 'NONE', #962, 1.042135311067126979 ) ;
#20744=CARTESIAN_POINT ( 'NONE',  ( -39.58809650894544774, 2.596771453999702661, 47.04930799450051637 ) ) ;
#20745=AXIS2_PLACEMENT_3D ( 'NONE', #3364, #15680, #18614 ) ;
#20749=FACE_OUTER_BOUND ( 'NONE', #16866, .T. ) ;
#20750=CARTESIAN_POINT ( 'NONE',  ( -40.53913548601165218, 7.333497694771939024, 60.31640775708849844 ) ) ;
#20753=DIRECTION ( 'NONE',  ( -0.6797146636928615981, -0.1949050434465267045, -0.7071067811865529018 ) ) ;
#20757=EDGE_CURVE ( 'NONE', #17347, #9190, #13184, .T. ) ;
#20761=CARTESIAN_POINT ( 'NONE',  ( -40.52669582637187062, 7.652910973922025129, 60.15421819779515289 ) ) ;
#20764=CIRCLE ( 'NONE', #8718, 1.003191532947548925 ) ;
#20765=STYLED_ITEM ( 'NONE', ( #1317 ), #18649 ) ;
#20766=ORIENTED_EDGE ( 'NONE', *, *, #1512, .F. ) ;
#20767=( BOUNDED_CURVE ( )  B_SPLINE_CURVE ( 3, ( #24659, #29751, #15611, #685 ),
 .UNSPECIFIED., .F., .F. ) 
 B_SPLINE_CURVE_WITH_KNOTS ( ( 4, 4 ),
 ( 1.558418845015053044E-14, 1.570796326794891673 ),
 .UNSPECIFIED. ) 
 CURVE ( )  GEOMETRIC_REPRESENTATION_ITEM ( )  RATIONAL_B_SPLINE_CURVE ( ( 1.000000000000000000, 0.8047378541243698225, 0.8047378541243698225, 1.000000000000000000 ) ) 
 REPRESENTATION_ITEM ( '' )  );
#20775=DIRECTION ( 'NONE',  ( 0.8746197071393926326, -0.4848096202463430537, -8.676864087101709653E-18 ) ) ;
#20782=VECTOR ( 'NONE', #1609, 1000.000000000000114 ) ;
#20784=VERTEX_POINT ( 'NONE', #3470 ) ;
#20787=CARTESIAN_POINT ( 'NONE',  ( -39.67555847965937943, 2.645252416024337361, 47.04930799450051637 ) ) ;
#20788=CARTESIAN_POINT ( 'NONE',  ( -40.75848109938849717, 9.580021662090986823, 35.54930799450052348 ) ) ;
#20791=CARTESIAN_POINT ( 'NONE',  ( -43.64073206722599707, 1.267352857069779848, 39.44930799450052916 ) ) ;
#20792=CARTESIAN_POINT ( 'NONE',  ( -40.59768508530252973, 7.003142309053439263, 35.04175310890629902 ) ) ;
#20804=EDGE_LOOP ( 'NONE', ( #27465, #22612, #25659, #15960 ) ) ;
#20806=ORIENTED_EDGE ( 'NONE', *, *, #31627, .T. ) ;
#20810=DIRECTION ( 'NONE',  ( -0.2756373558170044369, 0.9612616959383173398, 1.315048337272769818E-17 ) ) ;
#20815=ORIENTED_EDGE ( 'NONE', *, *, #10044, .T. ) ;
#20821=CARTESIAN_POINT ( 'NONE',  ( -40.02996145527347949, 7.371774464818581230, 60.41996114768177506 ) ) ;
#20822=AXIS2_PLACEMENT_3D ( 'NONE', #18973, #27027, #29499 ) ;
#20826=DIRECTION ( 'NONE',  ( -0.8746197071393925215, 0.4848096202463429982, 8.676864087101709653E-18 ) ) ;
#20827=CIRCLE ( 'NONE', #19243, 0.1000000000000018235 ) ;
#20834=CARTESIAN_POINT ( 'NONE',  ( -40.57832939096746827, 7.446916270396702231, 53.86067862812341644 ) ) ;
#20852=CARTESIAN_POINT ( 'NONE',  ( -40.11286833322907341, 2.887657226147507306, 37.04930799450052348 ) ) ;
#20856=EDGE_CURVE ( 'NONE', #18541, #9841, #8528, .T. ) ;
#20862=EDGE_LOOP ( 'NONE', ( #2478, #13429, #5105, #31277 ) ) ;
#20863=ORIENTED_EDGE ( 'NONE', *, *, #17045, .F. ) ;
#20871=ADVANCED_FACE ( 'NONE', ( #13307 ), #4609, .T. ) ;
#20881=DIRECTION ( 'NONE',  ( 0.9612616959383205595, 0.2756373558169932236, -1.660411357259282445E-16 ) ) ;
#20884=DIRECTION ( 'NONE',  ( -0.6184495258776593340, 0.3428121700606657773, 0.7071067811865443531 ) ) ;
#20886=DIRECTION ( 'NONE',  ( -0.03087013654144218910, 0.1076569600579696390, 0.9937087166876367172 ) ) ;
#20891=CARTESIAN_POINT ( 'NONE',  ( -41.02113223168485234, 7.230835263863472306, 39.54930799450052348 ) ) ;
#20895=DIRECTION ( 'NONE',  ( -0.8746197071393805311, 0.4848096202463645921, 8.676864087101954631E-18 ) ) ;
#20901=CARTESIAN_POINT ( 'NONE',  ( -40.13633318854532916, 6.906174383240056613, 34.55842931802699525 ) ) ;
#20904=ORIENTED_EDGE ( 'NONE', *, *, #32359, .T. ) ;
#20906=DIRECTION ( 'NONE',  ( 0.9612616959383205595, 0.2756373558169932236, -1.660411357259282445E-16 ) ) ;
#20907=CARTESIAN_POINT ( 'NONE',  ( -40.17244512953781310, 6.931285263614340941, 39.54930799450052348 ) ) ;
#20909=DIRECTION ( 'NONE',  ( -2.779292025043186357E-18, 1.288349127009862211E-17, -1.000000000000000000 ) ) ;
#20910=LINE ( 'NONE', #30937, #15191 ) ;
#20912=CARTESIAN_POINT ( 'NONE',  ( -41.13768170161382898, 11.26524684725914227, 38.19144330556764544 ) ) ;
#20918=ORIENTED_EDGE ( 'NONE', *, *, #23858, .T. ) ;
#20922=DIRECTION ( 'NONE',  ( -0.2756373558169932236, 0.9612616959383205595, -2.271050992151962865E-31 ) ) ;
#20924=EDGE_CURVE ( 'NONE', #9190, #5852, #20509, .T. ) ;
#20926=LINE ( 'NONE', #18464, #23471 ) ;
#20931=DIRECTION ( 'NONE',  ( 0.000000000000000000, 0.000000000000000000, -1.000000000000000000 ) ) ;
#20942=FACE_OUTER_BOUND ( 'NONE', #23646, .T. ) ;
#20948=CARTESIAN_POINT ( 'NONE',  ( -40.56019413908506266, 7.186695055018779144, 35.29694535755109541 ) ) ;
#20951=CIRCLE ( 'NONE', #4170, 0.09999999999999886757 ) ;
#20954=ORIENTED_EDGE ( 'NONE', *, *, #21181, .F. ) ;
#20956=CIRCLE ( 'NONE', #9435, 0.1000000000000028644 ) ;
#20965=SPHERICAL_SURFACE ( 'NONE', #978, 0.1000000000000000056 ) ;
#20971=EDGE_CURVE ( 'NONE', #25738, #15396, #29356, .T. ) ;
#20977=ORIENTED_EDGE ( 'NONE', *, *, #14864, .F. ) ;
#20987=AXIS2_PLACEMENT_3D ( 'NONE', #9236, #21201, #26792 ) ;
#20988=CARTESIAN_POINT ( 'NONE',  ( -40.15599670534037102, 7.478908884098767196, 35.39279590939684539 ) ) ;
#20992=DIRECTION ( 'NONE',  ( -0.4848096202463429427, -0.8746197071393925215, 2.352477780477436787E-16 ) ) ;
#20995=VERTEX_POINT ( 'NONE', #28879 ) ;
#20999=ORIENTED_EDGE ( 'NONE', *, *, #17668, .T. ) ;
#21000=DIRECTION ( 'NONE',  ( -0.9612616959383194493, -0.2756373558169974980, -8.795445018804946186E-19 ) ) ;
#21007=LINE ( 'NONE', #23956, #5487 ) ;
#21009=LINE ( 'NONE', #3456, #6036 ) ;
#21013=AXIS2_PLACEMENT_3D ( 'NONE', #27202, #10309, #7843 ) ;
#21017=CARTESIAN_POINT ( 'NONE',  ( -40.05987053574653345, 7.506472619680471858, 35.90717268343339441 ) ) ;
#21022=LINE ( 'NONE', #25798, #3526 ) ;
#21026=CYLINDRICAL_SURFACE ( 'NONE', #28327, 0.1000000000000006301 ) ;
#21028=CIRCLE ( 'NONE', #2694, 0.09999999999999904798 ) ;
#21031=ADVANCED_FACE ( 'NONE', ( #26245 ), #19003, .T. ) ;
#21033=VERTEX_POINT ( 'NONE', #21304 ) ;
#21034=AXIS2_PLACEMENT_3D ( 'NONE', #5014, #2704, #10104 ) ;
#21042=ADVANCED_FACE ( 'NONE', ( #4249 ), #14032, .T. ) ;
#21044=DIRECTION ( 'NONE',  ( -0.8746197071393790878, 0.4848096202463673676, 1.277302113040196197E-17 ) ) ;
#21054=CARTESIAN_POINT ( 'NONE',  ( -40.38311397581032480, 8.599301472032985671, 34.60485935866290674 ) ) ;
#21059=AXIS2_PLACEMENT_3D ( 'NONE', #10109, #25198, #24709 ) ;
#21060=FACE_OUTER_BOUND ( 'NONE', #31646, .T. ) ;
#21063=EDGE_CURVE ( 'NONE', #13529, #25136, #21635, .T. ) ;
#21074=ADVANCED_FACE ( 'NONE', ( #26013 ), #16163, .T. ) ;
#21076=EDGE_CURVE ( 'NONE', #9745, #24444, #11892, .T. ) ;
#21092=DIRECTION ( 'NONE',  ( -0.1651779284337430986, 0.9862637841664557703, 1.316559855253201822E-17 ) ) ;
#21093=CARTESIAN_POINT ( 'NONE',  ( -42.38351229602917414, 14.72295342448899191, 60.54930799450051637 ) ) ;
#21094=ORIENTED_EDGE ( 'NONE', *, *, #9121, .T. ) ;
#21096=CARTESIAN_POINT ( 'NONE',  ( -42.66751614955960292, 15.14923148629343430, 38.44930799450052916 ) ) ;
#21103=CARTESIAN_POINT ( 'NONE',  ( -40.62121046050739892, 6.937850113510459771, 34.96172641100285716 ) ) ;
#21106=ORIENTED_EDGE ( 'NONE', *, *, #4826, .F. ) ;
#21107=CARTESIAN_POINT ( 'NONE',  ( -42.03703168893574116, 3.954238390689463145, 47.04930799450051637 ) ) ;
#21108=CARTESIAN_POINT ( 'NONE',  ( -39.58809650894544774, 2.596771453999702661, 45.84930799450051353 ) ) ;
#21109=ORIENTED_EDGE ( 'NONE', *, *, #15587, .F. ) ;
#21111=ORIENTED_EDGE ( 'NONE', *, *, #23430, .F. ) ;
#21112=EDGE_CURVE ( 'NONE', #30194, #32106, #3693, .T. ) ;
#21117=CARTESIAN_POINT ( 'NONE',  ( -41.30594480120427647, 10.40086789971898895, 36.63067884439899302 ) ) ;
#21120=CIRCLE ( 'NONE', #6992, 0.1000000000000008660 ) ;
#21129=CARTESIAN_POINT ( 'NONE',  ( -40.47677217214096146, 7.509199159542113478, 38.76965595547781618 ) ) ;
#21130=DIRECTION ( 'NONE',  ( -0.2756373558169954996, 0.9612616959383198934, 8.751359879570023769E-15 ) ) ;
#21136=CARTESIAN_POINT ( 'NONE',  ( -40.46271621608484281, 3.081581074246047436, 47.04930799450051637 ) ) ;
#21137=CARTESIAN_POINT ( 'NONE',  ( -42.47434154250544225, 4.196643200812637531, 57.04930799450051637 ) ) ;
#21140=CIRCLE ( 'NONE', #22728, 1.199999999999999734 ) ;
#21146=TOROIDAL_SURFACE ( 'NONE', #27963, 1.142135311067127068, 0.1000000000000000056 ) ;
#21148=ADVANCED_FACE ( 'NONE', ( #20611 ), #1460, .T. ) ;
#21157=VERTEX_POINT ( 'NONE', #28808 ) ;
#21167=CARTESIAN_POINT ( 'NONE',  ( -40.68533706394653393, 6.798065515868073838, 34.62231845625134241 ) ) ;
#21168=ORIENTED_EDGE ( 'NONE', *, *, #9717, .F. ) ;
#21175=CARTESIAN_POINT ( 'NONE',  ( -39.64148344771002286, 7.657122216028891870, 61.94930799450052206 ) ) ;
#21177=EDGE_LOOP ( 'NONE', ( #12886, #25406, #21111 ) ) ;
#21181=EDGE_CURVE ( 'NONE', #30637, #28530, #20926, .T. ) ;
#21183=EDGE_CURVE ( 'NONE', #5658, #3050, #1983, .T. ) ;
#21188=TOROIDAL_SURFACE ( 'NONE', #16487, 1.899999999999999467, 0.1000000000000000056 ) ;
#21189=AXIS2_PLACEMENT_3D ( 'NONE', #7084, #9552, #6920 ) ;
#21193=CYLINDRICAL_SURFACE ( 'NONE', #23774, 0.1000000000000028644 ) ;
#21196=CARTESIAN_POINT ( 'NONE',  ( -40.10456357475989364, 7.631942973856654433, 60.14930799450051779 ) ) ;
#21199=DIRECTION ( 'NONE',  ( 0.6797146636928687036, 0.1949050434465272041, -0.7071067811865459074 ) ) ;
#21201=DIRECTION ( 'NONE',  ( 0.8746197071393926326, -0.4848096202463430537, -8.676864087101709653E-18 ) ) ;
#21203=AXIS2_PLACEMENT_3D ( 'NONE', #12186, #22181, #27444 ) ;
#21209=CIRCLE ( 'NONE', #22282, 0.09999999999999904798 ) ;
#21210=EDGE_CURVE ( 'NONE', #1803, #7874, #5151, .T. ) ;
#21213=CARTESIAN_POINT ( 'NONE',  ( -40.11264481937005399, 6.813248423021981637, 34.63680500816278141 ) ) ;
#21215=DIRECTION ( 'NONE',  ( 0.000000000000000000, 0.000000000000000000, -1.000000000000000000 ) ) ;
#21227=VERTEX_POINT ( 'NONE', #22866 ) ;
#21230=AXIS2_PLACEMENT_3D ( 'NONE', #25419, #3412, #10328 ) ;
#21231=( BOUNDED_SURFACE ( )  B_SPLINE_SURFACE ( 3, 2, ( 
 ( #3817, #31242, #8589 ),
 ( #8902, #5973, #26465 ),
 ( #3334, #6283, #11369 ),
 ( #18904, #5813, #28607 ) ),
 .UNSPECIFIED., .F., .F., .F. ) 
 B_SPLINE_SURFACE_WITH_KNOTS ( ( 4, 4 ),
 ( 3, 3 ),
 ( 1.510941981261796796, 1.570796326794896558 ),
 ( 0.000000000000000000, 1.000000000000000000 ),
 .UNSPECIFIED. ) 
 GEOMETRIC_REPRESENTATION_ITEM ( )  RATIONAL_B_SPLINE_SURFACE ( (
 ( 1.000000000000000000, 0.7219065546282052992, 1.000000000000000000),
 ( 1.000000000000000000, 0.7170297040967862356, 1.000000000000000000),
 ( 1.000000000000000000, 0.7120946502353998619, 1.000000000000000000),
 ( 1.000000000000000000, 0.7071067811865515695, 1.000000000000000000) ) ) 
 REPRESENTATION_ITEM ( '' )  SURFACE ( )  );
#21235=CIRCLE ( 'NONE', #1853, 0.1000000000000032530 ) ;
#21237=DIRECTION ( 'NONE',  ( 0.4848096202463673121, 0.8746197071393789768, 0.000000000000000000 ) ) ;
#21242=VERTEX_POINT ( 'NONE', #7621 ) ;
#21243=DIRECTION ( 'NONE',  ( -7.588956326749211550E-18, 4.206627182996911684E-18, -1.000000000000000000 ) ) ;
#21248=ORIENTED_EDGE ( 'NONE', *, *, #25008, .T. ) ;
#21256=DIRECTION ( 'NONE',  ( 0.9612616959383193382, 0.2756373558169973870, 8.795445018804928853E-19 ) ) ;
#21264=CARTESIAN_POINT ( 'NONE',  ( -40.63900869799031312, 6.896661531572857662, 34.99145992875370581 ) ) ;
#21271=ORIENTED_EDGE ( 'NONE', *, *, #6116, .T. ) ;
#21282=LINE ( 'NONE', #31315, #9729 ) ;
#21286=VERTEX_POINT ( 'NONE', #32404 ) ;
#21289=ORIENTED_EDGE ( 'NONE', *, *, #22096, .F. ) ;
#21292=CYLINDRICAL_SURFACE ( 'NONE', #4204, 0.1000000000000014905 ) ;
#21293=CARTESIAN_POINT ( 'NONE',  ( -41.23380787120766655, 11.23768311167744294, 37.04930799450052348 ) ) ;
#21298=CARTESIAN_POINT ( 'NONE',  ( -42.41019933908752648, 14.71530103803245915, 60.54930799450051637 ) ) ;
#21299=CARTESIAN_POINT ( 'NONE',  ( -40.09211399732166115, 9.667069410243957606, 34.64930799450051779 ) ) ;
#21304=CARTESIAN_POINT ( 'NONE',  ( -43.43257085947613660, 1.024086014757300767, 60.44930799450051495 ) ) ;
#21305=ORIENTED_EDGE ( 'NONE', *, *, #3576, .F. ) ;
#21308=CIRCLE ( 'NONE', #30232, 0.1000000000000018235 ) ;
#21311=VERTEX_POINT ( 'NONE', #10248 ) ;
#21313=CARTESIAN_POINT ( 'NONE',  ( -40.16174044770769314, 7.468546898574136783, 53.64930799450051779 ) ) ;
#21317=DIRECTION ( 'NONE',  ( -1.188208965918165239E-16, -1.880121038077812639E-16, -1.000000000000000000 ) ) ;
#21319=AXIS2_PLACEMENT_3D ( 'NONE', #1365, #25834, #882 ) ;
#21320=ORIENTED_EDGE ( 'NONE', *, *, #21360, .F. ) ;
#21321=CARTESIAN_POINT ( 'NONE',  ( -40.57832940339291383, 7.446916344587776848, 60.54930799450051637 ) ) ;
#21327=CARTESIAN_POINT ( 'NONE',  ( -40.41647043964083252, 8.356895951721261540, 59.54930799450050927 ) ) ;
#21329=ORIENTED_EDGE ( 'NONE', *, *, #28793, .T. ) ;
#21337=CARTESIAN_POINT ( 'NONE',  ( -40.50841487316075273, 7.574651041938937013, 60.23716689141008374 ) ) ;
#21343=AXIS2_PLACEMENT_3D ( 'NONE', #28776, #13528, #10906 ) ;
#21346=FACE_OUTER_BOUND ( 'NONE', #25833, .T. ) ;
#21349=ORIENTED_EDGE ( 'NONE', *, *, #22971, .T. ) ;
#21350=DIRECTION ( 'NONE',  ( -0.2756373558169956106, 0.9612616959383197823, 0.000000000000000000 ) ) ;
#21356=LINE ( 'NONE', #29249, #4738 ) ;
#21360=EDGE_CURVE ( 'NONE', #17357, #3287, #31231, .T. ) ;
#21361=CARTESIAN_POINT ( 'NONE',  ( -40.57832940339291383, 7.446916344587776848, 60.23882281530426042 ) ) ;
#21366=AXIS2_PLACEMENT_3D ( 'NONE', #4046, #14072, #11768 ) ;
#21367=CARTESIAN_POINT ( 'NONE',  ( -40.38222711384413088, 8.611297240477076897, 34.61707255558062002 ) ) ;
#21374=DIRECTION ( 'NONE',  ( -2.779292025043186357E-18, 1.288349127009862211E-17, -1.000000000000000000 ) ) ;
#21376=ORIENTED_EDGE ( 'NONE', *, *, #29026, .T. ) ;
#21377=LINE ( 'NONE', #31417, #27790 ) ;
#21379=DIRECTION ( 'NONE',  ( -0.9612616959383202264, -0.2756373558169947779, 3.659346610729174208E-19 ) ) ;
#21383=CARTESIAN_POINT ( 'NONE',  ( -40.52064652407315748, 7.631814549704944106, 60.17616479600645363 ) ) ;
#21387=ADVANCED_FACE ( 'NONE', ( #5800 ), #28756, .T. ) ;
#21388=AXIS2_PLACEMENT_3D ( 'NONE', #24439, #31831, #17051 ) ;
#21395=VERTEX_POINT ( 'NONE', #1022 ) ;
#21398=ORIENTED_EDGE ( 'NONE', *, *, #8992, .T. ) ;
#21406=CARTESIAN_POINT ( 'NONE',  ( -42.36691375901575185, 13.72999064396537250, 59.48380644099231773 ) ) ;
#21409=FACE_OUTER_BOUND ( 'NONE', #26583, .T. ) ;
#21412=CARTESIAN_POINT ( 'NONE',  ( -42.36691375901575185, 13.72999064396537250, 54.61480954800870791 ) ) ;
#21414=CARTESIAN_POINT ( 'NONE',  ( -40.01477201457416299, 7.207664580858174297, 35.09860252446828355 ) ) ;
#21415=DIRECTION ( 'NONE',  ( -0.8746197071393823075, 0.4848096202463614279, 0.000000000000000000 ) ) ;
#21422=ORIENTED_EDGE ( 'NONE', *, *, #13181, .T. ) ;
#21428=VERTEX_POINT ( 'NONE', #10887 ) ;
#21433=CARTESIAN_POINT ( 'NONE',  ( -41.92347351173192749, 13.84990507184044084, 54.57160570446790615 ) ) ;
#21450=CARTESIAN_POINT ( 'NONE',  ( -40.46704362897429519, 7.411062716778913817, 38.79847704167570299 ) ) ;
#21452=CARTESIAN_POINT ( 'NONE',  ( -39.58809650894544774, 2.596771453999702661, 47.04930799450051637 ) ) ;
#21456=CARTESIAN_POINT ( 'NONE',  ( -40.60251150970604073, 6.748447833883063574, 53.64930799450051779 ) ) ;
#21459=DIRECTION ( 'NONE',  ( 0.000000000000000000, 0.000000000000000000, 1.000000000000000000 ) ) ;
#21460=CYLINDRICAL_SURFACE ( 'NONE', #26209, 0.7928932188134565351 ) ;
#21461=DIRECTION ( 'NONE',  ( 0.1949050434465275650, -0.6797146636928697028, 0.7071067811865449082 ) ) ;
#21464=ADVANCED_FACE ( 'NONE', ( #15957 ), #25965, .F. ) ;
#21468=CIRCLE ( 'NONE', #7330, 0.1000000000000002137 ) ;
#21470=ORIENTED_EDGE ( 'NONE', *, *, #27314, .T. ) ;
#21474=EDGE_CURVE ( 'NONE', #5096, #25136, #26613, .T. ) ;
#21476=EDGE_LOOP ( 'NONE', ( #6199, #7813, #3153, #19799, #28393, #28386, #5798 ) ) ;
#21487=VECTOR ( 'NONE', #19558, 1000.000000000000227 ) ;
#21488=ORIENTED_EDGE ( 'NONE', *, *, #1617, .F. ) ;
#21491=CARTESIAN_POINT ( 'NONE',  ( -43.37834615508418068, 1.121909970995877082, 39.44930799450052916 ) ) ;
#21501=DIRECTION ( 'NONE',  ( 0.1949050434465252057, -0.6797146636928670382, 0.7071067811865481278 ) ) ;
#21503=FACE_OUTER_BOUND ( 'NONE', #19725, .T. ) ;
#21504=B_SPLINE_CURVE_WITH_KNOTS ( 'NONE', 3,
 ( #7113, #29936, #19578, #19904, #6786, #14997, #16788, #29602, #24674, #31898, #2191, #17277, #26810, #29764, #25002, #21871, #26967, #4326, #24336 ),
 .UNSPECIFIED., .F., .F.,
 ( 4, 3, 3, 3, 3, 3, 4 ),
 ( 3.237246860597884355E-16, 2.715504454938324236E-05, 5.405723342089737831E-05, 9.254577804459618708E-05, 0.0001429137362853355627, 0.0001870166610891571849, 0.0001891372738450128029 ),
 .UNSPECIFIED. ) ;
#21508=CARTESIAN_POINT ( 'NONE',  ( -40.65762574042817334, 9.591092754368339968, 38.50788663826321567 ) ) ;
#21510=ADVANCED_FACE ( 'NONE', ( #14150 ), #32034, .T. ) ;
#21511=ORIENTED_EDGE ( 'NONE', *, *, #3073, .F. ) ;
#21512=EDGE_CURVE ( 'NONE', #16648, #15550, #5498, .T. ) ;
#21516=DIRECTION ( 'NONE',  ( -0.2743622330404219545, 0.9568148143496242319, -0.09607692814701952744 ) ) ;
#21519=EDGE_LOOP ( 'NONE', ( #7823, #27119, #6827, #23728 ) ) ;
#21525=CARTESIAN_POINT ( 'NONE',  ( -40.02540636251514172, 2.839176264122877047, 57.04930799450051637 ) ) ;
#21541=ORIENTED_EDGE ( 'NONE', *, *, #626, .T. ) ;
#21542=CARTESIAN_POINT ( 'NONE',  ( -42.38687957179150345, 4.148162238788003719, 57.04930799450051637 ) ) ;
#21546=VECTOR ( 'NONE', #12072, 1000.000000000000000 ) ;
#21555=ADVANCED_FACE ( 'NONE', ( #11515 ), #29735, .T. ) ;
#21558=EDGE_CURVE ( 'NONE', #2431, #21817, #9714, .T. ) ;
#21559=ADVANCED_FACE ( 'NONE', ( #13992, #14479 ), #24471, .F. ) ;
#21564=DIRECTION ( 'NONE',  ( 0.8746197071393925215, -0.4848096202463429982, -8.676864087101708112E-18 ) ) ;
#21568=TOROIDAL_SURFACE ( 'NONE', #31036, 1.299999999999999822, 0.1000000000000000056 ) ;
#21572=LINE ( 'NONE', #26179, #1094 ) ;
#21574=DIRECTION ( 'NONE',  ( 0.000000000000000000, 0.000000000000000000, -1.000000000000000000 ) ) ;
#21577=CARTESIAN_POINT ( 'NONE',  ( -40.58856461370174884, 7.499380836222963254, 53.94930799450052206 ) ) ;
#21585=CARTESIAN_POINT ( 'NONE',  ( -40.16503835899720087, 7.510440877657817538, 35.29832907986742185 ) ) ;
#21589=EDGE_CURVE ( 'NONE', #18870, #2451, #31711, .T. ) ;
#21590=CIRCLE ( 'NONE', #4830, 0.1000000000000018235 ) ;
#21591=DIRECTION ( 'NONE',  ( 0.6797146636928705909, 0.1949050434465292025, -0.7071067811865436870 ) ) ;
#21597=ORIENTED_EDGE ( 'NONE', *, *, #28606, .T. ) ;
#21599=AXIS2_PLACEMENT_3D ( 'NONE', #13106, #32475, #15235 ) ;
#21600=ADVANCED_FACE ( 'NONE', ( #31553 ), #9688, .T. ) ;
#21602=VERTEX_POINT ( 'NONE', #9056 ) ;
#21610=ORIENTED_EDGE ( 'NONE', *, *, #15045, .F. ) ;
#21616=VECTOR ( 'NONE', #18630, 1000.000000000000000 ) ;
#21629=ADVANCED_FACE ( 'NONE', ( #2804 ), #25297, .T. ) ;
#21630=CARTESIAN_POINT ( 'NONE',  ( -40.94655644966159969, 10.23591835516384840, 37.04930799450052348 ) ) ;
#21631=ADVANCED_FACE ( 'NONE', ( #12342 ), #24343, .T. ) ;
#21632=DIRECTION ( 'NONE',  ( -0.4848096202463373916, -0.8746197071393956302, -9.920727850371752502E-18 ) ) ;
#21633=LINE ( 'NONE', #13942, #31945 ) ;
#21635=LINE ( 'NONE', #14268, #25580 ) ;
#21636=VERTEX_POINT ( 'NONE', #2323 ) ;
#21639=ORIENTED_EDGE ( 'NONE', *, *, #22630, .T. ) ;
#21641=AXIS2_PLACEMENT_3D ( 'NONE', #15730, #27890, #23283 ) ;
#21642=EDGE_CURVE ( 'NONE', #16662, #15784, #28007, .T. ) ;
#21651=CARTESIAN_POINT ( 'NONE',  ( -40.21091586930921125, 6.838981405724005036, 34.54930799450052348 ) ) ;
#21654=ORIENTED_EDGE ( 'NONE', *, *, #29417, .F. ) ;
#21658=DIRECTION ( 'NONE',  ( -0.9612616959383194493, -0.2756373558169972759, -8.795445018804905742E-19 ) ) ;
#21659=CARTESIAN_POINT ( 'NONE',  ( -42.79701293673568330, 15.60084045232229677, 37.04930799450052348 ) ) ;
#21666=CARTESIAN_POINT ( 'NONE',  ( -40.02540636251513462, 2.839176264122873050, 37.04930799450052348 ) ) ;
#21668=EDGE_CURVE ( 'NONE', #22420, #23989, #29609, .T. ) ;
#21669=VECTOR ( 'NONE', #13853, 1000.000000000000114 ) ;
#21689=EDGE_CURVE ( 'NONE', #15249, #23287, #12510, .T. ) ;
#21693=LINE ( 'NONE', #2002, #23176 ) ;
#21695=FACE_OUTER_BOUND ( 'NONE', #28857, .T. ) ;
#21700=EDGE_CURVE ( 'NONE', #28686, #19450, #18568, .T. ) ;
#21705=CARTESIAN_POINT ( 'NONE',  ( -38.96025635604169679, 15.13029464144909930, 54.54930799450051637 ) ) ;
#21715=CARTESIAN_POINT ( 'NONE',  ( -38.32955388700093380, 6.929907785659376707, 61.94930799450052206 ) ) ;
#21721=VERTEX_POINT ( 'NONE', #19871 ) ;
#21724=FACE_OUTER_BOUND ( 'NONE', #28599, .T. ) ;
#21730=ORIENTED_EDGE ( 'NONE', *, *, #3631, .T. ) ;
#21732=ORIENTED_EDGE ( 'NONE', *, *, #26893, .F. ) ;
#21735=DIRECTION ( 'NONE',  ( 0.2756373558169932236, -0.9612616959383204485, 1.479773560108267395E-16 ) ) ;
#21737=VERTEX_POINT ( 'NONE', #27754 ) ;
#21748=ORIENTED_EDGE ( 'NONE', *, *, #24799, .T. ) ;
#21756=ORIENTED_EDGE ( 'NONE', *, *, #21512, .T. ) ;
#21757=VECTOR ( 'NONE', #8354, 1000.000000000000000 ) ;
#21758=CIRCLE ( 'NONE', #11815, 2.000000000000001776 ) ;
#21760=AXIS2_PLACEMENT_3D ( 'NONE', #15816, #1188, #13041 ) ;
#21764=ORIENTED_EDGE ( 'NONE', *, *, #20268, .F. ) ;
#21772=VERTEX_POINT ( 'NONE', #13318 ) ;
#21777=CARTESIAN_POINT ( 'NONE',  ( -41.56459318755936749, 7.281738416154046156, 60.44930799450051495 ) ) ;
#21783=EDGE_CURVE ( 'NONE', #26975, #29530, #3371, .T. ) ;
#21786=DIRECTION ( 'NONE',  ( 0.1949050434465282311, -0.6797146636928674823, -0.7071067811865470176 ) ) ;
#21789=ORIENTED_EDGE ( 'NONE', *, *, #13362, .F. ) ;
#21799=ORIENTED_EDGE ( 'NONE', *, *, #17977, .T. ) ;
#21805=ORIENTED_EDGE ( 'NONE', *, *, #20757, .T. ) ;
#21806=CARTESIAN_POINT ( 'NONE',  ( -39.64148344771002286, 7.657122216028890982, 61.94930799450052206 ) ) ;
#21810=EDGE_CURVE ( 'NONE', #24691, #28989, #19123, .T. ) ;
#21813=DIRECTION ( 'NONE',  ( -0.2756373558169954441, 0.9612616959383198934, -1.479773560108263204E-16 ) ) ;
#21817=VERTEX_POINT ( 'NONE', #25770 ) ;
#21821=DIRECTION ( 'NONE',  ( 0.2756373558170082672, -0.9612616959383162296, 3.469446951953592101E-14 ) ) ;
#21828=DIRECTION ( 'NONE',  ( 0.4848096202463429427, 0.8746197071393925215, -2.352477780477436294E-16 ) ) ;
#21830=VERTEX_POINT ( 'NONE', #23788 ) ;
#21839=ADVANCED_FACE ( 'NONE', ( #6235 ), #3606, .F. ) ;
#21842=DIRECTION ( 'NONE',  ( 0.2756373558169974980, -0.9612616959383193382, -1.315048337272770589E-17 ) ) ;
#21843=ADVANCED_FACE ( 'NONE', ( #30867 ), #13791, .T. ) ;
#21847=ADVANCED_FACE ( 'NONE', ( #18058, #28085 ), #5593, .T. ) ;
#21848=ORIENTED_EDGE ( 'NONE', *, *, #19622, .F. ) ;
#21849=ADVANCED_FACE ( 'NONE', ( #20683 ), #26415, .T. ) ;
#21851=CARTESIAN_POINT ( 'NONE',  ( -40.66586793973302605, 8.138261812237590931, 54.59072935073782418 ) ) ;
#21852=PLANE ( 'NONE',  #14729 ) ;
#21853=CARTESIAN_POINT ( 'NONE',  ( -42.50976151518963064, 14.59907569580870224, 38.19144330556764544 ) ) ;
#21860=CARTESIAN_POINT ( 'NONE',  ( -40.58856461370174884, 7.499380836222963254, 53.94930799450052206 ) ) ;
#21871=CARTESIAN_POINT ( 'NONE',  ( -40.11669538345026353, 6.804256812083828265, 39.45088313409969771 ) ) ;
#21878=CIRCLE ( 'NONE', #28173, 0.9031915329475519449 ) ;
#21880=ADVANCED_FACE ( 'NONE', ( #31672, #19176 ), #16398, .T. ) ;
#21883=CARTESIAN_POINT ( 'NONE',  ( -41.89334324224037687, 13.85403361400641487, 54.61507042654626787 ) ) ;
#21886=DIRECTION ( 'NONE',  ( 0.000000000000000000, 0.000000000000000000, -1.000000000000000000 ) ) ;
#21887=CARTESIAN_POINT ( 'NONE',  ( -40.50726676055796105, 7.559560307024983494, 53.64930799450051779 ) ) ;
#21888=CARTESIAN_POINT ( 'NONE',  ( -40.11286833322908052, 2.887657226147511302, 57.04930799450051637 ) ) ;
#21889=AXIS2_PLACEMENT_3D ( 'NONE', #11606, #11922, #29003 ) ;
#21895=DIRECTION ( 'NONE',  ( 0.2756373558169959437, -0.9612616959383197823, 0.000000000000000000 ) ) ;
#21896=CARTESIAN_POINT ( 'NONE',  ( -40.67786913486117584, 6.803913533337310859, 39.48656708792704961 ) ) ;
#21904=CARTESIAN_POINT ( 'NONE',  ( -40.23847960488978970, 6.935107575318146367, 34.63465864742641998 ) ) ;
#21909=ORIENTED_EDGE ( 'NONE', *, *, #13952, .T. ) ;
#21910=DIRECTION ( 'NONE',  ( 0.4848096202462280901, 0.8746197071394562483, 0.000000000000000000 ) ) ;
#21913=EDGE_LOOP ( 'NONE', ( #31818, #17480, #3728, #17502 ) ) ;
#21915=UNCERTAINTY_MEASURE_WITH_UNIT (LENGTH_MEASURE( 1.000000000000000082E-05 ), #18546, 'distance_accuracy_value', 'NONE');
#21919=VECTOR ( 'NONE', #28027, 1000.000000000000114 ) ;
#21934=ORIENTED_EDGE ( 'NONE', *, *, #6183, .F. ) ;
#21936=CARTESIAN_POINT ( 'NONE',  ( -41.10400476907452116, 9.333823787025618657, 35.46646528202590787 ) ) ;
#21938=CARTESIAN_POINT ( 'NONE',  ( -42.28293707589220674, 13.65198258188957148, 54.55385885333606666 ) ) ;
#21941=TOROIDAL_SURFACE ( 'NONE', #24550, 1.899999999999999467, 0.1000000000000000056 ) ;
#21947=CYLINDRICAL_SURFACE ( 'NONE', #26071, 1.042135311067126979 ) ;
#21948=CIRCLE ( 'NONE', #12007, 2.000000000000001776 ) ;
#21950=LINE ( 'NONE', #12290, #20392 ) ;
#21952=EDGE_LOOP ( 'NONE', ( #14370, #10027 ) ) ;
#21956=AXIS2_PLACEMENT_3D ( 'NONE', #29604, #22035, #17446 ) ;
#21977=CARTESIAN_POINT ( 'NONE',  ( -40.71142685946214357, 9.415924026127871826, 39.52001867261917312 ) ) ;
#21981=ORIENTED_EDGE ( 'NONE', *, *, #19663, .F. ) ;
#21986=CARTESIAN_POINT ( 'NONE',  ( -40.68997348041997952, 6.796928795907699161, 60.54930799450051637 ) ) ;
#21989=LINE ( 'NONE', #29725, #11529 ) ;
#21996=CARTESIAN_POINT ( 'NONE',  ( -41.07644103349282005, 9.237697617431789965, 39.44930799450052206 ) ) ;
#21999=CIRCLE ( 'NONE', #20414, 0.2000000000000004274 ) ;
#22006=ORIENTED_EDGE ( 'NONE', *, *, #3889, .T. ) ;
#22012=DIRECTION ( 'NONE',  ( 0.7141240004913222972, -0.3958453973320028019, -0.5773502691896303940 ) ) ;
#22013=CARTESIAN_POINT ( 'NONE',  ( -40.68422973805265030, 6.807290781432339344, 39.44930799450052206 ) ) ;
#22017=AXIS2_PLACEMENT_3D ( 'NONE', #14127, #1644, #21821 ) ;
#22018=EDGE_CURVE ( 'NONE', #2789, #9190, #9182, .T. ) ;
#22019=CARTESIAN_POINT ( 'NONE',  ( -40.15225626691278649, 6.735663658092487793, 53.64930799450051779 ) ) ;
#22024=CARTESIAN_POINT ( 'NONE',  ( -40.39719969963199020, 8.565602912590085438, 34.57497286466457354 ) ) ;
#22025=EDGE_CURVE ( 'NONE', #29567, #20511, #2364, .T. ) ;
#22026=CARTESIAN_POINT ( 'NONE',  ( -40.14921103274695469, 6.917687794149811609, 34.55286917618232678 ) ) ;
#22030=CARTESIAN_POINT ( 'NONE',  ( -40.13663441551143762, 7.212672898651377729, 38.96029010263398362 ) ) ;
#22035=DIRECTION ( 'NONE',  ( -0.9612616959383205595, -0.2756373558169932236, 1.660411357259282445E-16 ) ) ;
#22040=LINE ( 'NONE', #31903, #17461 ) ;
#22042=DIRECTION ( 'NONE',  ( -0.8746197071393790878, 0.4848096202463673676, 1.277302113040196197E-17 ) ) ;
#22043=ORIENTED_EDGE ( 'NONE', *, *, #18031, .T. ) ;
#22046=AXIS2_PLACEMENT_3D ( 'NONE', #14415, #23928, #11458 ) ;
#22050=CARTESIAN_POINT ( 'NONE',  ( -40.16174044770769314, 7.468546898574136783, 59.44930799450051495 ) ) ;
#22052=ORIENTED_EDGE ( 'NONE', *, *, #23858, .F. ) ;
#22053=CARTESIAN_POINT ( 'NONE',  ( -40.02540636251514172, 2.839176264122877047, 57.04930799450051637 ) ) ;
#22060=EDGE_CURVE ( 'NONE', #16834, #11047, #9171, .T. ) ;
#22062=CARTESIAN_POINT ( 'NONE',  ( -40.68455241913549258, 6.798696092114603573, 39.47735115308336162 ) ) ;
#22065=CARTESIAN_POINT ( 'NONE',  ( -40.73091736380679606, 9.483895492497154578, 34.64930799450051779 ) ) ;
#22067=EDGE_CURVE ( 'NONE', #25827, #20229, #27396, .T. ) ;
#22069=CARTESIAN_POINT ( 'NONE',  ( -40.23847960489091236, 6.935107575317837281, 34.54930799450052348 ) ) ;
#22073=CARTESIAN_POINT ( 'NONE',  ( -40.02661603751052155, 7.039661056838986575, 34.81911587904692595 ) ) ;
#22087=EDGE_LOOP ( 'NONE', ( #3899, #2740, #2423, #20977 ) ) ;
#22088=AXIS2_PLACEMENT_3D ( 'NONE', #14504, #22695, #9743 ) ;
#22090=ORIENTED_EDGE ( 'NONE', *, *, #10244, .T. ) ;
#22096=EDGE_CURVE ( 'NONE', #23532, #8765, #23320, .T. ) ;
#22105=CARTESIAN_POINT ( 'NONE',  ( -42.37913764077812573, 15.23192269303853053, 35.54930799450051637 ) ) ;
#22107=CARTESIAN_POINT ( 'NONE',  ( -42.24141723705587737, 13.63285518870473290, 54.54930799450051637 ) ) ;
#22108=LINE ( 'NONE', #25069, #10574 ) ;
#22115=LINE ( 'NONE', #14581, #18753 ) ;
#22119=CARTESIAN_POINT ( 'NONE',  ( -40.65120636623950645, 8.087130829066872195, 57.04930799450051637 ) ) ;
#22120=DIRECTION ( 'NONE',  ( -0.9612616959383194493, -0.2756373558169972759, -8.795445018804905742E-19 ) ) ;
#22125=EDGE_LOOP ( 'NONE', ( #20121, #20726, #28971, #9768 ) ) ;
#22130=DIRECTION ( 'NONE',  ( -0.9612616959383221138, -0.2756373558169876170, 0.000000000000000000 ) ) ;
#22135=AXIS2_PLACEMENT_3D ( 'NONE', #4811, #14833, #2352 ) ;
#22151=CARTESIAN_POINT ( 'NONE',  ( -42.50976151518963064, 14.59907569580870224, 35.90717268343339441 ) ) ;
#22155=CARTESIAN_POINT ( 'NONE',  ( -40.69343167531472005, 8.234387981831414294, 59.54930799450052348 ) ) ;
#22156=ADVANCED_FACE ( 'NONE', ( #28678 ), #16195, .T. ) ;
#22158=ADVANCED_FACE ( 'NONE', ( #18338 ), #28201, .T. ) ;
#22162=EDGE_CURVE ( 'NONE', #16662, #27962, #13377, .T. ) ;
#22164=ORIENTED_EDGE ( 'NONE', *, *, #407, .T. ) ;
#22171=CARTESIAN_POINT ( 'NONE',  ( -40.06561427811386267, 7.496110634155836117, 60.54930799450051637 ) ) ;
#22181=DIRECTION ( 'NONE',  ( -0.4848096202463430537, -0.8746197071393926326, -9.920727850371701658E-18 ) ) ;
#22212=AXIS2_PLACEMENT_3D ( 'NONE', #28991, #27165, #1409 ) ;
#22213=CARTESIAN_POINT ( 'NONE',  ( -38.22549819199227272, 15.91524478274158483, 59.54930799450050927 ) ) ;
#22215=PLANE ( 'NONE',  #19179 ) ;
#22217=EDGE_CURVE ( 'NONE', #9700, #30206, #15723, .T. ) ;
#22220=CARTESIAN_POINT ( 'NONE',  ( -40.81568357405034675, 8.445604592586153814, 34.57497286466457354 ) ) ;
#22222=CARTESIAN_POINT ( 'NONE',  ( -41.88090303775678080, 13.82677487427665497, 59.44930799450051495 ) ) ;
#22223=AXIS2_PLACEMENT_3D ( 'NONE', #16760, #19217, #31393 ) ;
#22227=DIRECTION ( 'NONE',  ( -0.8746197071393790878, 0.4848096202463673676, 1.277302113040196197E-17 ) ) ;
#22236=CARTESIAN_POINT ( 'NONE',  ( -36.76418579970419387, 10.14130568307076352, 57.04930799450051637 ) ) ;
#22239=CARTESIAN_POINT ( 'NONE',  ( -40.18454328187963398, 7.548069831825862330, 60.44930799450051495 ) ) ;
#22243=ORIENTED_EDGE ( 'NONE', *, *, #28793, .F. ) ;
#22244=AXIS2_PLACEMENT_3D ( 'NONE', #27597, #2488, #17088 ) ;
#22246=ADVANCED_FACE ( 'NONE', ( #26373 ), #1906, .F. ) ;
#22253=ADVANCED_FACE ( 'NONE', ( #29319 ), #4216, .T. ) ;
#22255=ORIENTED_EDGE ( 'NONE', *, *, #1932, .F. ) ;
#22257=ADVANCED_FACE ( 'NONE', ( #3730 ), #6842, .F. ) ;
#22260=CARTESIAN_POINT ( 'NONE',  ( -42.54104507194909957, 14.67778162788815344, 59.54930799450050927 ) ) ;
#22266=CARTESIAN_POINT ( 'NONE',  ( -41.10316901461906980, 9.481183992871798694, 35.54930799450051637 ) ) ;
#22267=VERTEX_POINT ( 'NONE', #24393 ) ;
#22276=DIRECTION ( 'NONE',  ( -0.2756373558169973870, 0.9612616959383193382, 1.315048337272770280E-17 ) ) ;
#22277=VECTOR ( 'NONE', #8392, 1000.000000000000000 ) ;
#22278=EDGE_LOOP ( 'NONE', ( #30524, #2731, #27478, #26180 ) ) ;
#22279=ADVANCED_FACE ( 'NONE', ( #23910 ), #29162, .F. ) ;
#22282=AXIS2_PLACEMENT_3D ( 'NONE', #13255, #6014, #10788 ) ;
#22287=CARTESIAN_POINT ( 'NONE',  ( -39.85048242108726413, 2.742214340073605872, 47.04930799450051637 ) ) ;
#22288=VERTEX_POINT ( 'NONE', #14237 ) ;
#22289=ORIENTED_EDGE ( 'NONE', *, *, #5190, .T. ) ;
#22291=EDGE_LOOP ( 'NONE', ( #15407, #25093, #10868, #24022 ) ) ;
#22297=DIRECTION ( 'NONE',  ( 0.2756373558169976645, -0.9612616959383194493, 1.479773560108259753E-16 ) ) ;
#22298=CARTESIAN_POINT ( 'NONE',  ( -40.50720532202722524, 7.584939507552746818, 54.01510846932454513 ) ) ;
#22303=ADVANCED_FACE ( 'NONE', ( #26536 ), #9138, .F. ) ;
#22304=FACE_OUTER_BOUND ( 'NONE', #28825, .T. ) ;
#22312=CIRCLE ( 'NONE', #6596, 1.000000000000000666 ) ;
#22320=LINE ( 'NONE', #2627, #29668 ) ;
#22333=ORIENTED_EDGE ( 'NONE', *, *, #6772, .F. ) ;
#22335=DIRECTION ( 'NONE',  ( 0.000000000000000000, 1.000000000000000000, 0.000000000000000000 ) ) ;
#22337=EDGE_CURVE ( 'NONE', #18639, #7358, #1298, .T. ) ;
#22338=VERTEX_POINT ( 'NONE', #6516 ) ;
#22339=CYLINDRICAL_SURFACE ( 'NONE', #22244, 1.500000000000001332 ) ;
#22345=CARTESIAN_POINT ( 'NONE',  ( -40.50146157965988891, 7.595301493077381672, 34.64930799450051779 ) ) ;
#22347=CARTESIAN_POINT ( 'NONE',  ( -41.57366591477001805, 14.83385496645368384, 37.04930799450052348 ) ) ;
#22352=ORIENTED_EDGE ( 'NONE', *, *, #10445, .F. ) ;
#22353=CARTESIAN_POINT ( 'NONE',  ( -40.02540636251514172, 2.839176264122877047, 57.04930799450051637 ) ) ;
#22360=CARTESIAN_POINT ( 'NONE',  ( -40.18454328187963398, 7.548069831825863218, 60.54930799450051637 ) ) ;
#22361=CARTESIAN_POINT ( 'NONE',  ( -40.99980536824363497, 9.333232819382775602, 39.52001867261917312 ) ) ;
#22363=EDGE_LOOP ( 'NONE', ( #10323, #4005, #20115, #31217 ) ) ;
#22364=DIRECTION ( 'NONE',  ( 0.9612616959383205595, 0.2756373558169932236, -1.660411357259282445E-16 ) ) ;
#22370=ORIENTED_EDGE ( 'NONE', *, *, #27314, .F. ) ;
#22373=EDGE_CURVE ( 'NONE', #26808, #6349, #3558, .T. ) ;
#22377=CARTESIAN_POINT ( 'NONE',  ( -41.23380787120766655, 11.23768311167744294, 37.04930799450052348 ) ) ;
#22383=LINE ( 'NONE', #14694, #29885 ) ;
#22384=DIRECTION ( 'NONE',  ( -1.188208965918165239E-16, -1.880121038077813132E-16, -1.000000000000000000 ) ) ;
#22397=ORIENTED_EDGE ( 'NONE', *, *, #3404, .T. ) ;
#22398=DIRECTION ( 'NONE',  ( 0.4848096202463430537, 0.8746197071393926326, 1.323854077651070671E-16 ) ) ;
#22399=DIRECTION ( 'NONE',  ( -0.4848096202463429427, -0.8746197071393925215, 2.352477780477436294E-16 ) ) ;
#22401=DIRECTION ( 'NONE',  ( -0.8746197071393926326, 0.4848096202463430537, 8.676864087101709653E-18 ) ) ;
#22403=EDGE_CURVE ( 'NONE', #5569, #10175, #7244, .T. ) ;
#22416=CARTESIAN_POINT ( 'NONE',  ( -40.15225626691278649, 6.735663658092487793, 60.44930799450051495 ) ) ;
#22420=VERTEX_POINT ( 'NONE', #20276 ) ;
#22422=DIRECTION ( 'NONE',  ( 0.7141240004913198547, -0.3958453973320100738, -0.5773502691896283956 ) ) ;
#22423=ORIENTED_EDGE ( 'NONE', *, *, #2641, .T. ) ;
#22427=CARTESIAN_POINT ( 'NONE',  ( -41.08785830660042393, 9.277514380576532105, 39.40788663826320715 ) ) ;
#22429=FACE_OUTER_BOUND ( 'NONE', #2572, .T. ) ;
#22431=EDGE_CURVE ( 'NONE', #21772, #10919, #22580, .T. ) ;
#22433=DIRECTION ( 'NONE',  ( 0.9577728606650218746, 0.2746369484007246675, 0.08512164205816423468 ) ) ;
#22437=CIRCLE ( 'NONE', #20347, 2.000000000000001776 ) ;
#22440=AXIS2_PLACEMENT_3D ( 'NONE', #26314, #11221, #28944 ) ;
#22442=VERTEX_POINT ( 'NONE', #27177 ) ;
#22446=CIRCLE ( 'NONE', #10931, 0.1000000000000006301 ) ;
#22448=ORIENTED_EDGE ( 'NONE', *, *, #21112, .T. ) ;
#22451=CARTESIAN_POINT ( 'NONE',  ( -40.30085376570235667, 8.316488220933674569, 54.52001867261917312 ) ) ;
#22454=VECTOR ( 'NONE', #8875, 1000.000000000000227 ) ;
#22461=ORIENTED_EDGE ( 'NONE', *, *, #13434, .F. ) ;
#22462=DIRECTION ( 'NONE',  ( 0.8746197071393925215, -0.4848096202463429982, -8.676864087101708112E-18 ) ) ;
#22465=CARTESIAN_POINT ( 'NONE',  ( -41.00315188238673159, 10.79608561255925991, 36.12712545380572493 ) ) ;
#22472=ORIENTED_EDGE ( 'NONE', *, *, #6752, .F. ) ;
#22477=CARTESIAN_POINT ( 'NONE',  ( -40.16503835899720087, 7.510440877657823755, 38.80028690913362510 ) ) ;
#22484=EDGE_CURVE ( 'NONE', #19450, #28686, #22949, .T. ) ;
#22485=PLANE ( 'NONE',  #2361 ) ;
#22487=( BOUNDED_CURVE ( )  B_SPLINE_CURVE ( 3, ( #10738, #31236, #13836, #6277 ),
 .UNSPECIFIED., .F., .F. ) 
 B_SPLINE_CURVE_WITH_KNOTS ( ( 4, 4 ),
 ( 3.141592653589791784, 4.712388980384687898 ),
 .UNSPECIFIED. ) 
 CURVE ( )  GEOMETRIC_REPRESENTATION_ITEM ( )  RATIONAL_B_SPLINE_CURVE ( ( 1.000000000000000000, 0.8047378541243650485, 0.8047378541243650485, 1.000000000000000000 ) ) 
 REPRESENTATION_ITEM ( '' )  );
#22505=DIRECTION ( 'NONE',  ( 0.2756373558169932236, -0.9612616959383205595, 1.479773560108267395E-16 ) ) ;
#22508=FACE_OUTER_BOUND ( 'NONE', #20113, .T. ) ;
#22509=EDGE_CURVE ( 'NONE', #14586, #10311, #2371, .T. ) ;
#22514=CARTESIAN_POINT ( 'NONE',  ( -40.70335362822509495, 9.387769322903325886, 39.54930799450052348 ) ) ;
#22521=AXIS2_PLACEMENT_3D ( 'NONE', #22775, #9992, #25251 ) ;
#22533=SPHERICAL_SURFACE ( 'NONE', #28763, 0.1000000000000000056 ) ;
#22548=DIRECTION ( 'NONE',  ( 0.8746197071393926326, -0.4848096202463430537, -8.676864087101709653E-18 ) ) ;
#22557=ORIENTED_EDGE ( 'NONE', *, *, #26533, .T. ) ;
#22560=ORIENTED_EDGE ( 'NONE', *, *, #27106, .T. ) ;
#22564=DIRECTION ( 'NONE',  ( 0.8746197071393926326, -0.4848096202463430537, -8.676864087101709653E-18 ) ) ;
#22576=VERTEX_POINT ( 'NONE', #5365 ) ;
#22577=AXIS2_PLACEMENT_3D ( 'NONE', #12278, #17516, #12606 ) ;
#22578=EDGE_CURVE ( 'NONE', #23798, #24691, #22906, .T. ) ;
#22579=DIRECTION ( 'NONE',  ( 0.8746197071393926326, -0.4848096202463430537, -8.676864087101709653E-18 ) ) ;
#22580=LINE ( 'NONE', #19625, #11429 ) ;
#22585=VECTOR ( 'NONE', #964, 999.9999999999998863 ) ;
#22589=VECTOR ( 'NONE', #5168, 1000.000000000000000 ) ;
#22591=VERTEX_POINT ( 'NONE', #23069 ) ;
#22593=ORIENTED_EDGE ( 'NONE', *, *, #24603, .F. ) ;
#22599=CARTESIAN_POINT ( 'NONE',  ( -41.04685960816998147, 9.497330455345890599, 38.54930799450052348 ) ) ;
#22604=FACE_OUTER_BOUND ( 'NONE', #3183, .T. ) ;
#22605=CARTESIAN_POINT ( 'NONE',  ( -40.14651252454546437, 6.746025643617124423, 34.64930799450052490 ) ) ;
#22609=ORIENTED_EDGE ( 'NONE', *, *, #589, .T. ) ;
#22611=DIRECTION ( 'NONE',  ( 0.2756373558169954441, -0.9612616959383198934, 1.479773560108263451E-16 ) ) ;
#22612=ORIENTED_EDGE ( 'NONE', *, *, #15012, .F. ) ;
#22627=CARTESIAN_POINT ( 'NONE',  ( -39.64148344771002286, 7.657122216028891870, 32.14930799450051779 ) ) ;
#22630=EDGE_CURVE ( 'NONE', #18307, #22267, #22437, .T. ) ;
#22634=EDGE_CURVE ( 'NONE', #9470, #26626, #9104, .T. ) ;
#22636=CARTESIAN_POINT ( 'NONE',  ( -40.62017490690357846, 6.854514378931023444, 34.77675100468818670 ) ) ;
#22640=AXIS2_PLACEMENT_3D ( 'NONE', #23698, #24011, #29110 ) ;
#22651=ORIENTED_EDGE ( 'NONE', *, *, #12398, .F. ) ;
#22654=EDGE_CURVE ( 'NONE', #20495, #9745, #8622, .T. ) ;
#22656=CARTESIAN_POINT ( 'NONE',  ( -41.09081837022679906, 10.70862666502100069, 57.17865484131924347 ) ) ;
#22660=CIRCLE ( 'NONE', #12177, 0.1000000000000018235 ) ;
#22661=EDGE_LOOP ( 'NONE', ( #10633, #10908, #29961, #8636 ) ) ;
#22669=DIRECTION ( 'NONE',  ( -0.9577728606650218746, -0.2746369484007246675, 0.08512164205816423468 ) ) ;
#22672=LINE ( 'NONE', #30560, #28886 ) ;
#22674=CARTESIAN_POINT ( 'NONE',  ( -40.99173213700658636, 9.305078116158229662, 39.54930799450052348 ) ) ;
#22677=CARTESIAN_POINT ( 'NONE',  ( -40.41647043964083252, 8.356895951721261540, 59.64930799450051779 ) ) ;
#22679=CARTESIAN_POINT ( 'NONE',  ( -36.59542768321662720, 12.56771722797891400, 38.09144330556765112 ) ) ;
#22680=AXIS2_PLACEMENT_3D ( 'NONE', #18702, #18070, #28100 ) ;
#22682=CARTESIAN_POINT ( 'NONE',  ( -41.02113223168485234, 7.230835263863472306, 39.44930799450052206 ) ) ;
#22691=ORIENTED_EDGE ( 'NONE', *, *, #28945, .T. ) ;
#22694=DIRECTION ( 'NONE',  ( 1.431146867680865853E-17, 2.558717127065790464E-17, 1.000000000000000000 ) ) ;
#22695=DIRECTION ( 'NONE',  ( 0.1949050434465250392, -0.6797146636928682595, -0.7071067811865470176 ) ) ;
#22696=CARTESIAN_POINT ( 'NONE',  ( -42.03703168893574116, 3.954238390689462257, 45.74930799450051211 ) ) ;
#22699=DIRECTION ( 'NONE',  ( -2.779292025043186357E-18, 1.288349127009862057E-17, -1.000000000000000000 ) ) ;
#22704=ORIENTED_EDGE ( 'NONE', *, *, #15227, .T. ) ;
#22709=EDGE_CURVE ( 'NONE', #16387, #24759, #24547, .T. ) ;
#22712=AXIS2_PLACEMENT_3D ( 'NONE', #12284, #12122, #24254 ) ;
#22714=DIRECTION ( 'NONE',  ( -0.9612616959383221138, -0.2756373558169876170, 0.000000000000000000 ) ) ;
#22716=EDGE_LOOP ( 'NONE', ( #6809, #11913 ) ) ;
#22717=LINE ( 'NONE', #10258, #5006 ) ;
#22728=AXIS2_PLACEMENT_3D ( 'NONE', #6173, #8957, #31610 ) ;
#22732=DIRECTION ( 'NONE',  ( -0.9097384655268496711, -0.4151817967359032746, -2.088192543647023221E-17 ) ) ;
#22733=EDGE_LOOP ( 'NONE', ( #14622, #12449, #8057, #16572 ) ) ;
#22736=DIRECTION ( 'NONE',  ( 0.000000000000000000, 0.000000000000000000, -1.000000000000000000 ) ) ;
#22737=VECTOR ( 'NONE', #18596, 1000.000000000000114 ) ;
#22738=ORIENTED_EDGE ( 'NONE', *, *, #11824, .T. ) ;
#22740=LINE ( 'NONE', #10281, #16710 ) ;
#22747=ORIENTED_EDGE ( 'NONE', *, *, #25718, .F. ) ;
#22748=ORIENTED_EDGE ( 'NONE', *, *, #23430, .T. ) ;
#22756=CARTESIAN_POINT ( 'NONE',  ( -40.90015969217747482, 8.955334253785164123, 56.14611646155296398 ) ) ;
#22759=CARTESIAN_POINT ( 'NONE',  ( -43.69495677161796010, 1.169528900831203311, 60.44930799450051495 ) ) ;
#22764=DIRECTION ( 'NONE',  ( -0.4848096202463424986, -0.8746197071393928546, 2.220446049250312834E-16 ) ) ;
#22766=CARTESIAN_POINT ( 'NONE',  ( -40.09616233467386337, 6.848043556934458209, 34.82480928884837112 ) ) ;
#22770=ORIENTED_EDGE ( 'NONE', *, *, #16734, .F. ) ;
#22771=FACE_OUTER_BOUND ( 'NONE', #25130, .T. ) ;
#22774=EDGE_LOOP ( 'NONE', ( #18396, #23791, #26166, #19144 ) ) ;
#22775=CARTESIAN_POINT ( 'NONE',  ( -39.64148344771002286, 7.657122216028890982, 32.14930799450051779 ) ) ;
#22780=EDGE_LOOP ( 'NONE', ( #2807, #4212, #13152, #13763 ) ) ;
#22782=VERTEX_POINT ( 'NONE', #12995 ) ;
#22784=ADVANCED_FACE ( 'NONE', ( #22828 ), #25619, .T. ) ;
#22794=ADVANCED_FACE ( 'NONE', ( #16964 ), #31378, .F. ) ;
#22797=CARTESIAN_POINT ( 'NONE',  ( -43.95628906790246759, -0.1269931775117038586, 32.14930799450051779 ) ) ;
#22805=DIRECTION ( 'NONE',  ( 0.8746197071393926326, -0.4848096202463430537, -8.676864087101709653E-18 ) ) ;
#22806=ORIENTED_EDGE ( 'NONE', *, *, #26533, .F. ) ;
#22808=CARTESIAN_POINT ( 'NONE',  ( -42.38351229602917414, 14.72295342448899191, 58.95959122802360497 ) ) ;
#22814=CARTESIAN_POINT ( 'NONE',  ( -40.51045226066063520, 7.589116544599141534, 53.87859731638185679 ) ) ;
#22819=ADVANCED_FACE ( 'NONE', ( #20043 ), #30071, .T. ) ;
#22821=ORIENTED_EDGE ( 'NONE', *, *, #24154, .T. ) ;
#22822=ORIENTED_EDGE ( 'NONE', *, *, #16222, .T. ) ;
#22823=DIRECTION ( 'NONE',  ( 0.8746197071393926326, -0.4848096202463430537, -8.676864087101709653E-18 ) ) ;
#22828=FACE_OUTER_BOUND ( 'NONE', #27360, .T. ) ;
#22829=CARTESIAN_POINT ( 'NONE',  ( -40.67837904183829068, 9.488261090400163411, 39.44504779057211863 ) ) ;
#22831=EDGE_CURVE ( 'NONE', #15549, #24463, #7909, .T. ) ;
#22832=LINE ( 'NONE', #30233, #1953 ) ;
#22835=CARTESIAN_POINT ( 'NONE',  ( -40.51045226066063520, 7.589116544599135317, 60.22001867261916175 ) ) ;
#22836=CARTESIAN_POINT ( 'NONE',  ( -43.37834615508418068, 1.121909970995876638, 34.64930799450052490 ) ) ;
#22840=ORIENTED_EDGE ( 'NONE', *, *, #30110, .T. ) ;
#22848=VERTEX_POINT ( 'NONE', #25461 ) ;
#22849=LINE ( 'NONE', #5305, #17688 ) ;
#22858=ADVANCED_FACE ( 'NONE', ( #20358 ), #13545, .T. ) ;
#22866=CARTESIAN_POINT ( 'NONE',  ( -42.47434154250544225, 4.196643200812637531, 58.34930799450052064 ) ) ;
#22869=CARTESIAN_POINT ( 'NONE',  ( -36.76418579970419387, 10.14130568307076352, 57.95249952744806166 ) ) ;
#22875=ORIENTED_EDGE ( 'NONE', *, *, #29160, .F. ) ;
#22877=CARTESIAN_POINT ( 'NONE',  ( -40.60333149162104860, 7.557375771971046596, 54.64930799450051779 ) ) ;
#22878=( BOUNDED_CURVE ( )  B_SPLINE_CURVE ( 3, ( #11771, #11288, #4540, #18810 ),
 .UNSPECIFIED., .F., .F. ) 
 B_SPLINE_CURVE_WITH_KNOTS ( ( 4, 4 ),
 ( 2.008243333561409827, 2.704294664099573975 ),
 .UNSPECIFIED. ) 
 CURVE ( )  GEOMETRIC_REPRESENTATION_ITEM ( )  RATIONAL_B_SPLINE_CURVE ( ( 1.000000000000000000, 0.9600319177481757560, 0.9600319177481757560, 1.000000000000000000 ) ) 
 REPRESENTATION_ITEM ( '' )  );
#22884=CARTESIAN_POINT ( 'NONE',  ( -41.02113223168485234, 7.230835263863471418, 34.54930799450052348 ) ) ;
#22892=CARTESIAN_POINT ( 'NONE',  ( -42.24141723705587737, 13.63285518870473290, 59.54930799450050927 ) ) ;
#22893=CARTESIAN_POINT ( 'NONE',  ( -40.52669582637187773, 7.652910973922034010, 60.15421819779514578 ) ) ;
#22903=EDGE_LOOP ( 'NONE', ( #16192, #28520, #28425, #6771 ) ) ;
#22906=LINE ( 'NONE', #423, #13024 ) ;
#22909=EDGE_LOOP ( 'NONE', ( #17313, #27508, #24544 ) ) ;
#22916=DIRECTION ( 'NONE',  ( -0.8746197071393926326, 0.4848096202463430537, 8.676864087101709653E-18 ) ) ;
#22921=DIRECTION ( 'NONE',  ( 1.188208965918165239E-16, 1.880121038077813132E-16, 1.000000000000000000 ) ) ;
#22928=VERTEX_POINT ( 'NONE', #18382 ) ;
#22930=ORIENTED_EDGE ( 'NONE', *, *, #13278, .F. ) ;
#22939=VERTEX_POINT ( 'NONE', #6568 ) ;
#22942=DIRECTION ( 'NONE',  ( 0.8746197071393926326, -0.4848096202463430537, -8.676864087101709653E-18 ) ) ;
#22943=CARTESIAN_POINT ( 'NONE',  ( -40.02540636251513462, 2.839176264122873050, 37.04930799450052348 ) ) ;
#22949=CIRCLE ( 'NONE', #30301, 2.000000000000001776 ) ;
#22962=AXIS2_PLACEMENT_3D ( 'NONE', #5807, #5638, #8584 ) ;
#22971=EDGE_CURVE ( 'NONE', #18805, #22848, #26120, .T. ) ;
#22974=EDGE_CURVE ( 'NONE', #3661, #28974, #4091, .T. ) ;
#22975=AXIS2_PLACEMENT_3D ( 'NONE', #10364, #14522, #30386 ) ;
#22980=ORIENTED_EDGE ( 'NONE', *, *, #22431, .F. ) ;
#22982=DIRECTION ( 'NONE',  ( -1.188208965918165239E-16, -1.880121038077812885E-16, -1.000000000000000000 ) ) ;
#22984=LINE ( 'NONE', #15594, #18340 ) ;
#22985=CIRCLE ( 'NONE', #13054, 2.000000000000001776 ) ;
#22992=CARTESIAN_POINT ( 'NONE',  ( -41.93344242462055149, 13.82826554927147988, 59.53596428539564300 ) ) ;
#22994=CARTESIAN_POINT ( 'NONE',  ( -40.57832940339290673, 7.446916344587777736, 60.29072935073781991 ) ) ;
#23000=ORIENTED_EDGE ( 'NONE', *, *, #26483, .T. ) ;
#23011=CARTESIAN_POINT ( 'NONE',  ( -40.06118906035621308, 6.942907937678849173, 39.10569540309890613 ) ) ;
#23014=DIRECTION ( 'NONE',  ( 0.4848096202463429427, 0.8746197071393925215, -2.352477780477436787E-16 ) ) ;
#23018=EDGE_CURVE ( 'NONE', #30053, #14586, #26911, .T. ) ;
#23019=ORIENTED_EDGE ( 'NONE', *, *, #30808, .F. ) ;
#23036=DIRECTION ( 'NONE',  ( 0.8746197071393926326, -0.4848096202463430537, -8.676864087101709653E-18 ) ) ;
#23042=EDGE_CURVE ( 'NONE', #22928, #30572, #17237, .T. ) ;
#23045=CARTESIAN_POINT ( 'NONE',  ( -42.38687957179150345, 4.148162238788003719, 57.04930799450051637 ) ) ;
#23046=ORIENTED_EDGE ( 'NONE', *, *, #32315, .T. ) ;
#23047=DIRECTION ( 'NONE',  ( 0.000000000000000000, 0.000000000000000000, -1.000000000000000000 ) ) ;
#23052=VECTOR ( 'NONE', #15649, 1000.000000000000000 ) ;
#23062=AXIS2_PLACEMENT_3D ( 'NONE', #22682, #4964, #5455 ) ;
#23065=( BOUNDED_SURFACE ( )  B_SPLINE_SURFACE ( 3, 2, ( 
 ( #3903, #13929, #29179 ),
 ( #9315, #16533, #21129 ),
 ( #26231, #11452, #21450 ),
 ( #31486, #14088, #8679 ),
 ( #18669, #3578, #9153 ),
 ( #31652, #23608, #23924 ),
 ( #1435, #24084, #3743 ),
 ( #31323, #11147, #8827 ),
 ( #28690, #1602, #8994 ),
 ( #16211, #11623, #19152 ) ),
 .UNSPECIFIED., .F., .F., .T. ) 
 B_SPLINE_SURFACE_WITH_KNOTS ( ( 4, 2, 2, 2, 4 ),
 ( 3, 3 ),
 ( -1.680513367352531873E-18, 0.0003347409949942531512, 0.0006694819899885080371, 0.001004222984982762815, 0.001338963979977017809 ),
 ( 0.000000000000000000, 1.000000000000000000 ),
 .UNSPECIFIED. ) 
 GEOMETRIC_REPRESENTATION_ITEM ( )  RATIONAL_B_SPLINE_SURFACE ( (
 ( 1.000000000000000000, 0.7071067811865460184, 1.000000000000000000),
 ( 1.000000000000000000, 0.7102524952744432296, 1.000000000000000000),
 ( 1.000000000000000000, 0.7282169120239688764, 1.000000000000000000),
 ( 1.000000000000000000, 0.7754022835990964646, 1.000000000000000000),
 ( 1.000000000000000000, 0.8043059223103944388, 1.000000000000000000),
 ( 1.000000000000000000, 0.8571167854599045510, 1.000000000000000000),
 ( 1.000000000000000000, 0.8816198077921589826, 1.000000000000000000),
 ( 1.000000000000000000, 0.9175117844828227787, 1.000000000000000000),
 ( 1.000000000000000000, 0.9295466150067912547, 1.000000000000000000),
 ( 1.000000000000000000, 0.9308844615755744734, 1.000000000000000000) ) ) 
 REPRESENTATION_ITEM ( '' )  SURFACE ( )  );
#23069=CARTESIAN_POINT ( 'NONE',  ( -38.36853489569023168, 7.065850718397949315, 32.14930799450051779 ) ) ;
#23071=ADVANCED_FACE ( 'NONE', ( #1466 ), #24282, .F. ) ;
#23075=CARTESIAN_POINT ( 'NONE',  ( -40.23971823762673239, 6.784144620117123381, 60.54930799450051637 ) ) ;
#23076=CARTESIAN_POINT ( 'NONE',  ( -41.94956971822180947, 3.905757428664828890, 47.04930799450051637 ) ) ;
#23079=ORIENTED_EDGE ( 'NONE', *, *, #22509, .F. ) ;
#23082=CARTESIAN_POINT ( 'NONE',  ( -41.52218637998914375, 11.15499190493234671, 36.00717268343339583 ) ) ;
#23090=CARTESIAN_POINT ( 'NONE',  ( -40.51522948349269626, 7.610540244934344223, 53.90050787996893433 ) ) ;
#23096=CARTESIAN_POINT ( 'NONE',  ( -40.66259927863561785, 6.843847033173870109, 34.78317517103428003 ) ) ;
#23099=AXIS2_PLACEMENT_3D ( 'NONE', #2973, #20541, #18226 ) ;
#23100=DIRECTION ( 'NONE',  ( -2.779292025043186357E-18, 1.288349127009862211E-17, -1.000000000000000000 ) ) ;
#23102=ORIENTED_EDGE ( 'NONE', *, *, #19616, .T. ) ;
#23104=AXIS2_PLACEMENT_3D ( 'NONE', #14568, #8993, #4390 ) ;
#23110=EDGE_CURVE ( 'NONE', #110, #19940, #7701, .T. ) ;
#23112=DIRECTION ( 'NONE',  ( -0.2756373558169947779, 0.9612616959383200044, 0.000000000000000000 ) ) ;
#23117=FACE_OUTER_BOUND ( 'NONE', #22780, .T. ) ;
#23132=DIRECTION ( 'NONE',  ( 0.8746197071393926326, -0.4848096202463430537, -8.676864087101709653E-18 ) ) ;
#23135=FACE_BOUND ( 'NONE', #11657, .T. ) ;
#23136=DIRECTION ( 'NONE',  ( 0.8746197071393926326, -0.4848096202463430537, -8.676864087101709653E-18 ) ) ;
#23146=CIRCLE ( 'NONE', #24191, 0.09999999999999896472 ) ;
#23152=VERTEX_POINT ( 'NONE', #12958 ) ;
#23157=CARTESIAN_POINT ( 'NONE',  ( -42.38687957179149635, 4.148162238787999279, 37.04930799450052348 ) ) ;
#23161=DIRECTION ( 'NONE',  ( 0.4848096202463429427, 0.8746197071393925215, -2.352477780477436294E-16 ) ) ;
#23166=ADVANCED_FACE ( 'NONE', ( #22304 ), #25098, .T. ) ;
#23172=CARTESIAN_POINT ( 'NONE',  ( -42.50084779003665147, 14.56798984196178637, 37.04930799450052348 ) ) ;
#23175=FACE_BOUND ( 'NONE', #21952, .T. ) ;
#23176=VECTOR ( 'NONE', #26950, 1000.000000000000000 ) ;
#23179=CARTESIAN_POINT ( 'NONE',  ( -41.88090303775678080, 13.82677487427665497, 54.64930799450051779 ) ) ;
#23181=ORIENTED_EDGE ( 'NONE', *, *, #22709, .F. ) ;
#23195=VECTOR ( 'NONE', #8228, 1000.000000000000114 ) ;
#23196=DIRECTION ( 'NONE',  ( -0.2756373558170082672, 0.9612616959383162296, 0.000000000000000000 ) ) ;
#23198=AXIS2_PLACEMENT_3D ( 'NONE', #12929, #2421, #22422 ) ;
#23199=EDGE_LOOP ( 'NONE', ( #6330, #3072, #2059, #28191, #14835 ) ) ;
#23200=CARTESIAN_POINT ( 'NONE',  ( -41.10400476907452116, 9.333823787025618657, 38.63215070697513909 ) ) ;
#23202=DIRECTION ( 'NONE',  ( -2.779292025043186357E-18, 1.288349127009862211E-17, -1.000000000000000000 ) ) ;
#23205=AXIS2_PLACEMENT_3D ( 'NONE', #26200, #28360, #3722 ) ;
#23210=DIRECTION ( 'NONE',  ( 0.9612616959383200044, 0.2756373558169954996, -1.660411357259285896E-16 ) ) ;
#23211=PLANE ( 'NONE',  #24725 ) ;
#23212=DIRECTION ( 'NONE',  ( 2.779292025043186357E-18, -1.288349127009862211E-17, 1.000000000000000000 ) ) ;
#23213=CARTESIAN_POINT ( 'NONE',  ( -40.23397449525940317, 6.794506605641763564, 34.54930799450052348 ) ) ;
#23214=CARTESIAN_POINT ( 'NONE',  ( -40.47579404106497236, 7.230063580211346874, 38.88540821492420463 ) ) ;
#23215=EDGE_LOOP ( 'NONE', ( #32052, #7654, #26426, #356 ) ) ;
#23216=DIRECTION ( 'NONE',  ( -0.2756373558169947779, 0.9612616959383200044, 0.000000000000000000 ) ) ;
#23218=CARTESIAN_POINT ( 'NONE',  ( -42.67312000749024747, 15.16877446138198238, 35.54930799450051637 ) ) ;
#23222=DIRECTION ( 'NONE',  ( -0.2756373558170082672, 0.9612616959383162296, 0.000000000000000000 ) ) ;
#23224=CIRCLE ( 'NONE', #23733, 0.1000000000000018235 ) ;
#23227=CARTESIAN_POINT ( 'NONE',  ( -40.60333149162104860, 7.557375771971038603, 60.08350751967649472 ) ) ;
#23229=CIRCLE ( 'NONE', #26360, 1.300000000000002487 ) ;
#23233=EDGE_CURVE ( 'NONE', #8765, #14556, #19309, .T. ) ;
#23238=EDGE_LOOP ( 'NONE', ( #31510, #25812, #13923, #15484 ) ) ;
#23240=ORIENTED_EDGE ( 'NONE', *, *, #14046, .T. ) ;
#23243=FACE_OUTER_BOUND ( 'NONE', #22903, .T. ) ;
#23245=CIRCLE ( 'NONE', #5889, 2.000000000000001776 ) ;
#23251=DIRECTION ( 'NONE',  ( 7.588956326749211550E-18, -4.206627182996912454E-18, 1.000000000000000000 ) ) ;
#23253=VERTEX_POINT ( 'NONE', #8189 ) ;
#23256=DIRECTION ( 'NONE',  ( 0.4848096202463429982, 0.8746197071393925215, -4.250072516143176149E-17 ) ) ;
#23259=CIRCLE ( 'NONE', #9100, 0.1000000000000006301 ) ;
#23261=CARTESIAN_POINT ( 'NONE',  ( -41.13768170161382898, 11.26524684725914227, 35.90717268343339441 ) ) ;
#23264=VERTEX_POINT ( 'NONE', #5890 ) ;
#23267=ADVANCED_FACE ( 'NONE', ( #25900 ), #20965, .T. ) ;
#23268=ORIENTED_EDGE ( 'NONE', *, *, #25320, .T. ) ;
#23276=EDGE_CURVE ( 'NONE', #11074, #11047, #13576, .T. ) ;
#23277=AXIS2_PLACEMENT_3D ( 'NONE', #14705, #12903, #7315 ) ;
#23282=DIRECTION ( 'NONE',  ( 0.8746197071393926326, -0.4848096202463430537, -8.676864087101709653E-18 ) ) ;
#23283=DIRECTION ( 'NONE',  ( 0.2756373558170082672, -0.9612616959383162296, 0.000000000000000000 ) ) ;
#23287=VERTEX_POINT ( 'NONE', #24236 ) ;
#23288=CYLINDRICAL_SURFACE ( 'NONE', #18458, 0.1000000000000014905 ) ;
#23302=CARTESIAN_POINT ( 'NONE',  ( -40.59689739711614465, 7.533859135569301202, 60.29072935073781991 ) ) ;
#23307=EDGE_CURVE ( 'NONE', #10175, #3984, #19137, .T. ) ;
#23310=ORIENTED_EDGE ( 'NONE', *, *, #29621, .F. ) ;
#23313=ORIENTED_EDGE ( 'NONE', *, *, #24457, .T. ) ;
#23317=CIRCLE ( 'NONE', #23820, 1.142135311067127512 ) ;
#23320=CIRCLE ( 'NONE', #26453, 0.8999999999999991340 ) ;
#23323=CARTESIAN_POINT ( 'NONE',  ( -39.64148344771002286, 7.657122216028890982, 47.04930799450051637 ) ) ;
#23324=DIRECTION ( 'NONE',  ( -0.9612616959383221138, -0.2756373558169876170, 0.000000000000000000 ) ) ;
#23329=PLANE ( 'NONE',  #26240 ) ;
#23330=DIRECTION ( 'NONE',  ( 0.000000000000000000, 0.000000000000000000, -1.000000000000000000 ) ) ;
#23332=( NAMED_UNIT ( * ) PLANE_ANGLE_UNIT ( ) SI_UNIT ( $, .RADIAN. ) );
#23334=VERTEX_POINT ( 'NONE', #16360 ) ;
#23336=DIRECTION ( 'NONE',  ( -2.779292025043186357E-18, 1.288349127009862211E-17, -1.000000000000000000 ) ) ;
#23340=CARTESIAN_POINT ( 'NONE',  ( -40.65487266620045403, 9.475231293617262907, 34.66144002885648945 ) ) ;
#23342=DIRECTION ( 'NONE',  ( 0.8746197071393925215, -0.4848096202463429982, -8.676864087101708112E-18 ) ) ;
#23361=EDGE_LOOP ( 'NONE', ( #9820, #993, #289, #29012 ) ) ;
#23362=FACE_OUTER_BOUND ( 'NONE', #10038, .T. ) ;
#23363=AXIS2_PLACEMENT_3D ( 'NONE', #21525, #1350, #16766 ) ;
#23368=ORIENTED_EDGE ( 'NONE', *, *, #2719, .T. ) ;
#23370=CARTESIAN_POINT ( 'NONE',  ( -42.67844523361456766, 15.18734573188464765, 38.54111136810265492 ) ) ;
#23371=CARTESIAN_POINT ( 'NONE',  ( -42.26497471389478733, 14.66834543456875117, 55.08207028713757580 ) ) ;
#23372=CARTESIAN_POINT ( 'NONE',  ( -40.11027759654395197, 6.823245743731468416, 34.62590909864994870 ) ) ;
#23374=CARTESIAN_POINT ( 'NONE',  ( -40.47630348341015605, 7.507564784836493033, 38.76982006947343251 ) ) ;
#23375=ORIENTED_EDGE ( 'NONE', *, *, #31623, .F. ) ;
#23376=CARTESIAN_POINT ( 'NONE',  ( -42.50976151518963064, 14.59907569580870046, 37.04930799450052348 ) ) ;
#23378=FACE_OUTER_BOUND ( 'NONE', #19032, .T. ) ;
#23392=ADVANCED_FACE ( 'NONE', ( #11611 ), #23914, .T. ) ;
#23397=VERTEX_POINT ( 'NONE', #4379 ) ;
#23406=CARTESIAN_POINT ( 'NONE',  ( -40.15599670534037102, 7.478908884098773413, 38.19144330556764544 ) ) ;
#23410=LINE ( 'NONE', #3701, #28965 ) ;
#23414=CARTESIAN_POINT ( 'NONE',  ( -40.51045226066063520, 7.589116544599140646, 53.87859731638185679 ) ) ;
#23417=ORIENTED_EDGE ( 'NONE', *, *, #31861, .T. ) ;
#23419=CARTESIAN_POINT ( 'NONE',  ( -40.55615437192401629, 7.233232712783719265, 35.22901891019329668 ) ) ;
#23420=ORIENTED_EDGE ( 'NONE', *, *, #31424, .T. ) ;
#23429=VERTEX_POINT ( 'NONE', #25055 ) ;
#23430=EDGE_CURVE ( 'NONE', #29694, #6106, #2412, .T. ) ;
#23431=AXIS2_PLACEMENT_3D ( 'NONE', #23376, #3180, #23216 ) ;
#23436=CARTESIAN_POINT ( 'NONE',  ( -40.47970302497625994, 7.463434137431151250, 60.44930799450051495 ) ) ;
#23443=CARTESIAN_POINT ( 'NONE',  ( -41.02113223168485234, 7.230835263863471418, 34.64930799450051779 ) ) ;
#23448=AXIS2_PLACEMENT_3D ( 'NONE', #28416, #13640, #11334 ) ;
#23452=CARTESIAN_POINT ( 'NONE',  ( -42.68334051588268352, -0.7182646751426445819, 62.04930799450052348 ) ) ;
#23456=EDGE_CURVE ( 'NONE', #18307, #16525, #18310, .T. ) ;
#23464=CARTESIAN_POINT ( 'NONE',  ( -42.50976151518963064, 14.59907569580870046, 36.00717268343339583 ) ) ;
#23465=CARTESIAN_POINT ( 'NONE',  ( -40.59711871614117484, 7.548154485354792165, 53.86460186241264125 ) ) ;
#23466=VECTOR ( 'NONE', #17819, 1000.000000000000000 ) ;
#23469=ORIENTED_EDGE ( 'NONE', *, *, #10656, .T. ) ;
#23471=VECTOR ( 'NONE', #16321, 999.9999999999998863 ) ;
#23483=ORIENTED_EDGE ( 'NONE', *, *, #16041, .T. ) ;
#23486=CARTESIAN_POINT ( 'NONE',  ( -40.88331355377635390, 6.750204415894309307, 34.54930799450052348 ) ) ;
#23487=DIRECTION ( 'NONE',  ( -1.188208965918165239E-16, -1.880121038077813132E-16, -1.000000000000000000 ) ) ;
#23488=FACE_OUTER_BOUND ( 'NONE', #20862, .T. ) ;
#23489=CARTESIAN_POINT ( 'NONE',  ( -41.01929587258828036, 9.401204285752060130, 38.64930799450052490 ) ) ;
#23490=ORIENTED_EDGE ( 'NONE', *, *, #24800, .T. ) ;
#23491=ORIENTED_EDGE ( 'NONE', *, *, #22831, .T. ) ;
#23499=CARTESIAN_POINT ( 'NONE',  ( -40.05987053574653345, 7.506472619680473635, 38.70582007960419446 ) ) ;
#23500=EDGE_LOOP ( 'NONE', ( #4930, #21764, #20182, #19913 ) ) ;
#23501=DIRECTION ( 'NONE',  ( 7.588956326749211550E-18, -4.206627182996912454E-18, 1.000000000000000000 ) ) ;
#23511=FACE_OUTER_BOUND ( 'NONE', #25742, .T. ) ;
#23513=DIRECTION ( 'NONE',  ( -0.8746197071393926326, 0.4848096202463430537, 8.676864087101709653E-18 ) ) ;
#23514=DIRECTION ( 'NONE',  ( 0.000000000000000000, 0.000000000000000000, 1.000000000000000000 ) ) ;
#23518=TOROIDAL_SURFACE ( 'NONE', #29311, 1.899999999999999467, 0.1000000000000000056 ) ;
#23522=DIRECTION ( 'NONE',  ( -1.188208965918165239E-16, -1.880121038077813132E-16, -1.000000000000000000 ) ) ;
#23531=LINE ( 'NONE', #12900, #11090 ) ;
#23532=VERTEX_POINT ( 'NONE', #23075 ) ;
#23535=LINE ( 'NONE', #23218, #26926 ) ;
#23537=DIRECTION ( 'NONE',  ( -0.9612616959383221138, -0.2756373558169876170, 0.000000000000000000 ) ) ;
#23539=CARTESIAN_POINT ( 'NONE',  ( -43.29662792673756400, 1.063067023446606196, 60.44930799450051495 ) ) ;
#23542=CARTESIAN_POINT ( 'NONE',  ( -40.51522877113607279, 7.610537050327685904, 60.19811137623720754 ) ) ;
#23543=VERTEX_POINT ( 'NONE', #5854 ) ;
#23550=DIRECTION ( 'NONE',  ( 0.9612616959383205595, 0.2756373558169932236, -1.660411357259282445E-16 ) ) ;
#23553=DIRECTION ( 'NONE',  ( -0.1949050434465268433, 0.6797146636928679264, 0.7071067811865469066 ) ) ;
#23562=CARTESIAN_POINT ( 'NONE',  ( -43.29088418437023478, 1.073429008971242382, 34.64930799450052490 ) ) ;
#23565=ORIENTED_EDGE ( 'NONE', *, *, #931, .T. ) ;
#23566=DIRECTION ( 'NONE',  ( 0.8746197071393858602, -0.4848096202463547666, 0.000000000000000000 ) ) ;
#23567=CIRCLE ( 'NONE', #3630, 1.142135311067127512 ) ;
#23581=VECTOR ( 'NONE', #24999, 1000.000000000000227 ) ;
#23587=CARTESIAN_POINT ( 'NONE',  ( -40.05987053574653345, 7.506472619680472746, 38.70582007960419446 ) ) ;
#23592=EDGE_LOOP ( 'NONE', ( #12234, #32448, #2369, #1944 ) ) ;
#23602=AXIS2_PLACEMENT_3D ( 'NONE', #1833, #18892, #24314 ) ;
#23603=VECTOR ( 'NONE', #7450, 1000.000000000000227 ) ;
#23608=CARTESIAN_POINT ( 'NONE',  ( -40.59768508530202524, 7.003142309055506054, 39.05686288009237472 ) ) ;
#23609=CARTESIAN_POINT ( 'NONE',  ( -40.68642432603660808, 6.803331639906144090, 39.34088707671027407 ) ) ;
#23619=VECTOR ( 'NONE', #11533, 1000.000000000000000 ) ;
#23621=DIRECTION ( 'NONE',  ( 0.9612616959383221138, 0.2756373558169876170, 0.000000000000000000 ) ) ;
#23625=CARTESIAN_POINT ( 'NONE',  ( -41.91739890389096956, 13.90674392281398930, 59.49868301348410426 ) ) ;
#23626=DIRECTION ( 'NONE',  ( 0.9612616959383200044, 0.2756373558169954996, -1.660411357259285896E-16 ) ) ;
#23633=VERTEX_POINT ( 'NONE', #11102 ) ;
#23638=CIRCLE ( 'NONE', #17856, 0.1000000000000008243 ) ;
#23640=ORIENTED_EDGE ( 'NONE', *, *, #1016, .F. ) ;
#23646=EDGE_LOOP ( 'NONE', ( #27503, #28113, #11820 ) ) ;
#23656=DIRECTION ( 'NONE',  ( -0.4848096202463424431, -0.8746197071393927436, 2.220446049250312588E-16 ) ) ;
#23661=CARTESIAN_POINT ( 'NONE',  ( -36.18493864628602807, 8.798967949527998655, 53.54930799450051637 ) ) ;
#23663=ORIENTED_EDGE ( 'NONE', *, *, #27057, .T. ) ;
#23664=CARTESIAN_POINT ( 'NONE',  ( -40.69571722278731585, 6.786566810383049209, 39.44930799450052206 ) ) ;
#23677=CARTESIAN_POINT ( 'NONE',  ( -43.64647580959332629, 1.256990871545142330, 53.64930799450051779 ) ) ;
#23684=VERTEX_POINT ( 'NONE', #16640 ) ;
#23685=FACE_OUTER_BOUND ( 'NONE', #12568, .T. ) ;
#23689=ORIENTED_EDGE ( 'NONE', *, *, #24108, .T. ) ;
#23698=CARTESIAN_POINT ( 'NONE',  ( -41.56459318755936749, 7.281738416154046156, 60.44930799450051495 ) ) ;
#23701=DIRECTION ( 'NONE',  ( 0.8746197071393925215, -0.4848096202463429982, -8.676864087101708112E-18 ) ) ;
#23721=CARTESIAN_POINT ( 'NONE',  ( -42.36691375901575185, 13.72999064396537250, 54.61480954800870791 ) ) ;
#23726=DIRECTION ( 'NONE',  ( -0.9612616959383205595, -0.2756373558169931681, 1.660411357259282445E-16 ) ) ;
#23728=ORIENTED_EDGE ( 'NONE', *, *, #8744, .T. ) ;
#23732=FACE_OUTER_BOUND ( 'NONE', #1480, .T. ) ;
#23733=AXIS2_PLACEMENT_3D ( 'NONE', #3264, #31164, #28062 ) ;
#23736=CARTESIAN_POINT ( 'NONE',  ( -40.47576471041902124, 7.229986682739586890, 35.21321334501939049 ) ) ;
#23739=DIRECTION ( 'NONE',  ( -0.8746197071393927436, 0.4848096202463423876, 1.277302113040827440E-17 ) ) ;
#23742=EDGE_LOOP ( 'NONE', ( #5171, #6122, #17087, #26339 ) ) ;
#23747=ORIENTED_EDGE ( 'NONE', *, *, #2271, .F. ) ;
#23751=EDGE_LOOP ( 'NONE', ( #1368, #30272, #7602, #27415 ) ) ;
#23760=ORIENTED_EDGE ( 'NONE', *, *, #10686, .F. ) ;
#23763=CARTESIAN_POINT ( 'NONE',  ( -43.64647580959332629, 1.256990871545142330, 53.54930799450051637 ) ) ;
#23770=FACE_OUTER_BOUND ( 'NONE', #27678, .T. ) ;
#23771=FACE_OUTER_BOUND ( 'NONE', #27919, .T. ) ;
#23774=AXIS2_PLACEMENT_3D ( 'NONE', #23677, #28598, #15637 ) ;
#23779=DIRECTION ( 'NONE',  ( -0.7141240004913198547, 0.3958453973320100738, 0.5773502691896283956 ) ) ;
#23783=ADVANCED_FACE ( 'NONE', ( #28972 ), #6488, .T. ) ;
#23785=EDGE_CURVE ( 'NONE', #11711, #20495, #5257, .T. ) ;
#23786=EDGE_LOOP ( 'NONE', ( #2916, #14397, #24424, #2762 ) ) ;
#23788=CARTESIAN_POINT ( 'NONE',  ( -42.36153388572594736, 13.68895619636815653, 59.44930799450051495 ) ) ;
#23789=CARTESIAN_POINT ( 'NONE',  ( -40.72710635398858869, 8.382218338248518918, 40.36793714460204541 ) ) ;
#23791=ORIENTED_EDGE ( 'NONE', *, *, #30850, .T. ) ;
#23792=AXIS2_PLACEMENT_3D ( 'NONE', #18253, #10737, #13677 ) ;
#23796=ORIENTED_EDGE ( 'NONE', *, *, #5187, .T. ) ;
#23797=DIRECTION ( 'NONE',  ( -0.8746197071393926326, 0.4848096202463430537, 8.676864087101709653E-18 ) ) ;
#23798=VERTEX_POINT ( 'NONE', #75 ) ;
#23800=FACE_OUTER_BOUND ( 'NONE', #31119, .T. ) ;
#23801=CARTESIAN_POINT ( 'NONE',  ( -42.21246928125516718, 14.65068104870687726, 37.04930799450052348 ) ) ;
#23804=ORIENTED_EDGE ( 'NONE', *, *, #31470, .F. ) ;
#23808=EDGE_LOOP ( 'NONE', ( #31479, #23491, #12631, #27813 ) ) ;
#23817=CIRCLE ( 'NONE', #13868, 1.199999999999999734 ) ;
#23818=CIRCLE ( 'NONE', #13870, 2.000000000000001776 ) ;
#23820=AXIS2_PLACEMENT_3D ( 'NONE', #1761, #6855, #4230 ) ;
#23835=DIRECTION ( 'NONE',  ( -0.4848096202463427762, -0.8746197071393926326, 0.000000000000000000 ) ) ;
#23836=CARTESIAN_POINT ( 'NONE',  ( -40.40505316653322865, 8.317079188576510518, 59.54930799450052348 ) ) ;
#23837=AXIS2_PLACEMENT_3D ( 'NONE', #22943, #23282, #793 ) ;
#23838=EDGE_CURVE ( 'NONE', #25211, #25249, #22383, .T. ) ;
#23841=PLANE ( 'NONE',  #16030 ) ;
#23846=EDGE_CURVE ( 'NONE', #31307, #23684, #9446, .T. ) ;
#23848=VECTOR ( 'NONE', #32161, 1000.000000000000000 ) ;
#23855=CARTESIAN_POINT ( 'NONE',  ( -43.38408989745150990, 1.111547985471240008, 53.54930799450051637 ) ) ;
#23858=EDGE_CURVE ( 'NONE', #9599, #11721, #8034, .T. ) ;
#23863=CARTESIAN_POINT ( 'NONE',  ( -41.01929587258828747, 9.401204285752060130, 39.44930799450052206 ) ) ;
#23865=ORIENTED_EDGE ( 'NONE', *, *, #32030, .F. ) ;
#23872=LINE ( 'NONE', #1382, #14500 ) ;
#23873=DIRECTION ( 'NONE',  ( 0.4848096202463636484, 0.8746197071393810862, 0.000000000000000000 ) ) ;
#23880=DIRECTION ( 'NONE',  ( 0.000000000000000000, 0.000000000000000000, -1.000000000000000000 ) ) ;
#23881=EDGE_CURVE ( 'NONE', #8349, #802, #9955, .T. ) ;
#23888=ORIENTED_EDGE ( 'NONE', *, *, #12216, .T. ) ;
#23891=CARTESIAN_POINT ( 'NONE',  ( -40.73091736380679606, 9.483895492497156354, 35.44930799450052206 ) ) ;
#23893=CARTESIAN_POINT ( 'NONE',  ( -43.90780810587784089, -0.03953120679776531143, 47.04930799450051637 ) ) ;
#23899=LINE ( 'NONE', #13575, #26640 ) ;
#23905=ORIENTED_EDGE ( 'NONE', *, *, #24033, .T. ) ;
#23906=VERTEX_POINT ( 'NONE', #24525 ) ;
#23907=UNCERTAINTY_MEASURE_WITH_UNIT (LENGTH_MEASURE( 1.000000000000000082E-05 ), #18947, 'distance_accuracy_value', 'NONE');
#23909=ORIENTED_EDGE ( 'NONE', *, *, #14382, .F. ) ;
#23910=FACE_OUTER_BOUND ( 'NONE', #14786, .T. ) ;
#23913=DIRECTION ( 'NONE',  ( 0.2756373558169954996, -0.9612616959383200044, 2.463803012461673974E-31 ) ) ;
#23914=SPHERICAL_SURFACE ( 'NONE', #30908, 0.1000000000000000056 ) ;
#23916=CARTESIAN_POINT ( 'NONE',  ( -42.21195563036361875, 4.051200314738730768, 37.04930799450052348 ) ) ;
#23924=CARTESIAN_POINT ( 'NONE',  ( -40.54123211584759190, 7.002658380791086046, 39.07840589319199864 ) ) ;
#23925=CARTESIAN_POINT ( 'NONE',  ( -40.69503817910556620, 6.787791837612842549, 39.43724091009085697 ) ) ;
#23926=CARTESIAN_POINT ( 'NONE',  ( -40.86580004447909431, 8.503105189880381332, 39.44930799450052206 ) ) ;
#23928=DIRECTION ( 'NONE',  ( 0.8746197071393926326, -0.4848096202463430537, -8.676864087101709653E-18 ) ) ;
#23929=CARTESIAN_POINT ( 'NONE',  ( -41.24971778908466291, 11.62557032131817358, 58.05249952744806308 ) ) ;
#23931=DIRECTION ( 'NONE',  ( 0.1949050434465247617, -0.6797146636928672603, -0.7071067811865480168 ) ) ;
#23935=DIRECTION ( 'NONE',  ( 0.8746197071393926326, -0.4848096202463430537, -8.676864087101709653E-18 ) ) ;
#23945=ORIENTED_EDGE ( 'NONE', *, *, #31531, .T. ) ;
#23949=CARTESIAN_POINT ( 'NONE',  ( -40.78148461367150901, 8.178669543025179678, 59.57859731638185963 ) ) ;
#23956=CARTESIAN_POINT ( 'NONE',  ( -40.09211399732166115, 9.667069410243957606, 35.44930799450052206 ) ) ;
#23958=CARTESIAN_POINT ( 'NONE',  ( -42.46007270772396680, 14.70100007970371792, 58.95278695508191191 ) ) ;
#23961=DIRECTION ( 'NONE',  ( 0.4848096202463645921, 0.8746197071393805311, 0.000000000000000000 ) ) ;
#23964=ORIENTED_EDGE ( 'NONE', *, *, #10572, .F. ) ;
#23967=ADVANCED_FACE ( 'NONE', ( #18262 ), #873, .T. ) ;
#23975=EDGE_CURVE ( 'NONE', #9470, #4922, #17806, .T. ) ;
#23983=CIRCLE ( 'NONE', #25049, 0.1000000000000014905 ) ;
#23986=CARTESIAN_POINT ( 'NONE',  ( -40.59298576501942790, 7.024321269945727586, 35.15525576937660190 ) ) ;
#23988=AXIS2_PLACEMENT_3D ( 'NONE', #69, #2373, #27806 ) ;
#23989=VERTEX_POINT ( 'NONE', #25507 ) ;
#23991=DIRECTION ( 'NONE',  ( -0.8746197071393925215, 0.4848096202463429982, 8.676864087101708112E-18 ) ) ;
#23995=FACE_OUTER_BOUND ( 'NONE', #29671, .T. ) ;
#23997=DIRECTION ( 'NONE',  ( 0.9612616959383207815, 0.2756373558169926685, 8.795445018804289444E-19 ) ) ;
#24005=CARTESIAN_POINT ( 'NONE',  ( -40.11729073372970333, 6.802967823440400075, 34.64930799450051779 ) ) ;
#24011=DIRECTION ( 'NONE',  ( -2.779292025043186357E-18, 1.288349127009862211E-17, -1.000000000000000000 ) ) ;
#24017=FACE_OUTER_BOUND ( 'NONE', #25113, .T. ) ;
#24022=ORIENTED_EDGE ( 'NONE', *, *, #21210, .F. ) ;
#24023=ORIENTED_EDGE ( 'NONE', *, *, #13583, .T. ) ;
#24031=CARTESIAN_POINT ( 'NONE',  ( -40.49636040740121956, 6.939949491715666774, 34.54930799450052348 ) ) ;
#24032=EDGE_CURVE ( 'NONE', #777, #3764, #30442, .T. ) ;
#24033=EDGE_CURVE ( 'NONE', #1812, #2291, #25347, .T. ) ;
#24039=ORIENTED_EDGE ( 'NONE', *, *, #32359, .F. ) ;
#24046=DIRECTION ( 'NONE',  ( 0.4848096202463429427, 0.8746197071393925215, -2.352477780477436294E-16 ) ) ;
#24053=ORIENTED_EDGE ( 'NONE', *, *, #8385, .F. ) ;
#24058=DIRECTION ( 'NONE',  ( 0.000000000000000000, 0.000000000000000000, 1.000000000000000000 ) ) ;
#24060=ORIENTED_EDGE ( 'NONE', *, *, #24761, .F. ) ;
#24067=EDGE_CURVE ( 'NONE', #6401, #11200, #24323, .T. ) ;
#24077=ORIENTED_EDGE ( 'NONE', *, *, #1295, .T. ) ;
#24078=DIRECTION ( 'NONE',  ( 0.4848096202463673676, 0.8746197071393789768, 0.000000000000000000 ) ) ;
#24081=CARTESIAN_POINT ( 'NONE',  ( -39.84249199961863042, 8.796534049953976364, 39.44930799450052206 ) ) ;
#24084=CARTESIAN_POINT ( 'NONE',  ( -40.62121046050631179, 6.937850113512377348, 39.13688957799512025 ) ) ;
#24088=AXIS2_PLACEMENT_3D ( 'NONE', #19825, #12791, #5066 ) ;
#24090=FACE_OUTER_BOUND ( 'NONE', #30181, .T. ) ;
#24093=AXIS2_PLACEMENT_3D ( 'NONE', #13535, #31581, #23537 ) ;
#24101=DIRECTION ( 'NONE',  ( 0.4848096202463673121, 0.8746197071393789768, 0.000000000000000000 ) ) ;
#24105=EDGE_CURVE ( 'NONE', #9695, #7978, #14001, .T. ) ;
#24107=AXIS2_PLACEMENT_3D ( 'NONE', #699, #2835, #8098 ) ;
#24108=EDGE_CURVE ( 'NONE', #25827, #17347, #28938, .T. ) ;
#24109=VECTOR ( 'NONE', #15496, 1000.000000000000000 ) ;
#24111=VECTOR ( 'NONE', #16276, 1000.000000000000000 ) ;
#24114=DIRECTION ( 'NONE',  ( -0.1949050434465251780, 0.6797146636928671493, -0.7071067811865481278 ) ) ;
#24117=DIRECTION ( 'NONE',  ( 0.9612616959383206705, 0.2756373558169926130, 8.795445018804289444E-19 ) ) ;
#24122=DIRECTION ( 'NONE',  ( 0.000000000000000000, -8.673617379884027583E-16, -1.000000000000000000 ) ) ;
#24123=ORIENTED_EDGE ( 'NONE', *, *, #24831, .T. ) ;
#24128=ORIENTED_EDGE ( 'NONE', *, *, #27599, .T. ) ;
#24130=CARTESIAN_POINT ( 'NONE',  ( -40.23967075304302909, 7.740322171013528596, 60.29072935073781991 ) ) ;
#24135=ORIENTED_EDGE ( 'NONE', *, *, #22509, .T. ) ;
#24136=CIRCLE ( 'NONE', #8424, 0.1000000000000006301 ) ;
#24144=CARTESIAN_POINT ( 'NONE',  ( -40.70217169293939463, 9.596168124565082280, 38.54930799450053058 ) ) ;
#24146=ORIENTED_EDGE ( 'NONE', *, *, #13952, .F. ) ;
#24148=DIRECTION ( 'NONE',  ( 0.9097384655268497822, 0.4151817967359032191, 2.820562191637069803E-18 ) ) ;
#24151=EDGE_CURVE ( 'NONE', #28989, #26286, #31564, .T. ) ;
#24152=ORIENTED_EDGE ( 'NONE', *, *, #9066, .F. ) ;
#24154=EDGE_CURVE ( 'NONE', #6349, #31093, #9994, .T. ) ;
#24155=AXIS2_PLACEMENT_3D ( 'NONE', #31490, #21786, #9652 ) ;
#24156=DIRECTION ( 'NONE',  ( -0.2756373558170082672, 0.9612616959383162296, 0.000000000000000000 ) ) ;
#24163=DIRECTION ( 'NONE',  ( 0.8746197071393925215, -0.4848096202463429982, -8.676864087101709653E-18 ) ) ;
#24166=ORIENTED_EDGE ( 'NONE', *, *, #26449, .T. ) ;
#24169=CARTESIAN_POINT ( 'NONE',  ( -40.39264216188491474, 8.574558558407114006, 34.58262810048215385 ) ) ;
#24170=DIRECTION ( 'NONE',  ( -2.779292025043186357E-18, 1.288349127009862211E-17, -1.000000000000000000 ) ) ;
#24172=ORIENTED_EDGE ( 'NONE', *, *, #8193, .T. ) ;
#24173=DIRECTION ( 'NONE',  ( 0.9097384655268497822, 0.4151817967359032191, 2.820562191637069417E-18 ) ) ;
#24174=CARTESIAN_POINT ( 'NONE',  ( -40.18454328187963398, 7.548069831825863218, 53.64930799450051779 ) ) ;
#24176=ORIENTED_EDGE ( 'NONE', *, *, #13181, .F. ) ;
#24177=DIRECTION ( 'NONE',  ( 0.000000000000000000, 0.000000000000000000, 1.000000000000000000 ) ) ;
#24182=EDGE_LOOP ( 'NONE', ( #11384, #29996, #24907, #7366 ) ) ;
#24185=ORIENTED_EDGE ( 'NONE', *, *, #20525, .F. ) ;
#24186=AXIS2_PLACEMENT_3D ( 'NONE', #29790, #17302, #4842 ) ;
#24190=PLANE ( 'NONE',  #31004 ) ;
#24191=AXIS2_PLACEMENT_3D ( 'NONE', #4551, #2087, #14737 ) ;
#24197=CARTESIAN_POINT ( 'NONE',  ( -40.02540636251513462, 2.839176264122873050, 39.04930799450052348 ) ) ;
#24198=ADVANCED_FACE ( 'NONE', ( #21695 ), #31723, .F. ) ;
#24199=EDGE_CURVE ( 'NONE', #7112, #27336, #21356, .T. ) ;
#24201=DIRECTION ( 'NONE',  ( -0.9612616959383083470, -0.2756373558170356897, 0.000000000000000000 ) ) ;
#24204=VECTOR ( 'NONE', #12101, 1000.000000000000114 ) ;
#24206=CIRCLE ( 'NONE', #9550, 1.899999999999999023 ) ;
#24208=FACE_OUTER_BOUND ( 'NONE', #7532, .T. ) ;
#24209=ORIENTED_EDGE ( 'NONE', *, *, #31392, .T. ) ;
#24224=CARTESIAN_POINT ( 'NONE',  ( -40.02540636251513462, 2.839176264122873050, 39.04930799450052348 ) ) ;
#24227=ORIENTED_EDGE ( 'NONE', *, *, #9990, .T. ) ;
#24236=CARTESIAN_POINT ( 'NONE',  ( -40.41647043964083252, 8.356895951721261540, 54.54930799450051637 ) ) ;
#24238=CARTESIAN_POINT ( 'NONE',  ( -40.50727813154207269, 7.559769128450253284, 53.81525338917477796 ) ) ;
#24249=DIRECTION ( 'NONE',  ( 0.2756373558169947779, -0.9612616959383200044, 0.000000000000000000 ) ) ;
#24254=DIRECTION ( 'NONE',  ( 0.7141240004913296247, -0.3958453973319808195, 0.5773502691896363892 ) ) ;
#24258=DIRECTION ( 'NONE',  ( 0.000000000000000000, -6.672013369141553384E-16, 1.000000000000000000 ) ) ;
#24260=EDGE_CURVE ( 'NONE', #382, #15550, #32048, .T. ) ;
#24264=DIRECTION ( 'NONE',  ( -1.431146867680865853E-17, -2.558717127065790464E-17, -1.000000000000000000 ) ) ;
#24267=FACE_OUTER_BOUND ( 'NONE', #26390, .T. ) ;
#24269=ADVANCED_FACE ( 'NONE', ( #14493, #14816 ), #7094, .T. ) ;
#24282=PLANE ( 'NONE',  #12548 ) ;
#24287=VERTEX_POINT ( 'NONE', #24656 ) ;
#24289=DIRECTION ( 'NONE',  ( -2.779292025043186357E-18, 1.288349127009862211E-17, -1.000000000000000000 ) ) ;
#24290=CIRCLE ( 'NONE', #188, 1.500000000000001332 ) ;
#24298=CIRCLE ( 'NONE', #9636, 0.1000000000000006301 ) ;
#24309=DIRECTION ( 'NONE',  ( 0.3428121700606640565, 0.6184495258776567805, -0.7071067811865474617 ) ) ;
#24314=DIRECTION ( 'NONE',  ( 0.4848096202463636484, 0.8746197071393810862, 0.000000000000000000 ) ) ;
#24318=CARTESIAN_POINT ( 'NONE',  ( -40.35915383839597581, 8.550197532140535017, 39.44930799450052206 ) ) ;
#24319=FACE_OUTER_BOUND ( 'NONE', #11242, .T. ) ;
#24323=LINE ( 'NONE', #26466, #17308 ) ;
#24327=DIRECTION ( 'NONE',  ( -2.779292025043186357E-18, 1.288349127009862211E-17, -1.000000000000000000 ) ) ;
#24328=CYLINDRICAL_SURFACE ( 'NONE', #30468, 0.9031915329475500576 ) ;
#24329=VECTOR ( 'NONE', #20884, 1000.000000000000000 ) ;
#24331=CARTESIAN_POINT ( 'NONE',  ( -40.41647043964083252, 8.356895951721261540, 59.44930799450051495 ) ) ;
#24332=CARTESIAN_POINT ( 'NONE',  ( -42.21246928125516718, 14.65068104870687726, 37.04930799450052348 ) ) ;
#24336=CARTESIAN_POINT ( 'NONE',  ( -40.11729073372970333, 6.802967823440400963, 39.44930799450052206 ) ) ;
#24343=TOROIDAL_SURFACE ( 'NONE', #10205, 1.899999999999999467, 0.1000000000000000056 ) ;
#24345=ADVANCED_FACE ( 'NONE', ( #38 ), #7263, .T. ) ;
#24346=ORIENTED_EDGE ( 'NONE', *, *, #24638, .T. ) ;
#24349=EDGE_LOOP ( 'NONE', ( #1180, #831, #25371, #9520 ) ) ;
#24352=AXIS2_PLACEMENT_3D ( 'NONE', #28249, #990, #25936 ) ;
#24353=B_SPLINE_CURVE_WITH_KNOTS ( 'NONE', 3,
 ( #16850, #14242, #16676, #14078, #26701, #1261, #29327, #24238, #19303, #6364 ),
 .UNSPECIFIED., .F., .F.,
 ( 4, 3, 3, 4 ),
 ( 0.000000000000000000, 3.371050856462795163E-05, 6.737649377718237724E-05, 7.827667330985808435E-05 ),
 .UNSPECIFIED. ) ;
#24354=CARTESIAN_POINT ( 'NONE',  ( -42.30123736278718383, 13.66041317296246937, 59.53596428539564300 ) ) ;
#24360=ORIENTED_EDGE ( 'NONE', *, *, #29461, .T. ) ;
#24364=DIRECTION ( 'NONE',  ( 0.000000000000000000, 0.000000000000000000, 1.000000000000000000 ) ) ;
#24365=DIRECTION ( 'NONE',  ( 0.8746197071393895239, -0.4848096202463486604, -1.277302113040671208E-17 ) ) ;
#24366=CARTESIAN_POINT ( 'NONE',  ( -40.65766396543777716, 6.815881913223422295, 39.50959409847852299 ) ) ;
#24371=DIRECTION ( 'NONE',  ( 0.2756373558169947779, -0.9612616959383203374, -1.385316060672546240E-15 ) ) ;
#24376=CARTESIAN_POINT ( 'NONE',  ( -40.12099660621151997, 7.356848571226008993, 35.24284630439623811 ) ) ;
#24382=CIRCLE ( 'NONE', #31724, 2.000000000000001776 ) ;
#24383=EDGE_CURVE ( 'NONE', #21242, #17105, #13667, .T. ) ;
#24393=CARTESIAN_POINT ( 'NONE',  ( -40.11286833322908052, 2.887657226147509970, 55.04930799450051637 ) ) ;
#24397=CARTESIAN_POINT ( 'NONE',  ( -40.69193635511749108, 9.347952559758583746, 39.44930799450052206 ) ) ;
#24399=DIRECTION ( 'NONE',  ( 0.000000000000000000, 0.000000000000000000, 1.000000000000000000 ) ) ;
#24412=CARTESIAN_POINT ( 'NONE',  ( -39.64148344771002286, 7.657122216028890982, 32.14930799450051779 ) ) ;
#24419=FACE_BOUND ( 'NONE', #5083, .T. ) ;
#24420=DIRECTION ( 'NONE',  ( -0.2756373558169974980, 0.9612616959383193382, 1.315048337272770589E-17 ) ) ;
#24424=ORIENTED_EDGE ( 'NONE', *, *, #27305, .F. ) ;
#24431=ORIENTED_EDGE ( 'NONE', *, *, #5815, .T. ) ;
#24433=DIRECTION ( 'NONE',  ( -0.8746197071393925215, 0.4848096202463429982, 8.676864087101709653E-18 ) ) ;
#24439=CARTESIAN_POINT ( 'NONE',  ( -40.23672901771082877, 7.760455916344220384, 34.54930799450052348 ) ) ;
#24440=LINE ( 'NONE', #17210, #17041 ) ;
#24441=CARTESIAN_POINT ( 'NONE',  ( -40.05987053574653345, 7.506472619680472746, 38.70582007960419446 ) ) ;
#24444=VERTEX_POINT ( 'NONE', #27932 ) ;
#24448=PLANE ( 'NONE',  #30757 ) ;
#24451=CARTESIAN_POINT ( 'NONE',  ( -39.81510167530662159, 8.701012637326792643, 39.46050754198200394 ) ) ;
#24453=ORIENTED_EDGE ( 'NONE', *, *, #25972, .F. ) ;
#24457=EDGE_CURVE ( 'NONE', #15237, #17902, #14747, .T. ) ;
#24460=ORIENTED_EDGE ( 'NONE', *, *, #9416, .F. ) ;
#24462=DIRECTION ( 'NONE',  ( -0.8746197071393925215, 0.4848096202463429982, 8.676864087101708112E-18 ) ) ;
#24463=VERTEX_POINT ( 'NONE', #15778 ) ;
#24466=EDGE_CURVE ( 'NONE', #24759, #2133, #5453, .T. ) ;
#24469=ORIENTED_EDGE ( 'NONE', *, *, #20268, .T. ) ;
#24471=PLANE ( 'NONE',  #13862 ) ;
#24475=ADVANCED_FACE ( 'NONE', ( #23488 ), #23329, .F. ) ;
#24476=EDGE_LOOP ( 'NONE', ( #12272, #2179, #24729, #17948, #12439, #26472 ) ) ;
#24477=DIRECTION ( 'NONE',  ( -7.588956326749211550E-18, 4.206627182996912454E-18, -1.000000000000000000 ) ) ;
#24478=DIRECTION ( 'NONE',  ( -0.4848096202462977566, -0.8746197071394176126, 0.000000000000000000 ) ) ;
#24484=CARTESIAN_POINT ( 'NONE',  ( -40.02540636251514172, 2.839176264122877047, 57.04930799450051637 ) ) ;
#24489=ORIENTED_EDGE ( 'NONE', *, *, #11824, .F. ) ;
#24490=CYLINDRICAL_SURFACE ( 'NONE', #5030, 0.7928932188134565351 ) ;
#24493=AXIS2_PLACEMENT_3D ( 'NONE', #31360, #18540, #28573 ) ;
#24501=FACE_OUTER_BOUND ( 'NONE', #27553, .T. ) ;
#24504=VECTOR ( 'NONE', #3754, 1000.000000000000227 ) ;
#24525=CARTESIAN_POINT ( 'NONE',  ( -40.68997348041997952, 6.796928795907699161, 60.44930799450051495 ) ) ;
#24528=CARTESIAN_POINT ( 'NONE',  ( -43.72819403793993587, 1.315833819094414769, 39.54930799450052348 ) ) ;
#24530=CARTESIAN_POINT ( 'NONE',  ( -42.66751614955960292, 15.14923148629343608, 35.54930799450051637 ) ) ;
#24532=LINE ( 'NONE', #2051, #21546 ) ;
#24534=FACE_OUTER_BOUND ( 'NONE', #20042, .T. ) ;
#24544=ORIENTED_EDGE ( 'NONE', *, *, #626, .F. ) ;
#24545=EDGE_LOOP ( 'NONE', ( #14108, #6433, #7212, #15500 ) ) ;
#24547=CIRCLE ( 'NONE', #11448, 0.1000000000000018235 ) ;
#24550=AXIS2_PLACEMENT_3D ( 'NONE', #18872, #28263, #28584 ) ;
#24553=EDGE_CURVE ( 'NONE', #12894, #32314, #19953, .T. ) ;
#24555=ORIENTED_EDGE ( 'NONE', *, *, #20971, .F. ) ;
#24558=ADVANCED_FACE ( 'NONE', ( #1767 ), #19484, .T. ) ;
#24561=CARTESIAN_POINT ( 'NONE',  ( -40.16174044770769314, 7.468546898574136783, 53.54930799450051637 ) ) ;
#24571=CARTESIAN_POINT ( 'NONE',  ( -40.70508238852950456, 9.491303552449114278, 34.64930799450052490 ) ) ;
#24577=AXIS2_PLACEMENT_3D ( 'NONE', #20988, #6382, #8525 ) ;
#24580=CARTESIAN_POINT ( 'NONE',  ( -40.90015969217747482, 8.955334253785162346, 57.95249952744806166 ) ) ;
#24583=DIRECTION ( 'NONE',  ( 0.4848096202463425541, 0.8746197071393929656, -2.220446049250313081E-16 ) ) ;
#24585=AXIS2_PLACEMENT_3D ( 'NONE', #8053, #18046, #27907 ) ;
#24586=DIRECTION ( 'NONE',  ( 0.2756373558169942228, -0.9612616959383203374, 0.000000000000000000 ) ) ;
#24588=EDGE_LOOP ( 'NONE', ( #17242, #32360, #2456, #6509 ) ) ;
#24591=ORIENTED_EDGE ( 'NONE', *, *, #27993, .T. ) ;
#24592=ADVANCED_FACE ( 'NONE', ( #6862 ), #26877, .T. ) ;
#24603=EDGE_CURVE ( 'NONE', #3439, #2858, #18888, .T. ) ;
#24608=ADVANCED_FACE ( 'NONE', ( #26710 ), #19151, .F. ) ;
#24609=AXIS2_PLACEMENT_3D ( 'NONE', #21542, #28784, #1053 ) ;
#24610=ORIENTED_EDGE ( 'NONE', *, *, #3519, .T. ) ;
#24615=DIRECTION ( 'NONE',  ( -7.588956326749211550E-18, 4.206627182996911684E-18, -1.000000000000000000 ) ) ;
#24624=FACE_OUTER_BOUND ( 'NONE', #24182, .T. ) ;
#24626=ORIENTED_EDGE ( 'NONE', *, *, #13391, .T. ) ;
#24629=ORIENTED_EDGE ( 'NONE', *, *, #4705, .F. ) ;
#24638=EDGE_CURVE ( 'NONE', #25249, #3392, #13497, .T. ) ;
#24655=FACE_OUTER_BOUND ( 'NONE', #30491, .T. ) ;
#24656=CARTESIAN_POINT ( 'NONE',  ( -42.21195563036362586, 4.051200314738734320, 55.04930799450051637 ) ) ;
#24659=CARTESIAN_POINT ( 'NONE',  ( -41.01929587258828036, 9.401204285752060130, 34.64930799450051779 ) ) ;
#24662=AXIS2_PLACEMENT_3D ( 'NONE', #27299, #1862, #9414 ) ;
#24663=DIRECTION ( 'NONE',  ( -0.8746197071393926326, 0.4848096202463430537, 8.676864087101709653E-18 ) ) ;
#24674=CARTESIAN_POINT ( 'NONE',  ( -40.11902961310586591, 6.880801488287907830, 39.52370399052030336 ) ) ;
#24682=ADVANCED_FACE ( 'NONE', ( #27690 ), #118, .T. ) ;
#24683=EDGE_CURVE ( 'NONE', #32232, #30206, #12645, .T. ) ;
#24685=ORIENTED_EDGE ( 'NONE', *, *, #5833, .T. ) ;
#24689=DIRECTION ( 'NONE',  ( 0.9612616959383198934, 0.2756373558169956106, 0.000000000000000000 ) ) ;
#24691=VERTEX_POINT ( 'NONE', #22599 ) ;
#24697=CARTESIAN_POINT ( 'NONE',  ( -40.76127908587941562, 8.436192945956459965, 34.55055826194723068 ) ) ;
#24699=LINE ( 'NONE', #2700, #22589 ) ;
#24709=DIRECTION ( 'NONE',  ( -0.4848096202462977566, -0.8746197071394176126, 0.000000000000000000 ) ) ;
#24713=AXIS2_PLACEMENT_3D ( 'NONE', #5643, #10745, #27974 ) ;
#24716=AXIS2_PLACEMENT_3D ( 'NONE', #17673, #22921, #7839 ) ;
#24724=EDGE_CURVE ( 'NONE', #3682, #7574, #32300, .T. ) ;
#24725=AXIS2_PLACEMENT_3D ( 'NONE', #11069, #13050, #30608 ) ;
#24726=TOROIDAL_SURFACE ( 'NONE', #22135, 0.8999999999999995781, 0.1000000000000000056 ) ;
#24729=ORIENTED_EDGE ( 'NONE', *, *, #11761, .T. ) ;
#24740=AXIS2_PLACEMENT_3D ( 'NONE', #6819, #9776, #16818 ) ;
#24744=CARTESIAN_POINT ( 'NONE',  ( -42.30123736278718383, 13.66041317296246937, 54.56265170360538264 ) ) ;
#24749=CARTESIAN_POINT ( 'NONE',  ( -40.06503689199327312, 6.934220188909110405, 34.98002959068131901 ) ) ;
#24751=ORIENTED_EDGE ( 'NONE', *, *, #23233, .F. ) ;
#24753=ORIENTED_EDGE ( 'NONE', *, *, #24983, .T. ) ;
#24754=AXIS2_PLACEMENT_3D ( 'NONE', #27071, #4583, #26584 ) ;
#24759=VERTEX_POINT ( 'NONE', #19804 ) ;
#24761=EDGE_CURVE ( 'NONE', #16834, #11074, #23638, .T. ) ;
#24762=ORIENTED_EDGE ( 'NONE', *, *, #25356, .F. ) ;
#24766=DIRECTION ( 'NONE',  ( -0.4848096202463430537, -0.8746197071393926326, -9.920727850371701658E-18 ) ) ;
#24777=LINE ( 'NONE', #19024, #4836 ) ;
#24779=CARTESIAN_POINT ( 'NONE',  ( -40.46704588662232283, 7.410332433786886774, 35.29983070667008604 ) ) ;
#24787=CARTESIAN_POINT ( 'NONE',  ( -41.24971778908466291, 11.62557032131817358, 57.04930799450051637 ) ) ;
#24797=CARTESIAN_POINT ( 'NONE',  ( -40.59758774925371938, 7.567737757495682338, 35.90717268343339441 ) ) ;
#24798=EDGE_CURVE ( 'NONE', #32074, #16648, #2132, .T. ) ;
#24799=EDGE_CURVE ( 'NONE', #10889, #7845, #10037, .T. ) ;
#24800=EDGE_CURVE ( 'NONE', #229, #25363, #16296, .T. ) ;
#24804=ADVANCED_FACE ( 'NONE', ( #14848 ), #11730, .T. ) ;
#24808=CARTESIAN_POINT ( 'NONE',  ( -40.40505316653322865, 8.317079188576503412, 54.54930799450051637 ) ) ;
#24815=DIRECTION ( 'NONE',  ( 0.000000000000000000, 0.000000000000000000, -1.000000000000000000 ) ) ;
#24816=FACE_OUTER_BOUND ( 'NONE', #27950, .T. ) ;
#24817=FACE_OUTER_BOUND ( 'NONE', #22087, .T. ) ;
#24819=FACE_OUTER_BOUND ( 'NONE', #22125, .T. ) ;
#24824=DIRECTION ( 'NONE',  ( 0.9612616959383194493, 0.2756373558169974980, 8.795445018804946186E-19 ) ) ;
#24825=LINE ( 'NONE', #22019, #5349 ) ;
#24827=ORIENTED_EDGE ( 'NONE', *, *, #27347, .F. ) ;
#24828=VERTEX_POINT ( 'NONE', #4829 ) ;
#24831=EDGE_CURVE ( 'NONE', #3679, #18639, #10327, .T. ) ;
#24839=ORIENTED_EDGE ( 'NONE', *, *, #13798, .T. ) ;
#24841=FACE_OUTER_BOUND ( 'NONE', #22291, .T. ) ;
#24851=ORIENTED_EDGE ( 'NONE', *, *, #11527, .F. ) ;
#24856=ORIENTED_EDGE ( 'NONE', *, *, #12546, .F. ) ;
#24860=AXIS2_PLACEMENT_3D ( 'NONE', #25501, #25973, #20728 ) ;
#24865=EDGE_CURVE ( 'NONE', #21395, #21286, #16800, .T. ) ;
#24882=ORIENTED_EDGE ( 'NONE', *, *, #30062, .T. ) ;
#24891=ADVANCED_FACE ( 'NONE', ( #31911 ), #24190, .F. ) ;
#24895=ORIENTED_EDGE ( 'NONE', *, *, #7815, .T. ) ;
#24896=LINE ( 'NONE', #19628, #24204 ) ;
#24898=LINE ( 'NONE', #24561, #3956 ) ;
#24903=ORIENTED_EDGE ( 'NONE', *, *, #4341, .F. ) ;
#24907=ORIENTED_EDGE ( 'NONE', *, *, #8459, .F. ) ;
#24910=DIRECTION ( 'NONE',  ( -0.4848096202463427762, -0.8746197071393926326, 0.000000000000000000 ) ) ;
#24911=DIRECTION ( 'NONE',  ( 0.9612616959383213366, 0.2756373558169906701, -3.016780184296941179E-15 ) ) ;
#24916=CARTESIAN_POINT ( 'NONE',  ( -40.46271621608484281, 3.081581074246047880, 37.04930799450052348 ) ) ;
#24917=DIRECTION ( 'NONE',  ( -0.4848096202463673121, -0.8746197071393789768, 0.000000000000000000 ) ) ;
#24919=ORIENTED_EDGE ( 'NONE', *, *, #17853, .F. ) ;
#24924=CIRCLE ( 'NONE', #19654, 0.1000000000000006301 ) ;
#24925=CIRCLE ( 'NONE', #21760, 1.300000000000002487 ) ;
#24926=FACE_BOUND ( 'NONE', #31865, .T. ) ;
#24929=ORIENTED_EDGE ( 'NONE', *, *, #6264, .F. ) ;
#24932=ADVANCED_FACE ( 'NONE', ( #1678, #24655 ), #17259, .T. ) ;
#24935=CIRCLE ( 'NONE', #10804, 1.524998423334080533 ) ;
#24946=ORIENTED_EDGE ( 'NONE', *, *, #4117, .F. ) ;
#24950=CARTESIAN_POINT ( 'NONE',  ( -40.68984688381691228, 6.797157182225290306, 34.72546689663558084 ) ) ;
#24952=CARTESIAN_POINT ( 'NONE',  ( -41.74033427429298371, 15.41509661078533355, 38.44930799450052206 ) ) ;
#24956=FACE_OUTER_BOUND ( 'NONE', #27483, .T. ) ;
#24957=DIRECTION ( 'NONE',  ( 0.9612616959383128989, 0.2756373558170196469, 0.000000000000000000 ) ) ;
#24962=COLOUR_RGB ( '',0.7921568627450980005, 0.8196078431372548767, 0.9333333333333333481 ) ;
#24974=CARTESIAN_POINT ( 'NONE',  ( -40.50048552624281939, 7.561504794674588581, 53.84930799450049932 ) ) ;
#24983=EDGE_CURVE ( 'NONE', #13414, #18622, #4139, .T. ) ;
#24995=FACE_OUTER_BOUND ( 'NONE', #28730, .T. ) ;
#24996=VERTEX_POINT ( 'NONE', #18071 ) ;
#24999=DIRECTION ( 'NONE',  ( 0.8746197071393927436, -0.4848096202463423876, -1.277302113040827440E-17 ) ) ;
#25002=CARTESIAN_POINT ( 'NONE',  ( -40.11264481937004689, 6.813248423021984301, 39.46181098083825844 ) ) ;
#25005=DIRECTION ( 'NONE',  ( -0.6797146636928631525, -0.1949050434465325332, -0.7071067811865497932 ) ) ;
#25008=EDGE_CURVE ( 'NONE', #21286, #29013, #21028, .T. ) ;
#25016=LINE ( 'NONE', #7787, #14962 ) ;
#25024=ORIENTED_EDGE ( 'NONE', *, *, #1393, .F. ) ;
#25027=LINE ( 'NONE', #14862, #3755 ) ;
#25030=CARTESIAN_POINT ( 'NONE',  ( -38.36853489569023168, 7.065850718397949315, 32.04930799450052348 ) ) ;
#25031=VERTEX_POINT ( 'NONE', #5607 ) ;
#25040=PRODUCT_DEFINITION_SHAPE ( 'NONE', 'NONE',  #8905 ) ;
#25041=LINE ( 'NONE', #2722, #1008 ) ;
#25049=AXIS2_PLACEMENT_3D ( 'NONE', #10224, #20223, #30247 ) ;
#25053=EDGE_LOOP ( 'NONE', ( #4089, #16310, #12163, #30873 ) ) ;
#25055=CARTESIAN_POINT ( 'NONE',  ( -40.60722745863126448, 9.415333058485023443, 34.69072935073783270 ) ) ;
#25060=ORIENTED_EDGE ( 'NONE', *, *, #24033, .F. ) ;
#25068=CARTESIAN_POINT ( 'NONE',  ( -42.26253548098706858, 13.64258395852576911, 54.54930799450051637 ) ) ;
#25069=CARTESIAN_POINT ( 'NONE',  ( -40.02540636251514172, 2.839176264122877047, 59.04930799450051637 ) ) ;
#25072=FACE_BOUND ( 'NONE', #743, .T. ) ;
#25074=ORIENTED_EDGE ( 'NONE', *, *, #20161, .F. ) ;
#25080=DIRECTION ( 'NONE',  ( -0.9612616959383200044, -0.2756373558169954996, 1.660411357259285896E-16 ) ) ;
#25084=ADVANCED_FACE ( 'NONE', ( #20050 ), #27604, .F. ) ;
#25087=ADVANCED_FACE ( 'NONE', ( #25144 ), #2659, .T. ) ;
#25092=EDGE_CURVE ( 'NONE', #23906, #1567, #12671, .T. ) ;
#25093=ORIENTED_EDGE ( 'NONE', *, *, #15358, .T. ) ;
#25096=ORIENTED_EDGE ( 'NONE', *, *, #19523, .T. ) ;
#25098=CYLINDRICAL_SURFACE ( 'NONE', #6763, 2.000000000000001776 ) ;
#25111=CARTESIAN_POINT ( 'NONE',  ( -42.38687957179149635, 4.148162238787999279, 37.04930799450052348 ) ) ;
#25113=EDGE_LOOP ( 'NONE', ( #8545, #1458, #25690 ) ) ;
#25115=CARTESIAN_POINT ( 'NONE',  ( -42.26497471389478733, 14.66834543456875117, 59.01654570186344984 ) ) ;
#25118=VERTEX_POINT ( 'NONE', #29016 ) ;
#25121=ORIENTED_EDGE ( 'NONE', *, *, #31216, .T. ) ;
#25130=EDGE_LOOP ( 'NONE', ( #25667, #3402, #20070, #29626, #12095, #12839, #6287, #9869, #24166, #17468, #10854, #29135, #1246, #11603 ) ) ;
#25132=ORIENTED_EDGE ( 'NONE', *, *, #9448, .F. ) ;
#25136=VERTEX_POINT ( 'NONE', #14085 ) ;
#25139=DIRECTION ( 'NONE',  ( 0.9612616959383128989, 0.2756373558170196469, 0.000000000000000000 ) ) ;
#25143=CARTESIAN_POINT ( 'NONE',  ( -40.50726673551752555, 7.559560314205212350, 60.26436683999078525 ) ) ;
#25144=FACE_OUTER_BOUND ( 'NONE', #15692, .T. ) ;
#25150=DIRECTION ( 'NONE',  ( 0.8746197071393926326, -0.4848096202463430537, -8.676864087101709653E-18 ) ) ;
#25153=AXIS2_PLACEMENT_3D ( 'NONE', #20228, #7605, #4646 ) ;
#25159=FACE_OUTER_BOUND ( 'NONE', #5401, .T. ) ;
#25162=EDGE_LOOP ( 'NONE', ( #15840, #16889, #23865, #26641 ) ) ;
#25180=AXIS2_PLACEMENT_3D ( 'NONE', #16115, #21516, #19214 ) ;
#25186=CARTESIAN_POINT ( 'NONE',  ( -40.18454328187963398, 7.548069831825862330, 53.80788663826320573 ) ) ;
#25187=( BOUNDED_CURVE ( )  B_SPLINE_CURVE ( 3, ( #24744, #21938, #25068, #22107 ),
 .UNSPECIFIED., .F., .F. ) 
 B_SPLINE_CURVE_WITH_KNOTS ( ( 4, 4 ),
 ( 4.189866217988888586, 4.712388980384689674 ),
 .UNSPECIFIED. ) 
 CURVE ( )  GEOMETRIC_REPRESENTATION_ITEM ( )  RATIONAL_B_SPLINE_CURVE ( ( 1.000000000000000000, 0.9773766218953335860, 0.9773766218953335860, 1.000000000000000000 ) ) 
 REPRESENTATION_ITEM ( '' )  );
#25190=EDGE_LOOP ( 'NONE', ( #10781, #8397, #16344 ) ) ;
#25198=DIRECTION ( 'NONE',  ( 2.779292025043186357E-18, -1.288349127009862211E-17, 1.000000000000000000 ) ) ;
#25211=VERTEX_POINT ( 'NONE', #3742 ) ;
#25225=AXIS2_PLACEMENT_3D ( 'NONE', #25826, #15973, #5976 ) ;
#25227=CLOSED_SHELL ( 'NONE', ( #6822, #26341, #3750, #29272, #22253, #6114, #26378, #26374, #12832, #9187, #411, #26794, #23392, #20402, #13819, #15353, #14641, #7907, #21600, #6671, #8048, #3704, #19141, #21031, #25571, #6230, #29442, #9631, #21631, #30279, #24198, #27307, #28812, #16485, #12670, #27522, #26835, #21148, #8015, #16151, #19360, #31026, #15300, #18176, #11859, #23166, #30767, #29313, #12954, #2202, #4437, #26271, #21042, #8645, #16989, #5268, #11235, #19857, #9835, #21847, #10319, #32440, #27807, #18286, #9217, #19428, #21880, #27258, #24269, #26338, #24932, #2375, #8597, #32076, #8342, #18079, #25800, #28538, #30632, #27581, #4257, #986, #10827, #8946, #16433, #16356, #2562, #26860, #2114, #32259, #789, #3767, #3246, #24345, #17080, #30143, #22257, #19209, #8892, #3929, #22158, #21629, #2842, #25087, #26707, #1472, #16338, #29692, #1021, #22858, #27617, #26655, #22156, #21074, #3002, #24592, #11170, #19518, #27219, #25280, #3375, #18835, #22819, #21849, #2331, #28714, #14392, #7071, #18250, #26008, #7635, #26980, #4114, #11476, #6638, #21387, #8461, #27199, #15755, #21843, #14951, #12496, #752, #30803, #24558, #4532, #28713, #1513, #19445, #20871, #20249, #3747, #25851, #19138, #19775, #24608, #3151, #17746, #18806, #8261, #29903, #2891, #14840, #10984, #29389, #5262, #28669, #24475, #26445, #10836, #13823, #16736, #5878, #31069, #9668, #8810, #22303, #7231, #22279, #25893, #28210, #301, #813, #25084, #4494, #28033, #23071, #21555, #9886, #17496, #31823, #26606, #4835, #18964, #1443, #30588, #14071, #26897, #21559, #17442, #2777, #21464, #2161, #10585, #27350, #31792, #16001, #20679, #20032, #24891, #22246, #1982, #11009, #3165, #7908, #30396, #8176, #27717, #22794, #16339, #5868, #10254, #11667, #5541, #30814, #23967, #23783, #17594, #12872, #2030, #7653, #5231, #20303, #784, #15903, #21510, #17374, #13664, #22784, #31718, #28902, #15757, #4403, #7620, #18373, #4052, #11311, #20300, #6517, #28489, #14485, #32027, #30261, #14498, #8818, #24682, #28509, #6751, #24804, #4526, #14578, #18066, #29987, #16399, #16414, #18656, #23267, #6371, #27614, #21839, #11965, #31863, #16374, #585, #6936 ) ) ;
#25229=ORIENTED_EDGE ( 'NONE', *, *, #24105, .F. ) ;
#25233=ORIENTED_EDGE ( 'NONE', *, *, #5833, .F. ) ;
#25240=DIRECTION ( 'NONE',  ( 0.000000000000000000, 0.000000000000000000, 1.000000000000000000 ) ) ;
#25243=DIRECTION ( 'NONE',  ( 0.8746197071393926326, -0.4848096202463430537, -8.676864087101709653E-18 ) ) ;
#25245=ORIENTED_EDGE ( 'NONE', *, *, #8385, .T. ) ;
#25246=VECTOR ( 'NONE', #7748, 1000.000000000000000 ) ;
#25249=VERTEX_POINT ( 'NONE', #2577 ) ;
#25251=DIRECTION ( 'NONE',  ( -0.6184495258776567805, 0.3428121700606641120, 0.7071067811865474617 ) ) ;
#25252=STYLED_ITEM('',(#32529),#1854);
#25253=ORIENTED_EDGE ( 'NONE', *, *, #21112, .F. ) ;
#25264=ORIENTED_EDGE ( 'NONE', *, *, #16842, .F. ) ;
#25272=CARTESIAN_POINT ( 'NONE',  ( -40.68642432603679282, 6.803331639905807471, 34.75772891228915285 ) ) ;
#25275=CARTESIAN_POINT ( 'NONE',  ( -40.47970302497625994, 7.463434137431151250, 60.44930799450051495 ) ) ;
#25278=VERTEX_POINT ( 'NONE', #22105 ) ;
#25280=ADVANCED_FACE ( 'NONE', ( #19971 ), #30001, .T. ) ;
#25297=SPHERICAL_SURFACE ( 'NONE', #3888, 0.1000000000000000056 ) ;
#25300=ORIENTED_EDGE ( 'NONE', *, *, #6772, .T. ) ;
#25307=CARTESIAN_POINT ( 'NONE',  ( -41.94956971822180947, 3.905757428664828890, 47.04930799450051637 ) ) ;
#25316=CARTESIAN_POINT ( 'NONE',  ( -40.02540636251513462, 2.839176264122873050, 37.04930799450052348 ) ) ;
#25320=EDGE_CURVE ( 'NONE', #27962, #32074, #9486, .T. ) ;
#25321=CARTESIAN_POINT ( 'NONE',  ( -39.44363481821952888, 3.888719912690147940, 57.04930799450051637 ) ) ;
#25329=LINE ( 'NONE', #25486, #27809 ) ;
#25336=CIRCLE ( 'NONE', #11696, 2.000000000000001776 ) ;
#25345=EDGE_LOOP ( 'NONE', ( #4948, #5804, #17593 ) ) ;
#25347=LINE ( 'NONE', #22877, #23052 ) ;
#25350=ORIENTED_EDGE ( 'NONE', *, *, #24831, .F. ) ;
#25352=DIRECTION ( 'NONE',  ( 0.2756373558169932236, -0.9612616959383204485, 1.479773560108267395E-16 ) ) ;
#25354=EDGE_CURVE ( 'NONE', #3682, #180, #14547, .T. ) ;
#25355=CARTESIAN_POINT ( 'NONE',  ( -37.49824857498671093, 12.70128680827697387, 56.14611646155296398 ) ) ;
#25356=EDGE_CURVE ( 'NONE', #19002, #16387, #23146, .T. ) ;
#25357=CIRCLE ( 'NONE', #6470, 0.1000000000000014905 ) ;
#25358=EDGE_CURVE ( 'NONE', #1567, #4768, #17922, .T. ) ;
#25359=DIRECTION ( 'NONE',  ( 7.588956326749211550E-18, -4.206627182996911684E-18, 1.000000000000000000 ) ) ;
#25363=VERTEX_POINT ( 'NONE', #5867 ) ;
#25370=DIRECTION ( 'NONE',  ( -0.7141240004913222972, 0.3958453973320028019, 0.5773502691896303940 ) ) ;
#25371=ORIENTED_EDGE ( 'NONE', *, *, #24553, .F. ) ;
#25374=DIRECTION ( 'NONE',  ( 0.8746197071393858602, -0.4848096202463547666, 0.000000000000000000 ) ) ;
#25379=CARTESIAN_POINT ( 'NONE',  ( -37.58300281841709989, 16.01180101885526597, 36.00717268343339583 ) ) ;
#25383=DIRECTION ( 'NONE',  ( 0.2756373558169974980, -0.9612616959383193382, 8.979771562518858393E-33 ) ) ;
#25392=EDGE_CURVE ( 'NONE', #21602, #18307, #7678, .T. ) ;
#25395=FACE_BOUND ( 'NONE', #11826, .T. ) ;
#25398=EDGE_CURVE ( 'NONE', #5228, #3250, #2725, .T. ) ;
#25401=ORIENTED_EDGE ( 'NONE', *, *, #3519, .F. ) ;
#25406=ORIENTED_EDGE ( 'NONE', *, *, #8139, .T. ) ;
#25413=ORIENTED_EDGE ( 'NONE', *, *, #17245, .F. ) ;
#25419=CARTESIAN_POINT ( 'NONE',  ( -42.50976151518963064, 14.59907569580870046, 37.04930799450052348 ) ) ;
#25420=DIRECTION ( 'NONE',  ( 0.9612616959383198934, 0.2756373558169956106, 0.000000000000000000 ) ) ;
#25425=CIRCLE ( 'NONE', #6053, 0.1000000000000013517 ) ;
#25427=TOROIDAL_SURFACE ( 'NONE', #15476, 1.899999999999999467, 0.1000000000000000056 ) ;
#25432=CARTESIAN_POINT ( 'NONE',  ( -40.21210701746133509, 7.644196001419694575, 53.64930799450051779 ) ) ;
#25437=CARTESIAN_POINT ( 'NONE',  ( -40.73091736380679606, 9.483895492497154578, 38.64930799450052490 ) ) ;
#25438=CARTESIAN_POINT ( 'NONE',  ( -40.69193635511749108, 9.347952559758585522, 39.44930799450052206 ) ) ;
#25445=CARTESIAN_POINT ( 'NONE',  ( -40.70484894842233103, 8.274204744976163539, 59.64930799450051779 ) ) ;
#25446=VECTOR ( 'NONE', #14605, 1000.000000000000227 ) ;
#25449=AXIS2_PLACEMENT_3D ( 'NONE', #6289, #876, #16294 ) ;
#25457=LINE ( 'NONE', #30713, #29363 ) ;
#25461=CARTESIAN_POINT ( 'NONE',  ( -40.16503835899720087, 7.510440877657817538, 35.29832907986742185 ) ) ;
#25466=LINE ( 'NONE', #18222, #22277 ) ;
#25467=FACE_OUTER_BOUND ( 'NONE', #30330, .T. ) ;
#25473=ORIENTED_EDGE ( 'NONE', *, *, #13246, .F. ) ;
#25474=LINE ( 'NONE', #21017, #12928 ) ;
#25479=CARTESIAN_POINT ( 'NONE',  ( -36.59542768321662720, 12.56771722797891400, 36.00717268343339583 ) ) ;
#25486=CARTESIAN_POINT ( 'NONE',  ( -40.61178118339597631, 9.038025460530262123, 57.95249952744806166 ) ) ;
#25501=CARTESIAN_POINT ( 'NONE',  ( -43.38408989745150990, 1.111547985471239786, 60.44930799450051495 ) ) ;
#25504=EDGE_LOOP ( 'NONE', ( #16350, #26034, #11544, #17275 ) ) ;
#25505=DIRECTION ( 'NONE',  ( 0.2756373558170082672, -0.9612616959383162296, 0.000000000000000000 ) ) ;
#25507=CARTESIAN_POINT ( 'NONE',  ( -39.67555847965937943, 2.645252416024336028, 48.24930799450051211 ) ) ;
#25509=CARTESIAN_POINT ( 'NONE',  ( -43.73393778030726509, 1.305471833569777695, 60.44930799450051495 ) ) ;
#25513=DIRECTION ( 'NONE',  ( 0.8746197071393926326, -0.4848096202463430537, -8.676864087101709653E-18 ) ) ;
#25528=EDGE_CURVE ( 'NONE', #7551, #28083, #31559, .T. ) ;
#25532=EDGE_CURVE ( 'NONE', #27995, #13414, #15324, .T. ) ;
#25538=EDGE_LOOP ( 'NONE', ( #30837, #23368, #21756, #18726 ) ) ;
#25540=CARTESIAN_POINT ( 'NONE',  ( -42.38687957179150345, 4.148162238788003719, 55.14930799450051779 ) ) ;
#25560=EDGE_LOOP ( 'NONE', ( #23102, #26610, #15815, #9386, #17906 ) ) ;
#25566=VECTOR ( 'NONE', #10106, 1000.000000000000114 ) ;
#25567=EDGE_CURVE ( 'NONE', #12604, #28083, #20545, .T. ) ;
#25571=ADVANCED_FACE ( 'NONE', ( #29964 ), #7144, .T. ) ;
#25580=VECTOR ( 'NONE', #24264, 1000.000000000000000 ) ;
#25585=DIRECTION ( 'NONE',  ( 0.8746197071393926326, -0.4848096202463430537, -8.676864087101709653E-18 ) ) ;
#25586=CARTESIAN_POINT ( 'NONE',  ( -40.05987053574653345, 7.506472619680471858, 35.39279590939684539 ) ) ;
#25590=DIRECTION ( 'NONE',  ( 0.8746197071393925215, -0.4848096202463429982, -8.676864087101708112E-18 ) ) ;
#25592=ORIENTED_EDGE ( 'NONE', *, *, #10034, .T. ) ;
#25594=CARTESIAN_POINT ( 'NONE',  ( -40.65487266620045403, 9.475231293617264683, 38.63717596014456035 ) ) ;
#25605=AXIS2_PLACEMENT_3D ( 'NONE', #26079, #23626, #28882 ) ;
#25614=CARTESIAN_POINT ( 'NONE',  ( -42.38687957179149635, 4.148162238787999279, 35.74930799450051921 ) ) ;
#25619=CYLINDRICAL_SURFACE ( 'NONE', #6203, 0.1000000000000014905 ) ;
#25623=DIRECTION ( 'NONE',  ( -0.2756373558169973870, 0.9612616959383193382, -9.615507602343155278E-33 ) ) ;
#25632=DIRECTION ( 'NONE',  ( -0.1949050434465268433, 0.6797146636928677044, 0.7071067811865471286 ) ) ;
#25635=AXIS2_PLACEMENT_3D ( 'NONE', #10920, #27834, #7979 ) ;
#25637=EDGE_LOOP ( 'NONE', ( #24762, #16341, #23181 ) ) ;
#25647=CIRCLE ( 'NONE', #31409, 0.1000000000000001305 ) ;
#25657=CYLINDRICAL_SURFACE ( 'NONE', #10080, 0.1000000000000004774 ) ;
#25658=VECTOR ( 'NONE', #12206, 1000.000000000000114 ) ;
#25659=ORIENTED_EDGE ( 'NONE', *, *, #29399, .T. ) ;
#25660=AXIS2_PLACEMENT_3D ( 'NONE', #28629, #6141, #23222 ) ;
#25665=PLANE ( 'NONE',  #25225 ) ;
#25666=DIRECTION ( 'NONE',  ( 0.9612616959383193382, 0.2756373558169973870, 8.795445018804928853E-19 ) ) ;
#25667=ORIENTED_EDGE ( 'NONE', *, *, #15084, .T. ) ;
#25671=EDGE_CURVE ( 'NONE', #1905, #2732, #11650, .T. ) ;
#25675=CARTESIAN_POINT ( 'NONE',  ( -40.70335362822509495, 9.387769322903325886, 39.54930799450052348 ) ) ;
#25677=CYLINDRICAL_SURFACE ( 'NONE', #9620, 0.1000000000000018235 ) ;
#25680=DIRECTION ( 'NONE',  ( -1.188208965918165239E-16, -1.880121038077813132E-16, -1.000000000000000000 ) ) ;
#25683=AXIS2_PLACEMENT_3D ( 'NONE', #8429, #21044, #16121 ) ;
#25684=EDGE_CURVE ( 'NONE', #14105, #27032, #9280, .T. ) ;
#25689=DIRECTION ( 'NONE',  ( -0.3428121700606640565, -0.6184495258776567805, -0.7071067811865474617 ) ) ;
#25690=ORIENTED_EDGE ( 'NONE', *, *, #30035, .F. ) ;
#25696=EDGE_CURVE ( 'NONE', #14804, #1265, #21590, .T. ) ;
#25704=ORIENTED_EDGE ( 'NONE', *, *, #1336, .T. ) ;
#25706=CARTESIAN_POINT ( 'NONE',  ( -41.91739890389096956, 13.90674392281398930, 59.49868301348410426 ) ) ;
#25715=DIRECTION ( 'NONE',  ( 0.8746197071393925215, -0.4848096202463429982, -8.676864087101708112E-18 ) ) ;
#25718=EDGE_CURVE ( 'NONE', #10826, #24287, #25791, .T. ) ;
#25736=EDGE_LOOP ( 'NONE', ( #4885, #20405, #12919, #8491 ) ) ;
#25737=VECTOR ( 'NONE', #12937, 1000.000000000000114 ) ;
#25738=VERTEX_POINT ( 'NONE', #13218 ) ;
#25740=DIRECTION ( 'NONE',  ( 0.1949050434465251780, -0.6797146636928681485, -0.7071067811865470176 ) ) ;
#25742=EDGE_LOOP ( 'NONE', ( #22822, #15141, #18895, #10431 ) ) ;
#25750=AXIS2_PLACEMENT_3D ( 'NONE', #14325, #24163, #29423 ) ;
#25751=ORIENTED_EDGE ( 'NONE', *, *, #9139, .F. ) ;
#25753=LINE ( 'NONE', #20821, #18496 ) ;
#25757=CARTESIAN_POINT ( 'NONE',  ( -40.11286833322907341, 2.887657226147505973, 39.04930799450052348 ) ) ;
#25760=EDGE_CURVE ( 'NONE', #382, #26808, #26125, .T. ) ;
#25765=CARTESIAN_POINT ( 'NONE',  ( -41.91799733298573472, 13.87669230940966969, 59.51428496617474195 ) ) ;
#25770=CARTESIAN_POINT ( 'NONE',  ( -40.23847960489091236, 6.935107575317838169, 39.54930799450052348 ) ) ;
#25775=CIRCLE ( 'NONE', #11638, 0.09999999999999939493 ) ;
#25778=DIRECTION ( 'NONE',  ( -0.2756373558169905591, 0.9612616959383213366, -2.072800435186483623E-19 ) ) ;
#25780=LINE ( 'NONE', #21321, #28692 ) ;
#25785=FACE_OUTER_BOUND ( 'NONE', #1345, .T. ) ;
#25791=CIRCLE ( 'NONE', #29999, 2.000000000000001776 ) ;
#25798=CARTESIAN_POINT ( 'NONE',  ( -40.02540636251514172, 2.839176264122877047, 58.24930799450051921 ) ) ;
#25800=ADVANCED_FACE ( 'NONE', ( #5650 ), #10593, .F. ) ;
#25808=CIRCLE ( 'NONE', #15848, 0.2000000000000012601 ) ;
#25812=ORIENTED_EDGE ( 'NONE', *, *, #776, .F. ) ;
#25823=SPHERICAL_SURFACE ( 'NONE', #11534, 0.1000000000000000056 ) ;
#25825=VECTOR ( 'NONE', #8652, 1000.000000000000000 ) ;
#25826=CARTESIAN_POINT ( 'NONE',  ( -39.31817303416427478, 4.733858564475564634, 57.04930799450051637 ) ) ;
#25827=VERTEX_POINT ( 'NONE', #20584 ) ;
#25829=DIRECTION ( 'NONE',  ( 0.8746197071393926326, -0.4848096202463430537, -8.676864087101709653E-18 ) ) ;
#25832=CARTESIAN_POINT ( 'NONE',  ( -40.46704588662232993, 7.410332433786888551, 38.79878528233096091 ) ) ;
#25833=EDGE_LOOP ( 'NONE', ( #6511, #7471, #11760, #31404 ) ) ;
#25834=DIRECTION ( 'NONE',  ( 0.1949050434465282311, -0.6797146636928674823, -0.7071067811865470176 ) ) ;
#25839=CARTESIAN_POINT ( 'NONE',  ( -40.06561427811386267, 7.496110634155836117, 56.04611646155296256 ) ) ;
#25844=CARTESIAN_POINT ( 'NONE',  ( -40.61574147496727960, 7.605736927813758541, 60.17502049423573851 ) ) ;
#25845=ORIENTED_EDGE ( 'NONE', *, *, #19481, .F. ) ;
#25850=EDGE_CURVE ( 'NONE', #19852, #4736, #7246, .T. ) ;
#25851=ADVANCED_FACE ( 'NONE', ( #5340 ), #20743, .F. ) ;
#25858=DIRECTION ( 'NONE',  ( -1.188208965918165239E-16, -1.880121038077813132E-16, -1.000000000000000000 ) ) ;
#25863=FACE_OUTER_BOUND ( 'NONE', #5567, .T. ) ;
#25875=DIRECTION ( 'NONE',  ( 0.8746197071393926326, -0.4848096202463430537, -8.676864087101709653E-18 ) ) ;
#25878=VECTOR ( 'NONE', #27302, 1000.000000000000114 ) ;
#25882=DIRECTION ( 'NONE',  ( 0.9612616959383193382, 0.2756373558169973870, 8.795445018804928853E-19 ) ) ;
#25887=FACE_OUTER_BOUND ( 'NONE', #24545, .T. ) ;
#25893=ADVANCED_FACE ( 'NONE', ( #31089 ), #25986, .T. ) ;
#25894=AXIS2_PLACEMENT_3D ( 'NONE', #19279, #26681, #4200 ) ;
#25900=FACE_OUTER_BOUND ( 'NONE', #1622, .T. ) ;
#25901=FACE_OUTER_BOUND ( 'NONE', #30161, .T. ) ;
#25911=CARTESIAN_POINT ( 'NONE',  ( -40.11286833322908052, 2.887657226147511302, 55.14930799450051779 ) ) ;
#25912=AXIS2_PLACEMENT_3D ( 'NONE', #23076, #30312, #8307 ) ;
#25916=DIRECTION ( 'NONE',  ( 0.8746197071393926326, -0.4848096202463430537, -8.676864087101709653E-18 ) ) ;
#25921=CARTESIAN_POINT ( 'NONE',  ( -40.50746472795130870, 7.570599710249083181, 53.85997431717469652 ) ) ;
#25925=AXIS2_PLACEMENT_3D ( 'NONE', #1799, #14286, #21317 ) ;
#25926=EDGE_LOOP ( 'NONE', ( #20904, #31607, #8626, #10265, #17689 ) ) ;
#25928=CARTESIAN_POINT ( 'NONE',  ( -36.21250238186772208, 8.895094119121829124, 60.29072935073781991 ) ) ;
#25930=VECTOR ( 'NONE', #20694, 1000.000000000000114 ) ;
#25934=VERTEX_POINT ( 'NONE', #23371 ) ;
#25936=DIRECTION ( 'NONE',  ( 0.9612616959383221138, 0.2756373558169876170, 0.000000000000000000 ) ) ;
#25947=CYLINDRICAL_SURFACE ( 'NONE', #16550, 0.1000000000000028644 ) ;
#25950=VECTOR ( 'NONE', #27227, 1000.000000000000000 ) ;
#25952=DIRECTION ( 'NONE',  ( 0.8746197071393926326, -0.4848096202463430537, -8.676864087101709653E-18 ) ) ;
#25955=ORIENTED_EDGE ( 'NONE', *, *, #20116, .F. ) ;
#25965=PLANE ( 'NONE',  #26974 ) ;
#25968=EDGE_LOOP ( 'NONE', ( #13430, #14916, #5391, #28807 ) ) ;
#25972=EDGE_CURVE ( 'NONE', #30053, #18805, #4688, .T. ) ;
#25973=DIRECTION ( 'NONE',  ( -2.779292025043186357E-18, 1.288349127009862211E-17, -1.000000000000000000 ) ) ;
#25983=ORIENTED_EDGE ( 'NONE', *, *, #28399, .T. ) ;
#25986=PLANE ( 'NONE',  #22440 ) ;
#25995=DIRECTION ( 'NONE',  ( 0.2756373558169932236, -0.9612616959383206705, 1.479773560108267395E-16 ) ) ;
#26002=EDGE_CURVE ( 'NONE', #25278, #17298, #32057, .T. ) ;
#26005=ORIENTED_EDGE ( 'NONE', *, *, #10803, .F. ) ;
#26008=ADVANCED_FACE ( 'NONE', ( #14334 ), #9402, .T. ) ;
#26010=CARTESIAN_POINT ( 'NONE',  ( -40.59581018552366061, 9.375516295340281303, 34.64930799450051779 ) ) ;
#26013=FACE_OUTER_BOUND ( 'NONE', #8495, .T. ) ;
#26021=ORIENTED_EDGE ( 'NONE', *, *, #25567, .F. ) ;
#26026=DIRECTION ( 'NONE',  ( 0.000000000000000000, 0.000000000000000000, 1.000000000000000000 ) ) ;
#26027=CARTESIAN_POINT ( 'NONE',  ( -40.12608762486730996, 7.344210729236881008, 60.41996114768177506 ) ) ;
#26028=FACE_OUTER_BOUND ( 'NONE', #12046, .T. ) ;
#26029=FACE_OUTER_BOUND ( 'NONE', #25162, .T. ) ;
#26034=ORIENTED_EDGE ( 'NONE', *, *, #11767, .T. ) ;
#26035=CARTESIAN_POINT ( 'NONE',  ( -40.68422973805265030, 6.807290781432338456, 34.77612644482307758 ) ) ;
#26040=( BOUNDED_CURVE ( )  B_SPLINE_CURVE ( 3, ( #8728, #21508, #24144, #11199 ),
 .UNSPECIFIED., .F., .F. ) 
 B_SPLINE_CURVE_WITH_KNOTS ( ( 4, 4 ),
 ( 4.712388980384687009, 6.283185307179586232 ),
 .UNSPECIFIED. ) 
 CURVE ( )  GEOMETRIC_REPRESENTATION_ITEM ( )  RATIONAL_B_SPLINE_CURVE ( ( 1.000000000000000000, 0.8047378541243643824, 0.8047378541243643824, 1.000000000000000000 ) ) 
 REPRESENTATION_ITEM ( '' )  );
#26047=ORIENTED_EDGE ( 'NONE', *, *, #482, .T. ) ;
#26071=AXIS2_PLACEMENT_3D ( 'NONE', #1936, #27049, #31814 ) ;
#26074=CARTESIAN_POINT ( 'NONE',  ( -40.39697993529618003, 8.288924485351975235, 54.52001867261917312 ) ) ;
#26079=CARTESIAN_POINT ( 'NONE',  ( -40.23672901771082877, 7.760455916344221272, 39.54930799450052348 ) ) ;
#26095=FACE_OUTER_BOUND ( 'NONE', #2341, .T. ) ;
#26096=DIRECTION ( 'NONE',  ( 0.4848096202463673676, 0.8746197071393789768, 0.000000000000000000 ) ) ;
#26097=ORIENTED_EDGE ( 'NONE', *, *, #13229, .T. ) ;
#26101=VECTOR ( 'NONE', #11697, 1000.000000000000114 ) ;
#26103=LINE ( 'NONE', #8236, #9563 ) ;
#26104=DIRECTION ( 'NONE',  ( 0.8746197071393926326, -0.4848096202463430537, -8.676864087101709653E-18 ) ) ;
#26111=EDGE_CURVE ( 'NONE', #13529, #18870, #20706, .T. ) ;
#26112=DIRECTION ( 'NONE',  ( 0.2756373558169974980, -0.9612616959383193382, -1.315048337272770589E-17 ) ) ;
#26116=ORIENTED_EDGE ( 'NONE', *, *, #9719, .T. ) ;
#26120=CIRCLE ( 'NONE', #21388, 0.7928932188134565351 ) ;
#26125=CIRCLE ( 'NONE', #11973, 1.042135311067126979 ) ;
#26129=ORIENTED_EDGE ( 'NONE', *, *, #31274, .T. ) ;
#26135=DIRECTION ( 'NONE',  ( -0.9612616959383186721, -0.2756373558169996629, -8.795445018805237002E-19 ) ) ;
#26141=DIRECTION ( 'NONE',  ( 0.9097384655268496711, 0.4151817967359032746, -1.524080105319609646E-17 ) ) ;
#26144=CARTESIAN_POINT ( 'NONE',  ( -40.58095149058966200, 7.465239395913044973, 60.18771704643254594 ) ) ;
#26145=EDGE_LOOP ( 'NONE', ( #20102, #8775, #12768, #24469, #27970 ) ) ;
#26148=CARTESIAN_POINT ( 'NONE',  ( -40.38516919650994197, 8.640923867788874446, 34.64930799450051779 ) ) ;
#26156=EDGE_LOOP ( 'NONE', ( #26809, #26759, #9833, #27565 ) ) ;
#26157=CARTESIAN_POINT ( 'NONE',  ( -40.66586793973302605, 8.138261812237592707, 59.50788663826320146 ) ) ;
#26162=EDGE_CURVE ( 'NONE', #1265, #11047, #30246, .T. ) ;
#26165=CARTESIAN_POINT ( 'NONE',  ( -41.07560527903737579, 9.385057823277968225, 39.44930799450052206 ) ) ;
#26166=ORIENTED_EDGE ( 'NONE', *, *, #23846, .F. ) ;
#26175=CARTESIAN_POINT ( 'NONE',  ( -41.09927805198056916, 10.76852187697755880, 36.12712545380572493 ) ) ;
#26176=ORIENTED_EDGE ( 'NONE', *, *, #24199, .F. ) ;
#26179=CARTESIAN_POINT ( 'NONE',  ( -42.67312000749024747, 15.16877446138198238, 38.54930799450052348 ) ) ;
#26180=ORIENTED_EDGE ( 'NONE', *, *, #18961, .F. ) ;
#26181=FACE_OUTER_BOUND ( 'NONE', #20472, .T. ) ;
#26190=DIRECTION ( 'NONE',  ( 0.2072038891212098777, -0.4540212254542328463, 0.8665629089512670857 ) ) ;
#26195=CARTESIAN_POINT ( 'NONE',  ( -40.55769077061455619, 7.370228602978611043, 35.39483402557622327 ) ) ;
#26199=AXIS2_PLACEMENT_3D ( 'NONE', #29766, #7452, #4818 ) ;
#26200=CARTESIAN_POINT ( 'NONE',  ( -41.50472230201275892, 5.945882615091422352, 57.04930799450051637 ) ) ;
#26202=EDGE_CURVE ( 'NONE', #8364, #16525, #2558, .T. ) ;
#26204=EDGE_CURVE ( 'NONE', #11711, #12276, #5780, .T. ) ;
#26205=AXIS2_PLACEMENT_3D ( 'NONE', #8433, #23522, #23835 ) ;
#26206=ORIENTED_EDGE ( 'NONE', *, *, #17195, .T. ) ;
#26209=AXIS2_PLACEMENT_3D ( 'NONE', #31497, #26725, #18999 ) ;
#26210=ORIENTED_EDGE ( 'NONE', *, *, #4571, .T. ) ;
#26213=DIRECTION ( 'NONE',  ( 0.000000000000000000, 0.000000000000000000, 1.000000000000000000 ) ) ;
#26216=EDGE_LOOP ( 'NONE', ( #28242, #26176, #30254, #11401 ) ) ;
#26230=DIRECTION ( 'NONE',  ( -0.4848096202463368365, -0.8746197071393959632, 0.000000000000000000 ) ) ;
#26231=CARTESIAN_POINT ( 'NONE',  ( -40.55769077061466987, 7.370228602979226551, 38.70378196342478105 ) ) ;
#26235=DIRECTION ( 'NONE',  ( -0.2756373558170082672, 0.9612616959383162296, 0.000000000000000000 ) ) ;
#26240=AXIS2_PLACEMENT_3D ( 'NONE', #2971, #30883, #20539 ) ;
#26241=FACE_OUTER_BOUND ( 'NONE', #5739, .T. ) ;
#26244=ORIENTED_EDGE ( 'NONE', *, *, #25358, .F. ) ;
#26245=FACE_OUTER_BOUND ( 'NONE', #22774, .T. ) ;
#26253=VECTOR ( 'NONE', #16168, 1000.000000000000000 ) ;
#26255=B_SPLINE_CURVE_WITH_KNOTS ( 'NONE', 3,
 ( #12715, #14455, #22636, #19846, #156, #2134, #15096, #24779, #9846, #2295 ),
 .UNSPECIFIED., .F., .F.,
 ( 4, 2, 2, 2, 4 ),
 ( 2.968785590477208419E-05, 0.0003298221638443240276, 0.0006299564717838759473, 0.0009300907797234278128, 0.001230225087662979678 ),
 .UNSPECIFIED. ) ;
#26271=ADVANCED_FACE ( 'NONE', ( #3307 ), #21941, .T. ) ;
#26273=DIRECTION ( 'NONE',  ( 0.8746197071393926326, -0.4848096202463430537, -8.676864087101709653E-18 ) ) ;
#26277=ORIENTED_EDGE ( 'NONE', *, *, #14948, .F. ) ;
#26284=DIRECTION ( 'NONE',  ( 0.9612616959383206705, 0.2756373558169926130, 8.795445018804289444E-19 ) ) ;
#26286=VERTEX_POINT ( 'NONE', #16096 ) ;
#26295=DIRECTION ( 'NONE',  ( 0.000000000000000000, 0.000000000000000000, -1.000000000000000000 ) ) ;
#26298=EDGE_CURVE ( 'NONE', #21636, #12799, #8719, .T. ) ;
#26303=FACE_OUTER_BOUND ( 'NONE', #25345, .T. ) ;
#26307=EDGE_CURVE ( 'NONE', #28686, #23334, #32439, .T. ) ;
#26312=DIRECTION ( 'NONE',  ( 0.2756373558169938898, -0.9612616959383203374, 0.000000000000000000 ) ) ;
#26314=CARTESIAN_POINT ( 'NONE',  ( -42.59587854516874472, -0.7667456371672803916, 32.14930799450051779 ) ) ;
#26315=AXIS2_PLACEMENT_3D ( 'NONE', #27728, #472, #30356 ) ;
#26333=VECTOR ( 'NONE', #15057, 1000.000000000000000 ) ;
#26338=ADVANCED_FACE ( 'NONE', ( #9534 ), #1651, .F. ) ;
#26339=ORIENTED_EDGE ( 'NONE', *, *, #1138, .T. ) ;
#26341=ADVANCED_FACE ( 'NONE', ( #31851 ), #26925, .T. ) ;
#26343=CARTESIAN_POINT ( 'NONE',  ( -39.58809650894544774, 2.596771453999702661, 47.04930799450051637 ) ) ;
#26344=LINE ( 'NONE', #29137, #26253 ) ;
#26350=EDGE_LOOP ( 'NONE', ( #8376, #26442, #23796, #17042 ) ) ;
#26354=FACE_OUTER_BOUND ( 'NONE', #29215, .T. ) ;
#26355=CIRCLE ( 'NONE', #30566, 0.1000000000000012962 ) ;
#26358=CARTESIAN_POINT ( 'NONE',  ( -40.13646513110857938, 7.213257191582266969, 35.13906202186969097 ) ) ;
#26359=CARTESIAN_POINT ( 'NONE',  ( -40.50410981870283678, 7.604537000166495808, 35.33853321918559942 ) ) ;
#26360=AXIS2_PLACEMENT_3D ( 'NONE', #4543, #19474, #17166 ) ;
#26361=ORIENTED_EDGE ( 'NONE', *, *, #12988, .F. ) ;
#26364=ORIENTED_EDGE ( 'NONE', *, *, #22654, .F. ) ;
#26366=AXIS2_PLACEMENT_3D ( 'NONE', #9162, #16865, #9493 ) ;
#26367=VERTEX_POINT ( 'NONE', #29560 ) ;
#26368=ORIENTED_EDGE ( 'NONE', *, *, #13205, .F. ) ;
#26371=VERTEX_POINT ( 'NONE', #4771 ) ;
#26373=FACE_OUTER_BOUND ( 'NONE', #15908, .T. ) ;
#26374=ADVANCED_FACE ( 'NONE', ( #1814 ), #7814, .F. ) ;
#26378=ADVANCED_FACE ( 'NONE', ( #24624 ), #19317, .F. ) ;
#26386=EDGE_CURVE ( 'NONE', #23253, #9190, #2305, .T. ) ;
#26387=EDGE_CURVE ( 'NONE', #2410, #7171, #26595, .T. ) ;
#26389=VERTEX_POINT ( 'NONE', #17067 ) ;
#26390=EDGE_LOOP ( 'NONE', ( #23483, #10450, #29346, #9332 ) ) ;
#26402=FACE_OUTER_BOUND ( 'NONE', #9000, .T. ) ;
#26404=CIRCLE ( 'NONE', #18017, 0.09999999999999795164 ) ;
#26410=CARTESIAN_POINT ( 'NONE',  ( -40.58856461370174173, 7.499380836222963254, 53.94930799450051495 ) ) ;
#26415=CYLINDRICAL_SURFACE ( 'NONE', #17030, 0.1000000000000018235 ) ;
#26416=DIRECTION ( 'NONE',  ( 0.2756373558169947779, -0.9612616959383200044, 0.000000000000000000 ) ) ;
#26419=AXIS2_PLACEMENT_3D ( 'NONE', #14483, #4956, #24477 ) ;
#26426=ORIENTED_EDGE ( 'NONE', *, *, #1110, .T. ) ;
#26427=DIRECTION ( 'NONE',  ( 0.000000000000000000, 0.000000000000000000, 1.000000000000000000 ) ) ;
#26436=DIRECTION ( 'NONE',  ( 0.2756373558169941118, -0.9612616959383204485, -1.315048337272770897E-17 ) ) ;
#26442=ORIENTED_EDGE ( 'NONE', *, *, #12500, .T. ) ;
#26443=CARTESIAN_POINT ( 'NONE',  ( -40.50764110105879467, 7.565280838256598805, 60.25772877010867745 ) ) ;
#26445=ADVANCED_FACE ( 'NONE', ( #6738 ), #11994, .F. ) ;
#26448=CIRCLE ( 'NONE', #16483, 0.1000000000000014905 ) ;
#26449=EDGE_CURVE ( 'NONE', #8640, #32001, #6907, .T. ) ;
#26453=AXIS2_PLACEMENT_3D ( 'NONE', #17867, #15406, #28528 ) ;
#26457=FACE_OUTER_BOUND ( 'NONE', #25637, .T. ) ;
#26463=CARTESIAN_POINT ( 'NONE',  ( -40.76199410932685652, 8.110698076655891597, 54.59072935073782418 ) ) ;
#26465=CARTESIAN_POINT ( 'NONE',  ( -40.51522877113607990, 7.610537050327680575, 53.90050461276381100 ) ) ;
#26466=CARTESIAN_POINT ( 'NONE',  ( -40.11598084786749752, 7.671759737001393908, 53.80788663826320573 ) ) ;
#26469=VECTOR ( 'NONE', #23161, 1000.000000000000000 ) ;
#26472=ORIENTED_EDGE ( 'NONE', *, *, #32315, .F. ) ;
#26473=CARTESIAN_POINT ( 'NONE',  ( -40.59290754354907449, 7.518856927436786464, 53.97121855808759250 ) ) ;
#26477=AXIS2_PLACEMENT_3D ( 'NONE', #10888, #20881, #28445 ) ;
#26481=CARTESIAN_POINT ( 'NONE',  ( -40.18117225532236603, 7.056010640735439488, 39.15497037975539740 ) ) ;
#26483=EDGE_CURVE ( 'NONE', #29567, #26975, #11455, .T. ) ;
#26486=DIRECTION ( 'NONE',  ( 0.1949050434465282311, -0.6797146636928673713, -0.7071067811865467956 ) ) ;
#26493=ORIENTED_EDGE ( 'NONE', *, *, #23838, .F. ) ;
#26507=CARTESIAN_POINT ( 'NONE',  ( -43.38408989745150990, 1.111547985471240674, 53.64930799450051779 ) ) ;
#26514=B_SPLINE_CURVE_WITH_KNOTS ( 'NONE', 3,
 ( #18571, #16755, #16594, #23986, #1669, #4296, #1500, #11516 ),
 .UNSPECIFIED., .F., .F.,
 ( 4, 2, 2, 4 ),
 ( 0.000000000000000000, 0.0005357332384296896628, 0.0008035998576445335185, 0.001071466476859377374 ),
 .UNSPECIFIED. ) ;
#26533=EDGE_CURVE ( 'NONE', #21772, #19940, #9266, .T. ) ;
#26534=VECTOR ( 'NONE', #17293, 1000.000000000000114 ) ;
#26536=FACE_OUTER_BOUND ( 'NONE', #1010, .T. ) ;
#26543=FACE_OUTER_BOUND ( 'NONE', #29873, .T. ) ;
#26569=EDGE_CURVE ( 'NONE', #11074, #28974, #30823, .T. ) ;
#26580=LINE ( 'NONE', #4266, #18582 ) ;
#26581=CARTESIAN_POINT ( 'NONE',  ( -40.01416947921579492, 7.179266651195999493, 38.85693688870069451 ) ) ;
#26583=EDGE_LOOP ( 'NONE', ( #7325, #27824, #27268, #17129 ) ) ;
#26584=DIRECTION ( 'NONE',  ( -0.4848096202463655358, -0.8746197071393799760, 0.000000000000000000 ) ) ;
#26594=CARTESIAN_POINT ( 'NONE',  ( -39.59300248568538194, 7.744584186742828891, 61.94930799450052206 ) ) ;
#26595=LINE ( 'NONE', #9039, #18766 ) ;
#26603=EDGE_CURVE ( 'NONE', #10451, #22848, #1446, .T. ) ;
#26606=ADVANCED_FACE ( 'NONE', ( #23135, #26241 ), #28388, .F. ) ;
#26610=ORIENTED_EDGE ( 'NONE', *, *, #30543, .T. ) ;
#26613=LINE ( 'NONE', #1990, #11766 ) ;
#26614=DIRECTION ( 'NONE',  ( 0.000000000000000000, 0.000000000000000000, -1.000000000000000000 ) ) ;
#26618=CARTESIAN_POINT ( 'NONE',  ( -40.70484894842233103, 8.274204744976163539, 54.44930799450051495 ) ) ;
#26626=VERTEX_POINT ( 'NONE', #25757 ) ;
#26631=EDGE_CURVE ( 'NONE', #31093, #25031, #3590, .T. ) ;
#26632=AXIS2_PLACEMENT_3D ( 'NONE', #16671, #16841, #13914 ) ;
#26634=CARTESIAN_POINT ( 'NONE',  ( -43.69495677161796010, 1.169528900831203311, 60.54930799450051637 ) ) ;
#26635=AXIS2_PLACEMENT_3D ( 'NONE', #9737, #12367, #1685 ) ;
#26636=ORIENTED_EDGE ( 'NONE', *, *, #22403, .T. ) ;
#26640=VECTOR ( 'NONE', #11754, 1000.000000000000000 ) ;
#26641=ORIENTED_EDGE ( 'NONE', *, *, #25850, .F. ) ;
#26643=CARTESIAN_POINT ( 'NONE',  ( -38.32955388700093380, 6.929907785659375818, 32.14930799450051779 ) ) ;
#26644=DIRECTION ( 'NONE',  ( -2.946248497964555786E-19, -3.001156285468303092E-19, -1.000000000000000000 ) ) ;
#26647=EDGE_LOOP ( 'NONE', ( #11393, #29509, #16538, #27163 ) ) ;
#26648=CARTESIAN_POINT ( 'NONE',  ( -40.60922101150776342, 7.585765375989710790, 60.19601566531913051 ) ) ;
#26655=ADVANCED_FACE ( 'NONE', ( #23771 ), #11154, .T. ) ;
#26668=DIRECTION ( 'NONE',  ( 0.8746197071393926326, -0.4848096202463430537, -8.676864087101709653E-18 ) ) ;
#26670=CARTESIAN_POINT ( 'NONE',  ( -41.02113223168485234, 7.230835263863472306, 39.54930799450052348 ) ) ;
#26675=CARTESIAN_POINT ( 'NONE',  ( -48.24907229644473716, 10.92050229712533316, 54.54930799450051637 ) ) ;
#26680=CARTESIAN_POINT ( 'NONE',  ( -40.01678386995647685, 7.136726190597861397, 35.21344202038847726 ) ) ;
#26681=DIRECTION ( 'NONE',  ( 0.2756373558169932236, -0.9612616959383205595, 1.479773560108267395E-16 ) ) ;
#26684=AXIS2_PLACEMENT_3D ( 'NONE', #8508, #20810, #10662 ) ;
#26686=LINE ( 'NONE', #31619, #32141 ) ;
#26688=ORIENTED_EDGE ( 'NONE', *, *, #10733, .F. ) ;
#26689=EDGE_CURVE ( 'NONE', #3106, #21227, #18798, .T. ) ;
#26701=CARTESIAN_POINT ( 'NONE',  ( -40.50755597040444655, 7.564707434449536194, 53.84113122998387979 ) ) ;
#26704=CARTESIAN_POINT ( 'NONE',  ( -40.52510752649232728, 7.677764709599123272, 39.54930799450052348 ) ) ;
#26707=ADVANCED_FACE ( 'NONE', ( #10993 ), #28700, .T. ) ;
#26710=FACE_OUTER_BOUND ( 'NONE', #27404, .T. ) ;
#26713=CARTESIAN_POINT ( 'NONE',  ( -42.03703168893574116, 3.954238390689462257, 48.34930799450052064 ) ) ;
#26714=CARTESIAN_POINT ( 'NONE',  ( -40.68496126738414631, 6.805971067583988621, 39.32862205504143560 ) ) ;
#26715=CARTESIAN_POINT ( 'NONE',  ( -40.51522948349269626, 7.610540244934343335, 60.19810810903209131 ) ) ;
#26724=DIRECTION ( 'NONE',  ( -0.2756373558169974980, 0.9612616959383194493, 1.315048337272770743E-17 ) ) ;
#26725=DIRECTION ( 'NONE',  ( -0.9612616959383206705, -0.2756373558169931681, 1.660411357259282445E-16 ) ) ;
#26730=ORIENTED_EDGE ( 'NONE', *, *, #9003, .T. ) ;
#26737=VECTOR ( 'NONE', #4986, 1000.000000000000227 ) ;
#26738=AXIS2_PLACEMENT_3D ( 'NONE', #20736, #1189, #1351 ) ;
#26742=AXIS2_PLACEMENT_3D ( 'NONE', #17445, #22364, #12538 ) ;
#26744=FACE_OUTER_BOUND ( 'NONE', #6839, .T. ) ;
#26745=ORIENTED_EDGE ( 'NONE', *, *, #23110, .T. ) ;
#26748=CARTESIAN_POINT ( 'NONE',  ( -42.38351229602917414, 14.72295342448899014, 55.13902476097742777 ) ) ;
#26759=ORIENTED_EDGE ( 'NONE', *, *, #15204, .T. ) ;
#26761=DIRECTION ( 'NONE',  ( 1.141485058121273114E-16, 2.056979540075764156E-16, 1.000000000000000000 ) ) ;
#26764=EDGE_LOOP ( 'NONE', ( #10341, #5470, #31854, #20269 ) ) ;
#26776=ORIENTED_EDGE ( 'NONE', *, *, #19465, .T. ) ;
#26777=CARTESIAN_POINT ( 'NONE',  ( -42.39006672483308336, 15.27003693862974032, 35.55750462089839203 ) ) ;
#26781=ORIENTED_EDGE ( 'NONE', *, *, #4819, .T. ) ;
#26784=DIRECTION ( 'NONE',  ( 0.7141240004913198547, -0.3958453973320100738, 0.5773502691896283956 ) ) ;
#26785=CIRCLE ( 'NONE', #24186, 1.100000000000001199 ) ;
#26786=CARTESIAN_POINT ( 'NONE',  ( -40.60333149162104860, 7.557375771971046596, 60.08350751967648762 ) ) ;
#26792=DIRECTION ( 'NONE',  ( 0.000000000000000000, 0.000000000000000000, -1.000000000000000000 ) ) ;
#26793=EDGE_CURVE ( 'NONE', #1187, #26371, #2102, .T. ) ;
#26794=ADVANCED_FACE ( 'NONE', ( #17027 ), #21947, .F. ) ;
#26800=AXIS2_PLACEMENT_3D ( 'NONE', #15136, #20214, #5452 ) ;
#26801=DIRECTION ( 'NONE',  ( 0.2756373558169954441, -0.9612616959383198934, 1.479773560108263204E-16 ) ) ;
#26807=DIRECTION ( 'NONE',  ( 2.779292025043186357E-18, -1.288349127009862211E-17, 1.000000000000000000 ) ) ;
#26808=VERTEX_POINT ( 'NONE', #21630 ) ;
#26809=ORIENTED_EDGE ( 'NONE', *, *, #20084, .T. ) ;
#26810=CARTESIAN_POINT ( 'NONE',  ( -40.10975985016548151, 6.833710191006538537, 39.48304619656028791 ) ) ;
#26812=CARTESIAN_POINT ( 'NONE',  ( -38.36853489569023168, 7.065850718397949315, 32.04930799450052348 ) ) ;
#26815=ORIENTED_EDGE ( 'NONE', *, *, #20436, .F. ) ;
#26821=CARTESIAN_POINT ( 'NONE',  ( -40.60497062835319326, 7.562013838793847142, 53.87859731638185679 ) ) ;
#26835=ADVANCED_FACE ( 'NONE', ( #19162 ), #10362, .T. ) ;
#26842=CARTESIAN_POINT ( 'NONE',  ( -43.38408989745150990, 1.111547985471240008, 53.64930799450051779 ) ) ;
#26846=CARTESIAN_POINT ( 'NONE',  ( -40.11036131418492090, 6.815955993705607341, 34.73729068726325409 ) ) ;
#26848=EDGE_LOOP ( 'NONE', ( #15717, #6031, #1041 ) ) ;
#26851=CONICAL_SURFACE ( 'NONE', #3251, 1.003191532947548925, 0.7853981633974477239 ) ;
#26855=TOROIDAL_SURFACE ( 'NONE', #27447, 0.9000000000000003553, 0.1000000000000000056 ) ;
#26858=VECTOR ( 'NONE', #21632, 1000.000000000000114 ) ;
#26860=ADVANCED_FACE ( 'NONE', ( #32148 ), #21460, .F. ) ;
#26871=EDGE_CURVE ( 'NONE', #23906, #22442, #20956, .T. ) ;
#26872=EDGE_LOOP ( 'NONE', ( #32231, #5277, #25401 ) ) ;
#26874=ORIENTED_EDGE ( 'NONE', *, *, #179, .T. ) ;
#26877=CYLINDRICAL_SURFACE ( 'NONE', #18380, 0.1000000000000007272 ) ;
#26879=CARTESIAN_POINT ( 'NONE',  ( -40.59290754354907449, 7.518856927436782911, 60.12739743091343314 ) ) ;
#26887=CYLINDRICAL_SURFACE ( 'NONE', #7247, 0.1000000000000020595 ) ;
#26893=EDGE_CURVE ( 'NONE', #11047, #13254, #27658, .T. ) ;
#26897=ADVANCED_FACE ( 'NONE', ( #886 ), #15188, .T. ) ;
#26898=ORIENTED_EDGE ( 'NONE', *, *, #7192, .T. ) ;
#26904=( BOUNDED_CURVE ( )  B_SPLINE_CURVE ( 3, ( #13210, #871, #23200, #18259 ),
 .UNSPECIFIED., .F., .F. ) 
 B_SPLINE_CURVE_WITH_KNOTS ( ( 4, 4 ),
 ( 1.575603059825828550E-14, 1.570796326794877462 ),
 .UNSPECIFIED. ) 
 CURVE ( )  GEOMETRIC_REPRESENTATION_ITEM ( )  RATIONAL_B_SPLINE_CURVE ( ( 1.000000000000000000, 0.8047378541243732641, 0.8047378541243732641, 1.000000000000000000 ) ) 
 REPRESENTATION_ITEM ( '' )  );
#26911=LINE ( 'NONE', #31678, #2575 ) ;
#26912=LINE ( 'NONE', #22627, #25950 ) ;
#26922=ORIENTED_EDGE ( 'NONE', *, *, #31795, .F. ) ;
#26924=DIRECTION ( 'NONE',  ( 0.9612616959383221138, 0.2756373558169876170, 0.000000000000000000 ) ) ;
#26925=CYLINDRICAL_SURFACE ( 'NONE', #8329, 0.1000000000000014905 ) ;
#26926=VECTOR ( 'NONE', #8129, 1000.000000000000114 ) ;
#26930=FACE_OUTER_BOUND ( 'NONE', #23215, .T. ) ;
#26933=DIRECTION ( 'NONE',  ( -1.188208965918165239E-16, -1.880121038077813132E-16, -1.000000000000000000 ) ) ;
#26945=CARTESIAN_POINT ( 'NONE',  ( -40.52510752649232728, 7.677764709599123272, 39.54930799450052348 ) ) ;
#26949=DIRECTION ( 'NONE',  ( 0.4848096202463424431, 0.8746197071393927436, -2.220446049250312588E-16 ) ) ;
#26950=DIRECTION ( 'NONE',  ( -1.188208965918165239E-16, -1.880121038077813132E-16, -1.000000000000000000 ) ) ;
#26953=CARTESIAN_POINT ( 'NONE',  ( -40.63181322188042088, 6.822514116776794424, 39.52939200191682545 ) ) ;
#26954=ORIENTED_EDGE ( 'NONE', *, *, #30400, .F. ) ;
#26956=CARTESIAN_POINT ( 'NONE',  ( -40.44670421500372015, 8.525092865626815453, 34.54930799450052348 ) ) ;
#26965=ORIENTED_EDGE ( 'NONE', *, *, #1293, .F. ) ;
#26967=CARTESIAN_POINT ( 'NONE',  ( -40.11688989807090167, 6.803825020423238890, 39.45035836127284767 ) ) ;
#26969=DIRECTION ( 'NONE',  ( -0.2756373558169932236, 0.9612616959383206705, -2.468067202294475228E-14 ) ) ;
#26974=AXIS2_PLACEMENT_3D ( 'NONE', #15807, #13352, #4127 ) ;
#26975=VERTEX_POINT ( 'NONE', #13228 ) ;
#26980=ADVANCED_FACE ( 'NONE', ( #30619 ), #17804, .T. ) ;
#26983=CARTESIAN_POINT ( 'NONE',  ( -41.88090303775678080, 13.82677487427665497, 54.64930799450051779 ) ) ;
#26985=AXIS2_PLACEMENT_3D ( 'NONE', #23323, #25778, #8227 ) ;
#26998=CARTESIAN_POINT ( 'NONE',  ( -40.68740604810007966, 6.795923245628763709, 39.47252729750491795 ) ) ;
#27005=CARTESIAN_POINT ( 'NONE',  ( -40.19913497620437681, 7.013551051776422796, 34.87324101432411538 ) ) ;
#27007=LINE ( 'NONE', #14057, #1789 ) ;
#27015=VECTOR ( 'NONE', #16371, 1000.000000000000114 ) ;
#27020=EDGE_CURVE ( 'NONE', #32314, #27140, #20592, .T. ) ;
#27026=ORIENTED_EDGE ( 'NONE', *, *, #12683, .T. ) ;
#27027=DIRECTION ( 'NONE',  ( 0.2756373558169956106, -0.9612616959383200044, -1.315048337272770743E-17 ) ) ;
#27032=VERTEX_POINT ( 'NONE', #22892 ) ;
#27033=CARTESIAN_POINT ( 'NONE',  ( -43.90780810587784089, -0.03953120679776574165, 32.04930799450052348 ) ) ;
#27040=CARTESIAN_POINT ( 'NONE',  ( -40.60333149162104860, 7.557375771971046596, 60.08350751967648762 ) ) ;
#27048=EDGE_CURVE ( 'NONE', #16381, #25031, #497, .T. ) ;
#27049=DIRECTION ( 'NONE',  ( -0.9612616959383206705, -0.2756373558169934457, 1.660411357259282938E-16 ) ) ;
#27051=AXIS2_PLACEMENT_3D ( 'NONE', #19592, #29950, #29618 ) ;
#27053=CARTESIAN_POINT ( 'NONE',  ( -40.98031486389898248, 9.265261353013489298, 39.44930799450052206 ) ) ;
#27057=EDGE_CURVE ( 'NONE', #29530, #4744, #21377, .T. ) ;
#27066=CARTESIAN_POINT ( 'NONE',  ( -39.67555847965937943, 2.645252416024337361, 45.74930799450051211 ) ) ;
#27071=CARTESIAN_POINT ( 'NONE',  ( -43.38408989745150990, 1.111547985471239786, 60.44930799450051495 ) ) ;
#27073=EDGE_CURVE ( 'NONE', #25738, #9355, #1042, .T. ) ;
#27083=DIRECTION ( 'NONE',  ( 0.4848096202463636484, 0.8746197071393810862, 0.000000000000000000 ) ) ;
#27094=LINE ( 'NONE', #24797, #6547 ) ;
#27096=EDGE_CURVE ( 'NONE', #9876, #16357, #20438, .T. ) ;
#27106=EDGE_CURVE ( 'NONE', #1764, #28053, #31976, .T. ) ;
#27112=CARTESIAN_POINT ( 'NONE',  ( -41.23380787120766655, 11.23768311167744294, 36.00717268343339583 ) ) ;
#27117=CARTESIAN_POINT ( 'NONE',  ( -40.64500813507293486, 6.819128862114092193, 39.51928662074344345 ) ) ;
#27119=ORIENTED_EDGE ( 'NONE', *, *, #17976, .T. ) ;
#27120=CARTESIAN_POINT ( 'NONE',  ( -40.60333149162104860, 7.557375771971046596, 54.01510846932454513 ) ) ;
#27121=CARTESIAN_POINT ( 'NONE',  ( -40.43096862161028326, 8.533258663572608427, 34.55282792453323992 ) ) ;
#27122=EDGE_CURVE ( 'NONE', #4349, #8349, #21999, .T. ) ;
#27125=ORIENTED_EDGE ( 'NONE', *, *, #24032, .F. ) ;
#27127=CARTESIAN_POINT ( 'NONE',  ( -43.64073206722599707, 1.267352857069778960, 34.64930799450052490 ) ) ;
#27129=ORIENTED_EDGE ( 'NONE', *, *, #30304, .F. ) ;
#27135=AXIS2_PLACEMENT_3D ( 'NONE', #6065, #18517, #28699 ) ;
#27136=DIRECTION ( 'NONE',  ( 0.2756373558169932236, -0.9612616959383206705, -2.438471731092320121E-14 ) ) ;
#27140=VERTEX_POINT ( 'NONE', #23855 ) ;
#27141=CARTESIAN_POINT ( 'NONE',  ( -41.88090303775678080, 13.82677487427666030, 54.63190069796055326 ) ) ;
#27153=CARTESIAN_POINT ( 'NONE',  ( -40.69088518708426960, 6.792375053915788108, 39.46636398561383174 ) ) ;
#27154=ORIENTED_EDGE ( 'NONE', *, *, #15080, .F. ) ;
#27163=ORIENTED_EDGE ( 'NONE', *, *, #2034, .F. ) ;
#27165=DIRECTION ( 'NONE',  ( 0.8746197071393926326, -0.4848096202463430537, -8.676864087101709653E-18 ) ) ;
#27177=CARTESIAN_POINT ( 'NONE',  ( -40.60251150970604073, 6.748447833883064462, 60.54930799450051637 ) ) ;
#27178=ORIENTED_EDGE ( 'NONE', *, *, #5201, .T. ) ;
#27187=EDGE_LOOP ( 'NONE', ( #13752, #24077 ) ) ;
#27189=CARTESIAN_POINT ( 'NONE',  ( -41.04685960816998147, 9.497330455345890599, 35.54930799450052348 ) ) ;
#27190=VECTOR ( 'NONE', #17002, 1000.000000000000114 ) ;
#27198=EDGE_CURVE ( 'NONE', #13584, #12291, #7327, .T. ) ;
#27199=ADVANCED_FACE ( 'NONE', ( #6300 ), #13856, .T. ) ;
#27202=CARTESIAN_POINT ( 'NONE',  ( -41.02687597405218156, 7.220473278338834788, 53.64930799450051779 ) ) ;
#27206=CARTESIAN_POINT ( 'NONE',  ( -42.28040081837337993, 14.75252016492556351, 58.96875521528360053 ) ) ;
#27219=ADVANCED_FACE ( 'NONE', ( #14508 ), #1577, .T. ) ;
#27220=CARTESIAN_POINT ( 'NONE',  ( -42.37913764077812573, 15.23192269303852697, 38.54930799450052348 ) ) ;
#27226=CIRCLE ( 'NONE', #8375, 0.1000000000000007272 ) ;
#27227=DIRECTION ( 'NONE',  ( 0.6184495258776511184, -0.3428121700606679978, -0.7071067811865504593 ) ) ;
#27240=ORIENTED_EDGE ( 'NONE', *, *, #19461, .T. ) ;
#27256=VECTOR ( 'NONE', #24911, 1000.000000000000000 ) ;
#27258=ADVANCED_FACE ( 'NONE', ( #24501 ), #4982, .T. ) ;
#27262=EDGE_CURVE ( 'NONE', #9355, #6997, #9582, .T. ) ;
#27267=EDGE_CURVE ( 'NONE', #27795, #30194, #32389, .T. ) ;
#27268=ORIENTED_EDGE ( 'NONE', *, *, #1202, .F. ) ;
#27271=FACE_OUTER_BOUND ( 'NONE', #14219, .T. ) ;
#27272=DIRECTION ( 'NONE',  ( 0.4848096202463637039, 0.8746197071393810862, 0.000000000000000000 ) ) ;
#27279=CARTESIAN_POINT ( 'NONE',  ( -42.38687957179150345, 4.148162238788003719, 57.04930799450051637 ) ) ;
#27282=EDGE_CURVE ( 'NONE', #7171, #17901, #8412, .T. ) ;
#27288=VECTOR ( 'NONE', #18481, 1000.000000000000000 ) ;
#27290=CARTESIAN_POINT ( 'NONE',  ( -43.01732049266337299, 16.00634867709746700, 37.04930799450052348 ) ) ;
#27293=( BOUNDED_CURVE ( )  B_SPLINE_CURVE ( 3, ( #23863, #26165, #29277, #8925 ),
 .UNSPECIFIED., .F., .F. ) 
 B_SPLINE_CURVE_WITH_KNOTS ( ( 4, 4 ),
 ( 1.575603059825828550E-14, 1.570796326794877462 ),
 .UNSPECIFIED. ) 
 CURVE ( )  GEOMETRIC_REPRESENTATION_ITEM ( )  RATIONAL_B_SPLINE_CURVE ( ( 1.000000000000000000, 0.8047378541243732641, 0.8047378541243732641, 1.000000000000000000 ) ) 
 REPRESENTATION_ITEM ( '' )  );
#27297=EDGE_LOOP ( 'NONE', ( #15303, #15314, #10173, #19874 ) ) ;
#27299=CARTESIAN_POINT ( 'NONE',  ( -39.58809650894544774, 2.596771453999702661, 47.04930799450051637 ) ) ;
#27302=DIRECTION ( 'NONE',  ( 0.1949050434465252057, -0.6797146636928681485, -0.7071067811865469066 ) ) ;
#27304=ORIENTED_EDGE ( 'NONE', *, *, #17256, .T. ) ;
#27305=EDGE_CURVE ( 'NONE', #3234, #16288, #21504, .T. ) ;
#27307=ADVANCED_FACE ( 'NONE', ( #24841 ), #7284, .T. ) ;
#27308=ORIENTED_EDGE ( 'NONE', *, *, #3031, .T. ) ;
#27309=VECTOR ( 'NONE', #11627, 1000.000000000000000 ) ;
#27310=CIRCLE ( 'NONE', #18897, 2.000000000000001776 ) ;
#27312=DIRECTION ( 'NONE',  ( -0.9612616959383194493, -0.2756373558169974980, -8.795445018804946186E-19 ) ) ;
#27314=EDGE_CURVE ( 'NONE', #8640, #17298, #8879, .T. ) ;
#27321=CARTESIAN_POINT ( 'NONE',  ( -40.86580004447909431, 8.503105189880379555, 34.64930799450051779 ) ) ;
#27322=ORIENTED_EDGE ( 'NONE', *, *, #18011, .T. ) ;
#27323=CARTESIAN_POINT ( 'NONE',  ( -41.89334324224038397, 13.85403361400641487, 59.48354556245477198 ) ) ;
#27324=DIRECTION ( 'NONE',  ( -1.188208965918165239E-16, -1.880121038077813132E-16, -1.000000000000000000 ) ) ;
#27325=ORIENTED_EDGE ( 'NONE', *, *, #8371, .F. ) ;
#27327=DIRECTION ( 'NONE',  ( 0.9612616959383221138, 0.2756373558169876170, 0.000000000000000000 ) ) ;
#27329=DIRECTION ( 'NONE',  ( 0.000000000000000000, 0.000000000000000000, -1.000000000000000000 ) ) ;
#27332=EDGE_LOOP ( 'NONE', ( #16561, #7761, #15764, #17382 ) ) ;
#27333=AXIS2_PLACEMENT_3D ( 'NONE', #20791, #8322, #30978 ) ;
#27335=FACE_OUTER_BOUND ( 'NONE', #25736, .T. ) ;
#27336=VERTEX_POINT ( 'NONE', #57 ) ;
#27337=AXIS2_PLACEMENT_3D ( 'NONE', #5009, #19759, #32090 ) ;
#27342=DIRECTION ( 'NONE',  ( -0.6184495258776593340, 0.3428121700606657218, 0.7071067811865445751 ) ) ;
#27347=EDGE_CURVE ( 'NONE', #8513, #2319, #25329, .T. ) ;
#27348=AXIS2_PLACEMENT_3D ( 'NONE', #26670, #14533, #31447 ) ;
#27350=ADVANCED_FACE ( 'NONE', ( #10075 ), #15796, .T. ) ;
#27351=VECTOR ( 'NONE', #9798, 1000.000000000000000 ) ;
#27358=DIRECTION ( 'NONE',  ( 0.8746197071393926326, -0.4848096202463430537, -8.676864087101709653E-18 ) ) ;
#27360=EDGE_LOOP ( 'NONE', ( #17785, #19175, #14762, #19368 ) ) ;
#27364=DIRECTION ( 'NONE',  ( 0.000000000000000000, 0.000000000000000000, -1.000000000000000000 ) ) ;
#27382=ORIENTED_EDGE ( 'NONE', *, *, #15866, .T. ) ;
#27383=AXIS2_PLACEMENT_3D ( 'NONE', #451, #7528, #27874 ) ;
#27384=ORIENTED_EDGE ( 'NONE', *, *, #18845, .F. ) ;
#27385=DIRECTION ( 'NONE',  ( 0.6797146636928662611, 0.1949050434465333104, -0.7071067811865466846 ) ) ;
#27389=EDGE_CURVE ( 'NONE', #2185, #10889, #8096, .T. ) ;
#27390=VECTOR ( 'NONE', #23487, 1000.000000000000000 ) ;
#27395=EDGE_CURVE ( 'NONE', #2451, #25827, #697, .T. ) ;
#27396=LINE ( 'NONE', #2921, #23848 ) ;
#27399=EDGE_LOOP ( 'NONE', ( #9150, #24919, #1441, #19741 ) ) ;
#27401=DIRECTION ( 'NONE',  ( 0.8746197071393858602, -0.4848096202463547666, 0.000000000000000000 ) ) ;
#27404=EDGE_LOOP ( 'NONE', ( #26361, #23240, #11583, #23268 ) ) ;
#27405=ORIENTED_EDGE ( 'NONE', *, *, #7947, .F. ) ;
#27407=ORIENTED_EDGE ( 'NONE', *, *, #26387, .T. ) ;
#27408=DIRECTION ( 'NONE',  ( -0.6184495258776542270, 0.3428121700606624467, -0.7071067811865504593 ) ) ;
#27409=DIRECTION ( 'NONE',  ( -2.779292025043186357E-18, 1.288349127009862211E-17, -1.000000000000000000 ) ) ;
#27412=LINE ( 'NONE', #30364, #10079 ) ;
#27415=ORIENTED_EDGE ( 'NONE', *, *, #2442, .F. ) ;
#27417=CARTESIAN_POINT ( 'NONE',  ( -40.70508238852949745, 9.491303552449114278, 38.64930799450052490 ) ) ;
#27419=AXIS2_PLACEMENT_3D ( 'NONE', #14741, #27693, #22764 ) ;
#27423=ORIENTED_EDGE ( 'NONE', *, *, #18843, .T. ) ;
#27424=CARTESIAN_POINT ( 'NONE',  ( -42.36334586133936853, 13.70277685985800531, 59.47272913308562181 ) ) ;
#27425=CARTESIAN_POINT ( 'NONE',  ( -40.57861772207635198, 7.624524047285948569, 53.95737344240558286 ) ) ;
#27430=ORIENTED_EDGE ( 'NONE', *, *, #3935, .T. ) ;
#27432=ORIENTED_EDGE ( 'NONE', *, *, #31312, .T. ) ;
#27434=DIRECTION ( 'NONE',  ( 0.8746197071393926326, -0.4848096202463430537, -8.676864087101709653E-18 ) ) ;
#27438=VECTOR ( 'NONE', #28349, 1000.000000000000000 ) ;
#27440=CIRCLE ( 'NONE', #10612, 0.1000000000000011019 ) ;
#27441=CARTESIAN_POINT ( 'NONE',  ( -42.46007270772396680, 14.70100007970371792, 55.14582903391912083 ) ) ;
#27444=DIRECTION ( 'NONE',  ( 0.8746197071393858602, -0.4848096202463547666, 0.000000000000000000 ) ) ;
#27445=AXIS2_PLACEMENT_3D ( 'NONE', #22236, #7647, #15186 ) ;
#27447=AXIS2_PLACEMENT_3D ( 'NONE', #23443, #954, #3574 ) ;
#27451=DIRECTION ( 'NONE',  ( -1.141485058121273361E-16, -2.056979540075764649E-16, -1.000000000000000000 ) ) ;
#27456=CARTESIAN_POINT ( 'NONE',  ( -42.38687957179149635, 4.148162238788000167, 35.04930799450051637 ) ) ;
#27462=DIRECTION ( 'NONE',  ( -0.2756373558169956106, 0.9612616959383200044, 8.829587629302095151E-15 ) ) ;
#27465=ORIENTED_EDGE ( 'NONE', *, *, #30846, .F. ) ;
#27466=ORIENTED_EDGE ( 'NONE', *, *, #21810, .T. ) ;
#27470=LINE ( 'NONE', #7615, #26737 ) ;
#27475=ORIENTED_EDGE ( 'NONE', *, *, #13601, .F. ) ;
#27478=ORIENTED_EDGE ( 'NONE', *, *, #20971, .T. ) ;
#27479=FACE_OUTER_BOUND ( 'NONE', #31353, .T. ) ;
#27483=EDGE_LOOP ( 'NONE', ( #1386, #30970, #19159, #8987 ) ) ;
#27487=( BOUNDED_CURVE ( )  B_SPLINE_CURVE ( 3, ( #27189, #22266, #27528, #2900 ),
 .UNSPECIFIED., .F., .F. ) 
 B_SPLINE_CURVE_WITH_KNOTS ( ( 4, 4 ),
 ( -8.881784197001252323E-16, 1.570796326794894338 ),
 .UNSPECIFIED. ) 
 CURVE ( )  GEOMETRIC_REPRESENTATION_ITEM ( )  RATIONAL_B_SPLINE_CURVE ( ( 1.000000000000000000, 0.8047378541243652705, 0.8047378541243652705, 1.000000000000000000 ) ) 
 REPRESENTATION_ITEM ( '' )  );
#27495=AXIS2_PLACEMENT_3D ( 'NONE', #28936, #1676, #22012 ) ;
#27499=SPHERICAL_SURFACE ( 'NONE', #8968, 0.1000000000000000056 ) ;
#27503=ORIENTED_EDGE ( 'NONE', *, *, #1512, .T. ) ;
#27507=EDGE_CURVE ( 'NONE', #9841, #16253, #10956, .T. ) ;
#27508=ORIENTED_EDGE ( 'NONE', *, *, #15044, .T. ) ;
#27509=LINE ( 'NONE', #30141, #32461 ) ;
#27512=CIRCLE ( 'NONE', #13369, 2.000000000000001776 ) ;
#27519=CARTESIAN_POINT ( 'NONE',  ( -43.42682711710880739, 1.034448000281938285, 39.44930799450052916 ) ) ;
#27520=CARTESIAN_POINT ( 'NONE',  ( -40.11286833322908052, 2.887657226147511302, 58.94930799450051495 ) ) ;
#27522=ADVANCED_FACE ( 'NONE', ( #13501 ), #5792, .T. ) ;
#27528=CARTESIAN_POINT ( 'NONE',  ( -41.13825658839732569, 9.453274076459845077, 35.59072935073783128 ) ) ;
#27535=DIRECTION ( 'NONE',  ( -0.4848096202463636484, -0.8746197071393810862, 0.000000000000000000 ) ) ;
#27539=CARTESIAN_POINT ( 'NONE',  ( -42.35594856044747303, 14.62682725489516145, 60.54930799450051637 ) ) ;
#27545=VERTEX_POINT ( 'NONE', #31059 ) ;
#27548=VECTOR ( 'NONE', #12555, 1000.000000000000114 ) ;
#27549=DIRECTION ( 'NONE',  ( 0.4848096202463429982, 0.8746197071393925215, 9.920727850371700117E-18 ) ) ;
#27551=ORIENTED_EDGE ( 'NONE', *, *, #13537, .T. ) ;
#27553=EDGE_LOOP ( 'NONE', ( #14625, #13863, #24128, #15842 ) ) ;
#27558=AXIS2_PLACEMENT_3D ( 'NONE', #25307, #9559, #20211 ) ;
#27564=ORIENTED_EDGE ( 'NONE', *, *, #11607, .T. ) ;
#27565=ORIENTED_EDGE ( 'NONE', *, *, #10195, .T. ) ;
#27581=ADVANCED_FACE ( 'NONE', ( #11506, #21503 ), #9049, .F. ) ;
#27585=DIRECTION ( 'NONE',  ( 0.1949050434465283144, -0.6797146636928682595, -0.7071067811865461294 ) ) ;
#27587=AXIS2_PLACEMENT_3D ( 'NONE', #14787, #32184, #30049 ) ;
#27593=DIRECTION ( 'NONE',  ( 0.4848096202463645921, 0.8746197071393805311, 0.000000000000000000 ) ) ;
#27596=ORIENTED_EDGE ( 'NONE', *, *, #26111, .F. ) ;
#27597=CARTESIAN_POINT ( 'NONE',  ( -39.58809650894544774, 2.596771453999702661, 47.04930799450051637 ) ) ;
#27599=EDGE_CURVE ( 'NONE', #19419, #31307, #3473, .T. ) ;
#27603=CARTESIAN_POINT ( 'NONE',  ( -40.59710828457676968, 7.548125289910839975, 60.23404236618278418 ) ) ;
#27604=PLANE ( 'NONE',  #26800 ) ;
#27606=CARTESIAN_POINT ( 'NONE',  ( -40.28779227465695811, 2.984619150196779813, 57.04930799450051637 ) ) ;
#27607=DIRECTION ( 'NONE',  ( 0.4848096202463430537, 0.8746197071393926326, 1.323854077651070671E-16 ) ) ;
#27609=VERTEX_POINT ( 'NONE', #23664 ) ;
#27614=ADVANCED_FACE ( 'NONE', ( #16267 ), #21026, .F. ) ;
#27616=EDGE_CURVE ( 'NONE', #23429, #3682, #10145, .T. ) ;
#27617=ADVANCED_FACE ( 'NONE', ( #6102 ), #19862, .T. ) ;
#27620=DIRECTION ( 'NONE',  ( 2.779292025043186357E-18, -1.288349127009862211E-17, 1.000000000000000000 ) ) ;
#27622=VERTEX_POINT ( 'NONE', #17234 ) ;
#27654=ORIENTED_EDGE ( 'NONE', *, *, #19251, .T. ) ;
#27658=LINE ( 'NONE', #5180, #7873 ) ;
#27661=CIRCLE ( 'NONE', #23988, 0.1000000000000006301 ) ;
#27666=ORIENTED_EDGE ( 'NONE', *, *, #24683, .F. ) ;
#27669=AXIS2_PLACEMENT_3D ( 'NONE', #30959, #5681, #18776 ) ;
#27678=EDGE_LOOP ( 'NONE', ( #8898, #19902 ) ) ;
#27690=FACE_OUTER_BOUND ( 'NONE', #10500, .T. ) ;
#27692=CARTESIAN_POINT ( 'NONE',  ( -42.21195563036362586, 4.051200314738734320, 59.04930799450051637 ) ) ;
#27693=DIRECTION ( 'NONE',  ( -1.188208965918164993E-16, -1.880121038077812639E-16, -1.000000000000000000 ) ) ;
#27696=CARTESIAN_POINT ( 'NONE',  ( -39.50554051497144314, 7.696103224718195968, 61.94930799450052206 ) ) ;
#27702=VECTOR ( 'NONE', #22669, 1000.000000000000114 ) ;
#27705=VECTOR ( 'NONE', #26801, 1000.000000000000227 ) ;
#27709=CARTESIAN_POINT ( 'NONE',  ( -40.99628586177130529, 8.927770518203464789, 58.05249952744806308 ) ) ;
#27711=ORIENTED_EDGE ( 'NONE', *, *, #4571, .F. ) ;
#27717=ADVANCED_FACE ( 'NONE', ( #4448 ), #12000, .F. ) ;
#27728=CARTESIAN_POINT ( 'NONE',  ( -42.47434154250544225, 4.196643200812637531, 57.04930799450051637 ) ) ;
#27729=ORIENTED_EDGE ( 'NONE', *, *, #10584, .F. ) ;
#27740=DIRECTION ( 'NONE',  ( -0.2756373558169954441, 0.9612616959383198934, -1.479773560108263204E-16 ) ) ;
#27742=EDGE_LOOP ( 'NONE', ( #7786, #3434, #19751, #18366, #16644 ) ) ;
#27753=EDGE_LOOP ( 'NONE', ( #23000, #12582 ) ) ;
#27754=CARTESIAN_POINT ( 'NONE',  ( -40.28136326135769707, 8.248516754564388265, 59.50788663826320146 ) ) ;
#27758=ORIENTED_EDGE ( 'NONE', *, *, #998, .T. ) ;
#27760=DIRECTION ( 'NONE',  ( 2.779292025043186357E-18, -1.288349127009862211E-17, 1.000000000000000000 ) ) ;
#27765=CYLINDRICAL_SURFACE ( 'NONE', #19153, 0.1000000000000007272 ) ;
#27768=CARTESIAN_POINT ( 'NONE',  ( -40.99628586177130529, 8.927770518203464789, 56.04611646155296256 ) ) ;
#27773=VERTEX_POINT ( 'NONE', #30372 ) ;
#27776=CARTESIAN_POINT ( 'NONE',  ( -43.84458661617622255, -0.1317431541793673277, 61.99930799450051921 ) ) ;
#27783=VECTOR ( 'NONE', #20575, 1000.000000000000114 ) ;
#27786=ORIENTED_EDGE ( 'NONE', *, *, #19616, .F. ) ;
#27790=VECTOR ( 'NONE', #23701, 1000.000000000000114 ) ;
#27795=VERTEX_POINT ( 'NONE', #10688 ) ;
#27796=B_SPLINE_CURVE_WITH_KNOTS ( 'NONE', 3,
 ( #2380, #14692, #24697, #30271, #72, #29955, #9767, #2696, #22220, #10095, #5004, #29784, #2848, #7299, #17299, #7470, #27812, #19756, #27321 ),
 .UNSPECIFIED., .F., .F.,
 ( 4, 3, 3, 3, 3, 3, 4 ),
 ( 0.000000000000000000, 2.676417781644011357E-05, 5.329639190753654004E-05, 9.120475318091182042E-05, 0.0001427884462350388043, 0.0001845748449448716228, 0.0001865811973795250859 ),
 .UNSPECIFIED. ) ;
#27806=DIRECTION ( 'NONE',  ( -0.2756373558170082672, 0.9612616959383162296, 0.000000000000000000 ) ) ;
#27807=ADVANCED_FACE ( 'NONE', ( #8058 ), #8936, .T. ) ;
#27809=VECTOR ( 'NONE', #5471, 1000.000000000000114 ) ;
#27812=CARTESIAN_POINT ( 'NONE',  ( -40.86555073846352570, 8.502249289700491985, 34.64831079233957212 ) ) ;
#27813=ORIENTED_EDGE ( 'NONE', *, *, #20161, .T. ) ;
#27815=CARTESIAN_POINT ( 'NONE',  ( -42.21195563036361875, 4.051200314738730768, 37.04930799450052348 ) ) ;
#27823=DIRECTION ( 'NONE',  ( 0.4848096202463673676, 0.8746197071393789768, 0.000000000000000000 ) ) ;
#27824=ORIENTED_EDGE ( 'NONE', *, *, #9990, .F. ) ;
#27834=DIRECTION ( 'NONE',  ( -0.9612616959383205595, -0.2756373558169932236, 1.660411357259282445E-16 ) ) ;
#27838=EDGE_CURVE ( 'NONE', #21395, #4349, #28358, .T. ) ;
#27841=CARTESIAN_POINT ( 'NONE',  ( -40.06561427811386267, 7.496110634155836117, 60.44930799450051495 ) ) ;
#27845=ORIENTED_EDGE ( 'NONE', *, *, #5634, .F. ) ;
#27848=DIRECTION ( 'NONE',  ( 0.1949050434465325055, -0.6797146636928671493, 0.7071067811865460184 ) ) ;
#27851=AXIS2_PLACEMENT_3D ( 'NONE', #30121, #31923, #19598 ) ;
#27855=ORIENTED_EDGE ( 'NONE', *, *, #13107, .T. ) ;
#27857=CARTESIAN_POINT ( 'NONE',  ( -42.37913764077812573, 15.23192269303852697, 38.44930799450052916 ) ) ;
#27858=AXIS2_PLACEMENT_3D ( 'NONE', #3384, #23256, #5695 ) ;
#27863=CARTESIAN_POINT ( 'NONE',  ( -42.59587854516874472, -0.7667456371672799476, 47.04930799450051637 ) ) ;
#27868=B_SPLINE_CURVE_WITH_KNOTS ( 'NONE', 3,
 ( #12154, #32175, #19684, #25272, #4925, #15419, #24950, #17222, #7711, #5251, #2297, #14780, #9690 ),
 .UNSPECIFIED., .F., .F.,
 ( 4, 3, 3, 3, 4 ),
 ( -1.894624554243639413E-05, 0.000000000000000000, 3.302537635573856920E-05, 7.371668740090159136E-05, 0.0001101628305730022953 ),
 .UNSPECIFIED. ) ;
#27870=CARTESIAN_POINT ( 'NONE',  ( -40.60722745863126448, 9.415333058485023443, 38.60788663826321709 ) ) ;
#27873=EDGE_CURVE ( 'NONE', #21830, #1880, #16833, .T. ) ;
#27874=DIRECTION ( 'NONE',  ( -0.2756373558170018279, 0.9612616959383181170, 0.000000000000000000 ) ) ;
#27890=DIRECTION ( 'NONE',  ( -0.9612616959383207815, -0.2756373558169930016, 1.660411357259282199E-16 ) ) ;
#27892=ORIENTED_EDGE ( 'NONE', *, *, #5163, .T. ) ;
#27895=EDGE_LOOP ( 'NONE', ( #6955, #29563, #21981 ) ) ;
#27896=CARTESIAN_POINT ( 'NONE',  ( -40.11286833322907341, 2.887657226147507306, 37.04930799450052348 ) ) ;
#27899=DIRECTION ( 'NONE',  ( 0.9612616959383191162, 0.2756373558169986082, 8.795445018805098335E-19 ) ) ;
#27907=DIRECTION ( 'NONE',  ( 0.9612616959383221138, 0.2756373558169876170, 0.000000000000000000 ) ) ;
#27914=EDGE_CURVE ( 'NONE', #20784, #30017, #14715, .T. ) ;
#27919=EDGE_LOOP ( 'NONE', ( #15428, #30627, #23079, #7724 ) ) ;
#27927=LINE ( 'NONE', #8075, #17337 ) ;
#27928=CARTESIAN_POINT ( 'NONE',  ( -42.30123736278718383, 13.66041317296246937, 54.56265170360538264 ) ) ;
#27932=CARTESIAN_POINT ( 'NONE',  ( -40.64500813507293486, 6.819128862114091305, 34.57932936825760351 ) ) ;
#27934=DIRECTION ( 'NONE',  ( -0.8746197071393858602, 0.4848096202463547666, 0.000000000000000000 ) ) ;
#27935=AXIS2_PLACEMENT_3D ( 'NONE', #20166, #30192, #7703 ) ;
#27945=VECTOR ( 'NONE', #8494, 1000.000000000000114 ) ;
#27948=CARTESIAN_POINT ( 'NONE',  ( -40.01678386995657632, 7.136726190597403985, 38.88517396861320918 ) ) ;
#27950=EDGE_LOOP ( 'NONE', ( #14618, #17340, #4094 ) ) ;
#27951=DIRECTION ( 'NONE',  ( -0.4848096202463429982, -0.8746197071393925215, -9.920727850371698576E-18 ) ) ;
#27957=EDGE_LOOP ( 'NONE', ( #31501, #27551, #1909, #6275 ) ) ;
#27962=VERTEX_POINT ( 'NONE', #23464 ) ;
#27963=AXIS2_PLACEMENT_3D ( 'NONE', #30134, #32427, #20422 ) ;
#27965=( BOUNDED_SURFACE ( )  B_SPLINE_SURFACE ( 3, 2, ( 
 ( #4521, #12079, #21585 ),
 ( #16504, #19278, #24376 ),
 ( #26680, #21414, #26358 ),
 ( #14221, #14540, #1565 ),
 ( #31456, #22073, #29305 ),
 ( #26846, #8793, #11751 ),
 ( #19452, #6825, #1895 ),
 ( #18791, #3876, #16824 ) ),
 .UNSPECIFIED., .F., .F., .F. ) 
 B_SPLINE_SURFACE_WITH_KNOTS ( ( 4, 2, 2, 4 ),
 ( 3, 3 ),
 ( -1.490777987167568597E-18, 0.0005623261017282611598, 0.0008434891525923924986, 0.001124652203456523837 ),
 ( 0.000000000000000000, 1.000000000000000000 ),
 .UNSPECIFIED. ) 
 GEOMETRIC_REPRESENTATION_ITEM ( )  RATIONAL_B_SPLINE_SURFACE ( (
 ( 1.000000000000000000, 0.7071067811865558994, 1.000000000000000000),
 ( 1.000000000000000000, 0.6846567335762145934, 1.000000000000000000),
 ( 1.000000000000000000, 0.6190846722317443485, 1.000000000000000000),
 ( 1.000000000000000000, 0.5161161862683902868, 1.000000000000000000),
 ( 1.000000000000000000, 0.4814351115860299180, 1.000000000000000000),
 ( 1.000000000000000000, 0.4264341115149925532, 1.000000000000000000),
 ( 1.000000000000000000, 0.4080770041851934926, 1.000000000000000000),
 ( 1.000000000000000000, 0.4082482904638556342, 1.000000000000000000) ) ) 
 REPRESENTATION_ITEM ( '' )  SURFACE ( )  );
#27970=ORIENTED_EDGE ( 'NONE', *, *, #22162, .T. ) ;
#27974=DIRECTION ( 'NONE',  ( 0.000000000000000000, 0.000000000000000000, -1.000000000000000000 ) ) ;
#27978=DIRECTION ( 'NONE',  ( -0.4848096202463673121, -0.8746197071393789768, 0.000000000000000000 ) ) ;
#27989=FACE_OUTER_BOUND ( 'NONE', #28318, .T. ) ;
#27991=CARTESIAN_POINT ( 'NONE',  ( -40.02540636251514172, 2.839176264122877047, 57.04930799450051637 ) ) ;
#27993=EDGE_CURVE ( 'NONE', #13215, #9599, #31314, .T. ) ;
#27995=VERTEX_POINT ( 'NONE', #11160 ) ;
#27997=FACE_OUTER_BOUND ( 'NONE', #6532, .T. ) ;
#28001=CIRCLE ( 'NONE', #13348, 1.899999999999999023 ) ;
#28006=ORIENTED_EDGE ( 'NONE', *, *, #5360, .F. ) ;
#28007=CIRCLE ( 'NONE', #28553, 0.09999999999999939493 ) ;
#28014=CARTESIAN_POINT ( 'NONE',  ( -41.91739890389096956, 13.90674392281399818, 54.59993297551692848 ) ) ;
#28016=LINE ( 'NONE', #11109, #9685 ) ;
#28017=LINE ( 'NONE', #21093, #21616 ) ;
#28021=DIRECTION ( 'NONE',  ( -1.188208965918165239E-16, -1.880121038077813132E-16, -1.000000000000000000 ) ) ;
#28025=CYLINDRICAL_SURFACE ( 'NONE', #7540, 0.1000000000000007272 ) ;
#28027=DIRECTION ( 'NONE',  ( -0.2756373558169932236, 0.9612616959383204485, -1.479773560108267395E-16 ) ) ;
#28033=ADVANCED_FACE ( 'NONE', ( #3435 ), #28558, .T. ) ;
#28037=AXIS2_PLACEMENT_3D ( 'NONE', #17988, #27848, #7993 ) ;
#28039=CIRCLE ( 'NONE', #14934, 0.09999999999999795164 ) ;
#28044=ORIENTED_EDGE ( 'NONE', *, *, #27389, .F. ) ;
#28052=ORIENTED_EDGE ( 'NONE', *, *, #6814, .F. ) ;
#28053=VERTEX_POINT ( 'NONE', #19332 ) ;
#28055=CARTESIAN_POINT ( 'NONE',  ( -40.06561427811386267, 7.496110634155836117, 56.04611646155296256 ) ) ;
#28062=DIRECTION ( 'NONE',  ( 0.9612616959383221138, 0.2756373558169876170, 0.000000000000000000 ) ) ;
#28065=EDGE_LOOP ( 'NONE', ( #26097, #493, #18326, #22352 ) ) ;
#28068=B_SPLINE_CURVE_WITH_KNOTS ( 'NONE', 3,
 ( #24005, #1195, #11223, #3346, #21213, #23372, #28947, #30929, #31250, #18746, #6292, #16299, #879, #20901, #7273, #22026, #4317, #12368, #14828 ),
 .UNSPECIFIED., .F., .F.,
 ( 4, 3, 3, 3, 3, 3, 4 ),
 ( -2.120612755851273058E-06, 0.000000000000000000, 4.415954867017419676E-05, 9.459217447090470185E-05, 0.0001331301346428089677, 0.0001600668633085419994, 0.0001872567722942432159 ),
 .UNSPECIFIED. ) ;
#28072=DIRECTION ( 'NONE',  ( -0.7141240004913222972, 0.3958453973320028019, -0.5773502691896303940 ) ) ;
#28083=VERTEX_POINT ( 'NONE', #31819 ) ;
#28084=EDGE_CURVE ( 'NONE', #18405, #9796, #17898, .T. ) ;
#28085=FACE_OUTER_BOUND ( 'NONE', #11277, .T. ) ;
#28087=DIRECTION ( 'NONE',  ( -2.779292025043186357E-18, 1.288349127009862211E-17, -1.000000000000000000 ) ) ;
#28089=AXIS2_PLACEMENT_3D ( 'NONE', #29206, #21000, #19177 ) ;
#28092=CARTESIAN_POINT ( 'NONE',  ( -40.70508238852950456, 9.491303552449116054, 39.44930799450052206 ) ) ;
#28093=DIRECTION ( 'NONE',  ( -0.8746197071393790878, 0.4848096202463673676, 1.277302113040196197E-17 ) ) ;
#28095=DIRECTION ( 'NONE',  ( -0.9612616959383194493, -0.2756373558169972759, -8.795445018804905742E-19 ) ) ;
#28099=CARTESIAN_POINT ( 'NONE',  ( -39.67555847965937943, 2.645252416024337361, 47.04930799450051637 ) ) ;
#28100=DIRECTION ( 'NONE',  ( -0.4848096202463645921, -0.8746197071393805311, 0.000000000000000000 ) ) ;
#28104=CARTESIAN_POINT ( 'NONE',  ( -43.42682711710880739, 1.034448000281937396, 34.64930799450052490 ) ) ;
#28107=ORIENTED_EDGE ( 'NONE', *, *, #30104, .T. ) ;
#28108=CARTESIAN_POINT ( 'NONE',  ( -41.24971778908466291, 11.62557032131817181, 57.04930799450051637 ) ) ;
#28110=( GEOMETRIC_REPRESENTATION_CONTEXT ( 3 ) GLOBAL_UNCERTAINTY_ASSIGNED_CONTEXT ( ( #20643 ) ) GLOBAL_UNIT_ASSIGNED_CONTEXT ( ( #5776, #8870, #13807 ) ) REPRESENTATION_CONTEXT ( 'NONE', 'WORKASPACE' ) );
#28113=ORIENTED_EDGE ( 'NONE', *, *, #32030, .T. ) ;
#28138=CARTESIAN_POINT ( 'NONE',  ( -42.59587854516874472, -0.7667456371672812798, 32.14930799450051779 ) ) ;
#28145=FACE_OUTER_BOUND ( 'NONE', #26156, .T. ) ;
#28151=CARTESIAN_POINT ( 'NONE',  ( -40.65065394966018175, 6.870367549600012502, 39.15777990219699944 ) ) ;
#28153=ORIENTED_EDGE ( 'NONE', *, *, #23785, .F. ) ;
#28158=CARTESIAN_POINT ( 'NONE',  ( -40.46271621608484281, 3.081581074246047436, 47.04930799450051637 ) ) ;
#28161=SHAPE_REPRESENTATION ( 'Terminals', ( #8172 ), #12388 ) ;
#28166=EDGE_CURVE ( 'NONE', #25278, #1884, #27226, .T. ) ;
#28173=AXIS2_PLACEMENT_3D ( 'NONE', #6776, #19728, #16778 ) ;
#28174=CARTESIAN_POINT ( 'NONE',  ( -40.61463551858322063, 9.441168033762318501, 35.47959690138647204 ) ) ;
#28179=CARTESIAN_POINT ( 'NONE',  ( -41.94956971822180947, 3.905757428664830222, 45.04930799450051637 ) ) ;
#28187=DIRECTION ( 'NONE',  ( -0.2756373558170082672, 0.9612616959383162296, 0.000000000000000000 ) ) ;
#28191=ORIENTED_EDGE ( 'NONE', *, *, #9717, .T. ) ;
#28193=CARTESIAN_POINT ( 'NONE',  ( -42.28651568955962858, 14.71554561121750559, 55.11195069825311776 ) ) ;
#28196=ORIENTED_EDGE ( 'NONE', *, *, #4168, .T. ) ;
#28198=CIRCLE ( 'NONE', #16651, 0.1000000000000014905 ) ;
#28199=ORIENTED_EDGE ( 'NONE', *, *, #1745, .F. ) ;
#28201=CYLINDRICAL_SURFACE ( 'NONE', #1829, 0.1000000000000028644 ) ;
#28207=CARTESIAN_POINT ( 'NONE',  ( -39.64148344771002286, 7.657122216028890982, 61.94930799450052206 ) ) ;
#28209=EDGE_CURVE ( 'NONE', #19002, #24759, #29867, .T. ) ;
#28210=ADVANCED_FACE ( 'NONE', ( #7854 ), #29856, .T. ) ;
#28229=DIRECTION ( 'NONE',  ( 0.000000000000000000, 0.000000000000000000, -1.000000000000000000 ) ) ;
#28234=ORIENTED_EDGE ( 'NONE', *, *, #31531, .F. ) ;
#28235=EDGE_CURVE ( 'NONE', #13775, #22338, #30018, .T. ) ;
#28238=AXIS2_PLACEMENT_3D ( 'NONE', #29195, #29359, #24101 ) ;
#28239=ORIENTED_EDGE ( 'NONE', *, *, #8573, .T. ) ;
#28242=ORIENTED_EDGE ( 'NONE', *, *, #28288, .F. ) ;
#28243=DIRECTION ( 'NONE',  ( -0.2756373558170082672, 0.9612616959383162296, 0.000000000000000000 ) ) ;
#28247=ORIENTED_EDGE ( 'NONE', *, *, #23881, .T. ) ;
#28249=CARTESIAN_POINT ( 'NONE',  ( -41.23380787120766655, 11.23768311167744294, 38.19144330556764544 ) ) ;
#28255=CYLINDRICAL_SURFACE ( 'NONE', #12190, 1.500000000000001332 ) ;
#28260=ORIENTED_EDGE ( 'NONE', *, *, #21589, .T. ) ;
#28261=DIRECTION ( 'NONE',  ( 0.000000000000000000, 0.000000000000000000, 1.000000000000000000 ) ) ;
#28263=DIRECTION ( 'NONE',  ( -0.8746197071393926326, 0.4848096202463430537, 8.676864087101709653E-18 ) ) ;
#28268=CARTESIAN_POINT ( 'NONE',  ( -40.12089184044746304, 6.795442064577189356, 39.45353434682061078 ) ) ;
#28270=EDGE_LOOP ( 'NONE', ( #31184, #11152, #2209 ) ) ;
#28280=ORIENTED_EDGE ( 'NONE', *, *, #1422, .F. ) ;
#28285=EDGE_LOOP ( 'NONE', ( #27304, #10972 ) ) ;
#28287=DIRECTION ( 'NONE',  ( -0.8746197071394243849, 0.4848096202462855997, 0.000000000000000000 ) ) ;
#28288=EDGE_CURVE ( 'NONE', #27336, #17105, #12458, .T. ) ;
#28289=DIRECTION ( 'NONE',  ( 0.4848096202463365034, 0.8746197071393960742, -2.220446049250302481E-16 ) ) ;
#28290=VECTOR ( 'NONE', #16426, 1000.000000000000227 ) ;
#28308=CARTESIAN_POINT ( 'NONE',  ( -40.15599670534037102, 7.478908884098772525, 35.64930799450052490 ) ) ;
#28314=VECTOR ( 'NONE', #10893, 1000.000000000000000 ) ;
#28316=EDGE_CURVE ( 'NONE', #155, #9876, #8888, .T. ) ;
#28318=EDGE_LOOP ( 'NONE', ( #3834, #19996, #20766, #471 ) ) ;
#28319=EDGE_LOOP ( 'NONE', ( #9863, #28581, #30040, #7708 ) ) ;
#28320=EDGE_CURVE ( 'NONE', #25934, #15549, #18084, .T. ) ;
#28322=VECTOR ( 'NONE', #28719, 999.9999999999998863 ) ;
#28327=AXIS2_PLACEMENT_3D ( 'NONE', #3794, #8569, #854 ) ;
#28346=AXIS2_PLACEMENT_3D ( 'NONE', #14702, #1889, #14865 ) ;
#28349=DIRECTION ( 'NONE',  ( -0.1949050434465251780, 0.6797146636928681485, 0.7071067811865470176 ) ) ;
#28351=VERTEX_POINT ( 'NONE', #23587 ) ;
#28354=DIRECTION ( 'NONE',  ( 0.9612616959383221138, 0.2756373558169876170, 0.000000000000000000 ) ) ;
#28358=CIRCLE ( 'NONE', #18369, 0.1000000000000004774 ) ;
#28360=DIRECTION ( 'NONE',  ( -0.8746197071393925215, 0.4848096202463429982, 8.676864087101709653E-18 ) ) ;
#28371=DIRECTION ( 'NONE',  ( -0.9612616959383205595, -0.2756373558169932236, 1.660411357259282445E-16 ) ) ;
#28381=DIRECTION ( 'NONE',  ( 0.000000000000000000, 0.000000000000000000, -1.000000000000000000 ) ) ;
#28385=DIRECTION ( 'NONE',  ( -0.6797146636928670382, -0.1949050434465290915, -0.7071067811865470176 ) ) ;
#28386=ORIENTED_EDGE ( 'NONE', *, *, #27020, .T. ) ;
#28388=PLANE ( 'NONE',  #27135 ) ;
#28393=ORIENTED_EDGE ( 'NONE', *, *, #5029, .T. ) ;
#28399=EDGE_CURVE ( 'NONE', #6416, #2451, #5164, .T. ) ;
#28400=EDGE_CURVE ( 'NONE', #13414, #22288, #5484, .T. ) ;
#28410=CIRCLE ( 'NONE', #15320, 0.09999999999999795164 ) ;
#28412=CIRCLE ( 'NONE', #28925, 0.09999999999999815981 ) ;
#28413=DIRECTION ( 'NONE',  ( 0.000000000000000000, 0.000000000000000000, -1.000000000000000000 ) ) ;
#28416=CARTESIAN_POINT ( 'NONE',  ( -43.64647580959332629, 1.256990871545142774, 53.64930799450051779 ) ) ;
#28424=ORIENTED_EDGE ( 'NONE', *, *, #32216, .T. ) ;
#28425=ORIENTED_EDGE ( 'NONE', *, *, #11807, .F. ) ;
#28426=EDGE_CURVE ( 'NONE', #30888, #30637, #13211, .T. ) ;
#28428=AXIS2_PLACEMENT_3D ( 'NONE', #17309, #12074, #27329 ) ;
#28431=ORIENTED_EDGE ( 'NONE', *, *, #12198, .T. ) ;
#28432=DIRECTION ( 'NONE',  ( 0.000000000000000000, 0.000000000000000000, 1.000000000000000000 ) ) ;
#28435=CARTESIAN_POINT ( 'NONE',  ( -40.60722745863126448, 9.415333058485023443, 34.69072935073783270 ) ) ;
#28439=EDGE_CURVE ( 'NONE', #8660, #23633, #5007, .T. ) ;
#28440=CIRCLE ( 'NONE', #21599, 2.000000000000001776 ) ;
#28445=DIRECTION ( 'NONE',  ( -0.2756373558169959437, 0.9612616959383197823, 0.000000000000000000 ) ) ;
#28447=AXIS2_PLACEMENT_3D ( 'NONE', #20329, #14939, #10019 ) ;
#28448=CARTESIAN_POINT ( 'NONE',  ( -37.58300281841709989, 16.01180101885526597, 38.09144330556765112 ) ) ;
#28462=FACE_OUTER_BOUND ( 'NONE', #20, .T. ) ;
#28465=CARTESIAN_POINT ( 'NONE',  ( -40.38504631157857006, 8.640495317104287309, 34.64880948087299117 ) ) ;
#28471=DIRECTION ( 'NONE',  ( -0.2756373558169954441, 0.9612616959383198934, -1.479773560108263451E-16 ) ) ;
#28475=DIRECTION ( 'NONE',  ( -0.4848096202463424431, -0.8746197071393927436, 2.220446049250312588E-16 ) ) ;
#28476=CARTESIAN_POINT ( 'NONE',  ( -39.67555847965937943, 2.645252416024336028, 45.04930799450051637 ) ) ;
#28478=DIRECTION ( 'NONE',  ( 0.4848096202463429427, 0.8746197071393925215, -2.352477780477436294E-16 ) ) ;
#28489=ADVANCED_FACE ( 'NONE', ( #12890 ), #21231, .T. ) ;
#28498=ORIENTED_EDGE ( 'NONE', *, *, #12586, .F. ) ;
#28500=CARTESIAN_POINT ( 'NONE',  ( -43.82034613516389498, -0.08801216882239978889, 32.04930799450052348 ) ) ;
#28507=DIRECTION ( 'NONE',  ( -0.2756373558169932236, 0.9612616959383205595, 2.536267806945839542E-31 ) ) ;
#28509=ADVANCED_FACE ( 'NONE', ( #18736 ), #25823, .T. ) ;
#28517=ORIENTED_EDGE ( 'NONE', *, *, #3442, .F. ) ;
#28518=CARTESIAN_POINT ( 'NONE',  ( -39.85048242108726413, 2.742214340073605872, 47.04930799450051637 ) ) ;
#28520=ORIENTED_EDGE ( 'NONE', *, *, #8193, .F. ) ;
#28521=AXIS2_PLACEMENT_3D ( 'NONE', #6652, #16646, #27327 ) ;
#28522=ORIENTED_EDGE ( 'NONE', *, *, #5634, .T. ) ;
#28526=VERTEX_POINT ( 'NONE', #3490 ) ;
#28527=EDGE_CURVE ( 'NONE', #13059, #13215, #16124, .T. ) ;
#28528=DIRECTION ( 'NONE',  ( -0.4848096202463405002, -0.8746197071393938538, 0.000000000000000000 ) ) ;
#28530=VERTEX_POINT ( 'NONE', #13519 ) ;
#28533=FACE_OUTER_BOUND ( 'NONE', #19358, .T. ) ;
#28537=CARTESIAN_POINT ( 'NONE',  ( -40.11286833322908052, 2.887657226147511302, 58.34930799450052064 ) ) ;
#28538=ADVANCED_FACE ( 'NONE', ( #13841 ), #6449, .T. ) ;
#28544=( BOUNDED_CURVE ( )  B_SPLINE_CURVE ( 3, ( #6247, #28732, #23958, #6411 ),
 .UNSPECIFIED., .F., .F. ) 
 B_SPLINE_CURVE_WITH_KNOTS ( ( 4, 4 ),
 ( 5.010168875603692840, 6.432075254789125118 ),
 .UNSPECIFIED. ) 
 CURVE ( )  GEOMETRIC_REPRESENTATION_ITEM ( )  RATIONAL_B_SPLINE_CURVE ( ( 1.000000000000000000, 0.8384934736035498659, 0.8384934736035498659, 1.000000000000000000 ) ) 
 REPRESENTATION_ITEM ( '' )  );
#28548=EDGE_LOOP ( 'NONE', ( #16544, #2391, #14430, #30010 ) ) ;
#28551=TOROIDAL_SURFACE ( 'NONE', #27558, 1.299999999999999822, 0.1000000000000000056 ) ;
#28553=AXIS2_PLACEMENT_3D ( 'NONE', #5106, #22982, #22335 ) ;
#28558=PLANE ( 'NONE',  #19899 ) ;
#28565=FACE_OUTER_BOUND ( 'NONE', #19638, .T. ) ;
#28573=DIRECTION ( 'NONE',  ( -0.3958453973319808195, -0.7141240004913296247, 0.5773502691896363892 ) ) ;
#28577=LINE ( 'NONE', #10863, #26469 ) ;
#28581=ORIENTED_EDGE ( 'NONE', *, *, #29864, .T. ) ;
#28584=DIRECTION ( 'NONE',  ( 7.588956326749211550E-18, -4.206627182996912454E-18, 1.000000000000000000 ) ) ;
#28590=CARTESIAN_POINT ( 'NONE',  ( -40.50965841522093314, 7.583953161651079355, 60.22550310247657279 ) ) ;
#28592=AXIS2_PLACEMENT_3D ( 'NONE', #27279, #16330, #1396 ) ;
#28595=ORIENTED_EDGE ( 'NONE', *, *, #17256, .F. ) ;
#28597=DIRECTION ( 'NONE',  ( -0.8746197071393790878, 0.4848096202463673676, 1.277302113040196197E-17 ) ) ;
#28598=DIRECTION ( 'NONE',  ( -0.8746197071393926326, 0.4848096202463430537, 8.676864087101709653E-18 ) ) ;
#28599=EDGE_LOOP ( 'NONE', ( #12827, #12008, #11212, #19386 ) ) ;
#28606=EDGE_CURVE ( 'NONE', #14877, #9695, #8405, .T. ) ;
#28607=CARTESIAN_POINT ( 'NONE',  ( -40.52669582637187062, 7.652910973922026017, 53.94439779120587986 ) ) ;
#28620=AXIS2_PLACEMENT_3D ( 'NONE', #1302, #6078, #26416 ) ;
#28625=CARTESIAN_POINT ( 'NONE',  ( -42.37913764077812573, 15.23192269303853053, 35.64930799450052490 ) ) ;
#28629=CARTESIAN_POINT ( 'NONE',  ( -36.15737491070432696, 8.702841779934164634, 53.64930799450051779 ) ) ;
#28633=AXIS2_PLACEMENT_3D ( 'NONE', #8561, #25632, #8398 ) ;
#28637=EDGE_CURVE ( 'NONE', #11200, #16822, #15299, .T. ) ;
#28639=PLANE ( 'NONE',  #20745 ) ;
#28640=CYLINDRICAL_SURFACE ( 'NONE', #16117, 0.1000000000000014905 ) ;
#28644=ORIENTED_EDGE ( 'NONE', *, *, #27395, .T. ) ;
#28648=EDGE_CURVE ( 'NONE', #90, #21602, #16770, .T. ) ;
#28658=CARTESIAN_POINT ( 'NONE',  ( -38.32955388700093380, 6.929907785659376707, 47.04930799450051637 ) ) ;
#28659=CARTESIAN_POINT ( 'NONE',  ( -42.41019933908752648, 14.71530103803245915, 58.95721942880052779 ) ) ;
#28661=ORIENTED_EDGE ( 'NONE', *, *, #16890, .T. ) ;
#28667=CARTESIAN_POINT ( 'NONE',  ( -40.46271621608484281, 3.081581074246047436, 48.54930799450051637 ) ) ;
#28668=VERTEX_POINT ( 'NONE', #683 ) ;
#28669=ADVANCED_FACE ( 'NONE', ( #12847 ), #3130, .F. ) ;
#28670=ORIENTED_EDGE ( 'NONE', *, *, #20609, .T. ) ;
#28675=EDGE_CURVE ( 'NONE', #16288, #27795, #2642, .T. ) ;
#28676=EDGE_CURVE ( 'NONE', #26626, #16357, #11036, .T. ) ;
#28678=FACE_OUTER_BOUND ( 'NONE', #988, .T. ) ;
#28685=ORIENTED_EDGE ( 'NONE', *, *, #30304, .T. ) ;
#28686=VERTEX_POINT ( 'NONE', #13170 ) ;
#28690=CARTESIAN_POINT ( 'NONE',  ( -40.70098307446854591, 6.778209214780407166, 39.41092630925031415 ) ) ;
#28692=VECTOR ( 'NONE', #13800, 1000.000000000000000 ) ;
#28697=DIRECTION ( 'NONE',  ( -0.8746197071393925215, 0.4848096202463429982, 8.676864087101709653E-18 ) ) ;
#28699=DIRECTION ( 'NONE',  ( -0.2756373558169973870, 0.9612616959383193382, 1.315048337272770435E-17 ) ) ;
#28700=TOROIDAL_SURFACE ( 'NONE', #3079, 0.8928932188134564019, 0.1000000000000000056 ) ;
#28709=CARTESIAN_POINT ( 'NONE',  ( -40.65487266620045403, 9.475231293617264683, 35.46144002885649371 ) ) ;
#28712=ORIENTED_EDGE ( 'NONE', *, *, #26871, .T. ) ;
#28713=ADVANCED_FACE ( 'NONE', ( #22508 ), #3622, .T. ) ;
#28714=ADVANCED_FACE ( 'NONE', ( #30085 ), #2116, .T. ) ;
#28719=DIRECTION ( 'NONE',  ( -0.9612616959383207815, -0.2756373558169926685, -8.795445018804289444E-19 ) ) ;
#28724=( BOUNDED_CURVE ( )  B_SPLINE_CURVE ( 3, ( #29285, #19429, #18770, #24354 ),
 .UNSPECIFIED., .F., .F. ) 
 B_SPLINE_CURVE_WITH_KNOTS ( ( 4, 4 ),
 ( 4.712388980384689674, 5.234911742780512967 ),
 .UNSPECIFIED. ) 
 CURVE ( )  GEOMETRIC_REPRESENTATION_ITEM ( )  RATIONAL_B_SPLINE_CURVE ( ( 1.000000000000000000, 0.9773766218953314766, 0.9773766218953314766, 1.000000000000000000 ) ) 
 REPRESENTATION_ITEM ( '' )  );
#28730=EDGE_LOOP ( 'NONE', ( #30117, #1743, #13627, #13112 ) ) ;
#28732=CARTESIAN_POINT ( 'NONE',  ( -42.48853158357926674, 14.65761848575743898, 58.96871121695127016 ) ) ;
#28744=DIRECTION ( 'NONE',  ( -0.8746197071393926326, 0.4848096202463430537, 8.676864087101709653E-18 ) ) ;
#28747=VECTOR ( 'NONE', #1544, 1000.000000000000227 ) ;
#28750=AXIS2_PLACEMENT_3D ( 'NONE', #1973, #12161, #14463 ) ;
#28754=EDGE_LOOP ( 'NONE', ( #16246, #26745, #32064, #3193 ) ) ;
#28756=CYLINDRICAL_SURFACE ( 'NONE', #6717, 0.1000000000000028644 ) ;
#28763=AXIS2_PLACEMENT_3D ( 'NONE', #7118, #22042, #19583 ) ;
#28767=CARTESIAN_POINT ( 'NONE',  ( -40.18454328187963398, 7.548069831825862330, 60.44930799450051495 ) ) ;
#28769=CYLINDRICAL_SURFACE ( 'NONE', #6883, 0.1000000000000014905 ) ;
#28772=DIRECTION ( 'NONE',  ( 1.188208965918164993E-16, 1.880121038077812639E-16, 1.000000000000000000 ) ) ;
#28776=CARTESIAN_POINT ( 'NONE',  ( -41.56459318755936749, 7.281738416154046156, 60.54930799450051637 ) ) ;
#28777=VECTOR ( 'NONE', #22120, 999.9999999999998863 ) ;
#28779=EDGE_LOOP ( 'NONE', ( #31534, #31058 ) ) ;
#28781=DIRECTION ( 'NONE',  ( -2.472450503250596893E-15, -7.226442137580869828E-16, 1.000000000000000000 ) ) ;
#28783=ORIENTED_EDGE ( 'NONE', *, *, #8371, .T. ) ;
#28784=DIRECTION ( 'NONE',  ( -0.8746197071393926326, 0.4848096202463430537, 8.676864087101709653E-18 ) ) ;
#28788=VERTEX_POINT ( 'NONE', #21327 ) ;
#28793=EDGE_CURVE ( 'NONE', #24444, #17822, #29654, .T. ) ;
#28794=ORIENTED_EDGE ( 'NONE', *, *, #1993, .F. ) ;
#28795=EDGE_CURVE ( 'NONE', #7978, #28788, #24136, .T. ) ;
#28797=EDGE_CURVE ( 'NONE', #28668, #19852, #8395, .T. ) ;
#28799=EDGE_CURVE ( 'NONE', #5512, #21772, #15792, .T. ) ;
#28807=ORIENTED_EDGE ( 'NONE', *, *, #31216, .F. ) ;
#28808=CARTESIAN_POINT ( 'NONE',  ( -42.48178708409979265, 14.60617548783703690, 55.10133939125226021 ) ) ;
#28812=ADVANCED_FACE ( 'NONE', ( #25785 ), #13334, .T. ) ;
#28813=CARTESIAN_POINT ( 'NONE',  ( -39.85048242108726413, 2.742214340073605872, 47.04930799450051637 ) ) ;
#28815=DIRECTION ( 'NONE',  ( -0.9612616959383221138, -0.2756373558169876170, 0.000000000000000000 ) ) ;
#28824=PLANE ( 'NONE',  #15369 ) ;
#28825=EDGE_LOOP ( 'NONE', ( #23760, #14055, #29497, #22747 ) ) ;
#28827=CARTESIAN_POINT ( 'NONE',  ( -40.60023598829667435, 7.576973264584798251, 35.33853321918559942 ) ) ;
#28834=ORIENTED_EDGE ( 'NONE', *, *, #1202, .T. ) ;
#28835=VECTOR ( 'NONE', #2820, 1000.000000000000000 ) ;
#28837=VECTOR ( 'NONE', #7348, 1000.000000000000227 ) ;
#28850=AXIS2_PLACEMENT_3D ( 'NONE', #30044, #27899, #3093 ) ;
#28852=CARTESIAN_POINT ( 'NONE',  ( -40.41647043964083252, 8.356895951721261540, 54.44930799450051495 ) ) ;
#28857=EDGE_LOOP ( 'NONE', ( #25121, #20188, #10503, #7996 ) ) ;
#28859=VERTEX_POINT ( 'NONE', #23489 ) ;
#28863=DIRECTION ( 'NONE',  ( -2.779292025043186357E-18, 1.288349127009862057E-17, -1.000000000000000000 ) ) ;
#28879=CARTESIAN_POINT ( 'NONE',  ( -40.68535844407768565, 8.206233278606877235, 54.52001867261917312 ) ) ;
#28882=DIRECTION ( 'NONE',  ( 0.2756373558169958327, -0.9612616959383198934, 0.000000000000000000 ) ) ;
#28885=AXIS2_PLACEMENT_3D ( 'NONE', #13300, #13132, #26235 ) ;
#28886=VECTOR ( 'NONE', #192, 999.9999999999998863 ) ;
#28891=DIRECTION ( 'NONE',  ( -2.779292025043186357E-18, 1.288349127009862211E-17, -1.000000000000000000 ) ) ;
#28900=CARTESIAN_POINT ( 'NONE',  ( -40.46271621608484281, 3.081581074246047436, 47.04930799450051637 ) ) ;
#28902=ADVANCED_FACE ( 'NONE', ( #11989 ), #14782, .F. ) ;
#28907=SHAPE_REPRESENTATION_RELATIONSHIP ( 'NONE' , 'NONE' ,  #28161, #18649 ) ;
#28909=EDGE_LOOP ( 'NONE', ( #24209, #2951, #12296, #7014 ) ) ;
#28911=DIRECTION ( 'NONE',  ( 0.2756373558170082672, -0.9612616959383162296, 0.000000000000000000 ) ) ;
#28912=AXIS2_PLACEMENT_3D ( 'NONE', #20787, #15384, #10306 ) ;
#28914=EDGE_CURVE ( 'NONE', #29694, #30888, #19191, .T. ) ;
#28916=EDGE_LOOP ( 'NONE', ( #24227, #24172, #8751, #9712 ) ) ;
#28919=ORIENTED_EDGE ( 'NONE', *, *, #3442, .T. ) ;
#28925=AXIS2_PLACEMENT_3D ( 'NONE', #27127, #2017, #30252 ) ;
#28931=DIRECTION ( 'NONE',  ( 0.2756373558170093774, -0.9612616959383158965, 0.000000000000000000 ) ) ;
#28936=CARTESIAN_POINT ( 'NONE',  ( -40.50720532202722524, 7.584939507552747706, 60.08350751967648762 ) ) ;
#28938=LINE ( 'NONE', #16291, #30425 ) ;
#28939=VECTOR ( 'NONE', #11862, 1000.000000000000114 ) ;
#28944=DIRECTION ( 'NONE',  ( -0.6184495258776567805, 0.3428121700606641120, -0.7071067811865474617 ) ) ;
#28945=EDGE_CURVE ( 'NONE', #8738, #3050, #9691, .T. ) ;
#28946=CIRCLE ( 'NONE', #26315, 1.899999999999999023 ) ;
#28947=CARTESIAN_POINT ( 'NONE',  ( -40.10975985016548151, 6.833710191006537649, 34.61556979244075194 ) ) ;
#28952=CYLINDRICAL_SURFACE ( 'NONE', #21319, 0.1000000000000008243 ) ;
#28953=DIRECTION ( 'NONE',  ( 0.2756373558169947779, -0.9612616959383201154, 0.000000000000000000 ) ) ;
#28962=EDGE_LOOP ( 'NONE', ( #16088, #17528, #15537, #725 ) ) ;
#28963=ORIENTED_EDGE ( 'NONE', *, *, #31392, .F. ) ;
#28965=VECTOR ( 'NONE', #11263, 1000.000000000000000 ) ;
#28966=AXIS2_PLACEMENT_3D ( 'NONE', #30293, #15192, #5353 ) ;
#28971=ORIENTED_EDGE ( 'NONE', *, *, #28795, .F. ) ;
#28972=FACE_OUTER_BOUND ( 'NONE', #24349, .T. ) ;
#28973=DIRECTION ( 'NONE',  ( 0.2756373558169942228, -0.9612616959383203374, 0.000000000000000000 ) ) ;
#28974=VERTEX_POINT ( 'NONE', #21977 ) ;
#28985=EDGE_CURVE ( 'NONE', #21737, #6336, #19423, .T. ) ;
#28989=VERTEX_POINT ( 'NONE', #20503 ) ;
#28991=CARTESIAN_POINT ( 'NONE',  ( -40.02540636251514172, 2.839176264122877047, 57.04930799450051637 ) ) ;
#28994=DIRECTION ( 'NONE',  ( -0.8746197071393927436, 0.4848096202463423876, 1.277302113040827440E-17 ) ) ;
#28997=AXIS2_PLACEMENT_3D ( 'NONE', #12043, #9089, #18923 ) ;
#28999=ORIENTED_EDGE ( 'NONE', *, *, #23881, .F. ) ;
#29000=ORIENTED_EDGE ( 'NONE', *, *, #23307, .F. ) ;
#29003=DIRECTION ( 'NONE',  ( 1.431146867680865853E-17, 2.558717127065790464E-17, 1.000000000000000000 ) ) ;
#29005=ORIENTED_EDGE ( 'NONE', *, *, #1216, .F. ) ;
#29009=CIRCLE ( 'NONE', #10161, 2.000000000000001776 ) ;
#29012=ORIENTED_EDGE ( 'NONE', *, *, #11933, .F. ) ;
#29013=VERTEX_POINT ( 'NONE', #318 ) ;
#29016=CARTESIAN_POINT ( 'NONE',  ( -42.03703168893574116, 3.954238390689462257, 48.94930799450051495 ) ) ;
#29020=EDGE_CURVE ( 'NONE', #8513, #14507, #13147, .T. ) ;
#29025=DIRECTION ( 'NONE',  ( 0.1949050434465282311, -0.6797146636928673713, -0.7071067811865470176 ) ) ;
#29026=EDGE_CURVE ( 'NONE', #2319, #23152, #8046, .T. ) ;
#29029=CARTESIAN_POINT ( 'NONE',  ( -40.18454328187963398, 7.548069831825863218, 53.54930799450051637 ) ) ;
#29046=EDGE_CURVE ( 'NONE', #2645, #23989, #20016, .T. ) ;
#29048=DIRECTION ( 'NONE',  ( 0.8746197071393925215, -0.4848096202463429982, -8.676864087101708112E-18 ) ) ;
#29063=DIRECTION ( 'NONE',  ( 0.4848096202463429427, 0.8746197071393925215, -2.352477780477436787E-16 ) ) ;
#29068=CARTESIAN_POINT ( 'NONE',  ( -40.59758774925371938, 7.567737757495683226, 39.54930799450052348 ) ) ;
#29077=AXIS2_PLACEMENT_3D ( 'NONE', #14439, #24433, #31825 ) ;
#29081=EDGE_CURVE ( 'NONE', #9952, #9196, #7881, .T. ) ;
#29082=CARTESIAN_POINT ( 'NONE',  ( -39.58809650894544774, 2.596771453999702661, 47.04930799450051637 ) ) ;
#29091=LINE ( 'NONE', #16767, #28939 ) ;
#29100=DIRECTION ( 'NONE',  ( 0.000000000000000000, 0.000000000000000000, -1.000000000000000000 ) ) ;
#29110=DIRECTION ( 'NONE',  ( -0.4848096202463421656, -0.8746197071393929656, -9.920727850371707821E-18 ) ) ;
#29112=ORIENTED_EDGE ( 'NONE', *, *, #14535, .F. ) ;
#29115=LINE ( 'NONE', #16948, #20406 ) ;
#29120=EDGE_CURVE ( 'NONE', #13785, #20229, #20178, .T. ) ;
#29123=AXIS2_PLACEMENT_3D ( 'NONE', #9475, #7168, #12430 ) ;
#29135=ORIENTED_EDGE ( 'NONE', *, *, #30737, .T. ) ;
#29137=CARTESIAN_POINT ( 'NONE',  ( -43.43257085947613660, 1.024086014757300767, 60.54930799450051637 ) ) ;
#29138=VERTEX_POINT ( 'NONE', #11305 ) ;
#29139=DIRECTION ( 'NONE',  ( 0.8746197071393925215, -0.4848096202463429982, -8.676864087101709653E-18 ) ) ;
#29141=CARTESIAN_POINT ( 'NONE',  ( -40.16174044770769314, 7.468546898574135895, 53.64930799450051779 ) ) ;
#29144=FACE_OUTER_BOUND ( 'NONE', #23238, .T. ) ;
#29151=EDGE_LOOP ( 'NONE', ( #31696, #5752, #5881 ) ) ;
#29155=ORIENTED_EDGE ( 'NONE', *, *, #594, .T. ) ;
#29158=TOROIDAL_SURFACE ( 'NONE', #15014, 1.142135311067127068, 0.1000000000000000056 ) ;
#29159=EDGE_LOOP ( 'NONE', ( #3095, #11390, #24453, #5234 ) ) ;
#29160=EDGE_CURVE ( 'NONE', #1265, #8738, #2148, .T. ) ;
#29162=PLANE ( 'NONE',  #21889 ) ;
#29177=DIRECTION ( 'NONE',  ( -1.188208965918164993E-16, -1.880121038077812639E-16, -1.000000000000000000 ) ) ;
#29179=CARTESIAN_POINT ( 'NONE',  ( -40.50410981870283678, 7.604537000166497585, 38.76008276981544753 ) ) ;
#29187=DIRECTION ( 'NONE',  ( 0.8746197071393926326, -0.4848096202463430537, -8.676864087101709653E-18 ) ) ;
#29190=DIRECTION ( 'NONE',  ( 0.2756373558169954441, -0.9612616959383198934, 1.479773560108263204E-16 ) ) ;
#29195=CARTESIAN_POINT ( 'NONE',  ( -40.70335362822509495, 9.387769322903325886, 39.54930799450052348 ) ) ;
#29196=TOROIDAL_SURFACE ( 'NONE', #1943, 0.9000000000000003553, 0.1000000000000000056 ) ;
#29202=ORIENTED_EDGE ( 'NONE', *, *, #15069, .T. ) ;
#29205=CARTESIAN_POINT ( 'NONE',  ( -42.38687957179149635, 4.148162238787999279, 38.34930799450052064 ) ) ;
#29206=CARTESIAN_POINT ( 'NONE',  ( -40.23967075304302909, 7.740322171013526820, 53.80788663826320573 ) ) ;
#29208=ORIENTED_EDGE ( 'NONE', *, *, #17195, .F. ) ;
#29215=EDGE_LOOP ( 'NONE', ( #19948, #17150, #24610, #1080 ) ) ;
#29219=CARTESIAN_POINT ( 'NONE',  ( -38.36853489569023168, 7.065850718397949315, 32.04930799450052348 ) ) ;
#29225=CARTESIAN_POINT ( 'NONE',  ( -40.06561427811386267, 7.496110634155836117, 59.44930799450051495 ) ) ;
#29232=EDGE_CURVE ( 'NONE', #4736, #5228, #16378, .T. ) ;
#29235=AXIS2_PLACEMENT_3D ( 'NONE', #19954, #7499, #14553 ) ;
#29243=DIRECTION ( 'NONE',  ( 0.9612616959383193382, 0.2756373558169973870, 8.795445018804928853E-19 ) ) ;
#29249=CARTESIAN_POINT ( 'NONE',  ( -40.60333149162104860, 7.557375771971046596, 58.05249952744806308 ) ) ;
#29253=EDGE_LOOP ( 'NONE', ( #23945, #19761, #22806, #32334, #13409 ) ) ;
#29255=VECTOR ( 'NONE', #30749, 1000.000000000000114 ) ;
#29259=LINE ( 'NONE', #26634, #13509 ) ;
#29261=AXIS2_PLACEMENT_3D ( 'NONE', #22884, #5174, #30609 ) ;
#29263=ORIENTED_EDGE ( 'NONE', *, *, #10129, .F. ) ;
#29266=AXIS2_PLACEMENT_3D ( 'NONE', #21107, #6506, #31142 ) ;
#29269=DIRECTION ( 'NONE',  ( 0.8746197071393926326, -0.4848096202463430537, -8.676864087101709653E-18 ) ) ;
#29272=ADVANCED_FACE ( 'NONE', ( #9161 ), #12121, .T. ) ;
#29276=ORIENTED_EDGE ( 'NONE', *, *, #15668, .T. ) ;
#29277=CARTESIAN_POINT ( 'NONE',  ( -41.10400476907452116, 9.333823787025622210, 39.43215070697513625 ) ) ;
#29280=EDGE_CURVE ( 'NONE', #607, #12276, #19157, .T. ) ;
#29282=AXIS2_PLACEMENT_3D ( 'NONE', #17908, #27, #2808 ) ;
#29284=VECTOR ( 'NONE', #30574, 1000.000000000000227 ) ;
#29285=CARTESIAN_POINT ( 'NONE',  ( -42.24141723705587737, 13.63285518870473290, 59.54930799450050927 ) ) ;
#29287=CARTESIAN_POINT ( 'NONE',  ( -42.66751614955960292, 15.14923148629343963, 35.64930799450052490 ) ) ;
#29291=EDGE_LOOP ( 'NONE', ( #32267, #18569, #11649, #10479, #21730, #9107 ) ) ;
#29297=PLANE ( 'NONE',  #799 ) ;
#29298=CARTESIAN_POINT ( 'NONE',  ( -43.64073206722599707, 1.267352857069779848, 39.44930799450052916 ) ) ;
#29302=CARTESIAN_POINT ( 'NONE',  ( -40.18117225532238024, 7.056010640735429718, 34.94364560924564245 ) ) ;
#29305=CARTESIAN_POINT ( 'NONE',  ( -40.19935072163751499, 7.013056605096608109, 34.87232122021060832 ) ) ;
#29311=AXIS2_PLACEMENT_3D ( 'NONE', #6880, #22401, #16877 ) ;
#29312=DIRECTION ( 'NONE',  ( 0.4848096202463430537, 0.8746197071393926326, 1.323854077651070671E-16 ) ) ;
#29313=ADVANCED_FACE ( 'NONE', ( #3909 ), #13934, .F. ) ;
#29315=ORIENTED_EDGE ( 'NONE', *, *, #8023, .T. ) ;
#29319=FACE_OUTER_BOUND ( 'NONE', #19307, .T. ) ;
#29320=VECTOR ( 'NONE', #32449, 1000.000000000000114 ) ;
#29323=ORIENTED_EDGE ( 'NONE', *, *, #24799, .F. ) ;
#29327=CARTESIAN_POINT ( 'NONE',  ( -40.50730207061041455, 7.560184202955509747, 53.81891027488745749 ) ) ;
#29346=ORIENTED_EDGE ( 'NONE', *, *, #26871, .F. ) ;
#29348=AXIS2_PLACEMENT_3D ( 'NONE', #569, #17642, #10914 ) ;
#29349=DIRECTION ( 'NONE',  ( -0.9612616959383205595, -0.2756373558169931681, 1.660411357259282445E-16 ) ) ;
#29354=CARTESIAN_POINT ( 'NONE',  ( -40.02540636251513462, 2.839176264122874382, 38.34930799450052064 ) ) ;
#29356=LINE ( 'NONE', #16545, #3034 ) ;
#29357=ORIENTED_EDGE ( 'NONE', *, *, #11473, .T. ) ;
#29359=DIRECTION ( 'NONE',  ( 1.188208965918165239E-16, 1.880121038077813132E-16, 1.000000000000000000 ) ) ;
#29363=VECTOR ( 'NONE', #18379, 1000.000000000000000 ) ;
#29366=AXIS2_PLACEMENT_3D ( 'NONE', #2081, #12765, #271 ) ;
#29376=ORIENTED_EDGE ( 'NONE', *, *, #18488, .T. ) ;
#29387=DIRECTION ( 'NONE',  ( 0.9612616959383194493, 0.2756373558169974980, 8.795445018804946186E-19 ) ) ;
#29389=ADVANCED_FACE ( 'NONE', ( #5216, #25072, #22604, #25395 ), #20296, .T. ) ;
#29391=EDGE_CURVE ( 'NONE', #2410, #12082, #29413, .T. ) ;
#29397=VECTOR ( 'NONE', #30363, 999.9999999999998863 ) ;
#29399=EDGE_CURVE ( 'NONE', #10259, #25118, #30993, .T. ) ;
#29402=AXIS2_PLACEMENT_3D ( 'NONE', #6163, #24365, #9273 ) ;
#29405=CARTESIAN_POINT ( 'NONE',  ( -39.52978099598376360, 7.652372239361225681, 61.99930799450051921 ) ) ;
#29407=ORIENTED_EDGE ( 'NONE', *, *, #20924, .F. ) ;
#29409=CARTESIAN_POINT ( 'NONE',  ( -43.86882709718853590, -0.1754741395363378920, 32.14930799450051779 ) ) ;
#29413=CIRCLE ( 'NONE', #577, 1.500000000000001332 ) ;
#29417=EDGE_CURVE ( 'NONE', #3387, #10451, #1454, .T. ) ;
#29423=DIRECTION ( 'NONE',  ( -2.779292025043186357E-18, 1.288349127009862211E-17, -1.000000000000000000 ) ) ;
#29424=DIRECTION ( 'NONE',  ( -0.2756373558170018279, 0.9612616959383181170, 0.000000000000000000 ) ) ;
#29429=AXIS2_PLACEMENT_3D ( 'NONE', #22836, #15455, #10543 ) ;
#29432=EDGE_CURVE ( 'NONE', #12894, #18455, #2687, .T. ) ;
#29438=LINE ( 'NONE', #19410, #21669 ) ;
#29442=ADVANCED_FACE ( 'NONE', ( #22429 ), #15272, .T. ) ;
#29450=ORIENTED_EDGE ( 'NONE', *, *, #19782, .F. ) ;
#29453=DIRECTION ( 'NONE',  ( -0.4848096202463429982, -0.8746197071393925215, -9.920727850371698576E-18 ) ) ;
#29455=EDGE_CURVE ( 'NONE', #22939, #3679, #5384, .T. ) ;
#29458=CARTESIAN_POINT ( 'NONE',  ( -40.08841711228579641, 7.575633567407562552, 60.29072935073781991 ) ) ;
#29461=EDGE_CURVE ( 'NONE', #12291, #3439, #10471, .T. ) ;
#29464=ORIENTED_EDGE ( 'NONE', *, *, #12386, .T. ) ;
#29466=CIRCLE ( 'NONE', #10082, 1.624998423334081066 ) ;
#29469=ORIENTED_EDGE ( 'NONE', *, *, #25671, .T. ) ;
#29472=CARTESIAN_POINT ( 'NONE',  ( -43.68921302925062378, 1.179890886355840163, 39.44930799450052916 ) ) ;
#29474=CARTESIAN_POINT ( 'NONE',  ( -40.46271621608484281, 3.081581074246047880, 37.04930799450052348 ) ) ;
#29480=EDGE_CURVE ( 'NONE', #16381, #382, #5056, .T. ) ;
#29485=ORIENTED_EDGE ( 'NONE', *, *, #24457, .F. ) ;
#29497=ORIENTED_EDGE ( 'NONE', *, *, #6752, .T. ) ;
#29499=DIRECTION ( 'NONE',  ( 0.9612616959383221138, 0.2756373558169876170, 0.000000000000000000 ) ) ;
#29504=DIRECTION ( 'NONE',  ( 0.4848096202463429982, 0.8746197071393925215, 9.920727850371698576E-18 ) ) ;
#29509=ORIENTED_EDGE ( 'NONE', *, *, #3614, .F. ) ;
#29510=DIRECTION ( 'NONE',  ( 0.2756373558170082672, -0.9612616959383162296, 0.000000000000000000 ) ) ;
#29530=VERTEX_POINT ( 'NONE', #15703 ) ;
#29540=CYLINDRICAL_SURFACE ( 'NONE', #10520, 0.1000000000000028644 ) ;
#29545=LINE ( 'NONE', #9518, #25446 ) ;
#29550=ORIENTED_EDGE ( 'NONE', *, *, #15084, .F. ) ;
#29560=CARTESIAN_POINT ( 'NONE',  ( -41.04685960816998147, 9.497330455345890599, 35.54930799450052348 ) ) ;
#29563=ORIENTED_EDGE ( 'NONE', *, *, #21181, .T. ) ;
#29567=VERTEX_POINT ( 'NONE', #18319 ) ;
#29568=CARTESIAN_POINT ( 'NONE',  ( -40.06561427811386267, 7.496110634155836117, 58.05249952744806308 ) ) ;
#29574=CARTESIAN_POINT ( 'NONE',  ( -39.37937466094673766, 7.181451953876404559, 39.54930799450052348 ) ) ;
#29580=CARTESIAN_POINT ( 'NONE',  ( -40.65093765668705572, 9.567768634527945792, 35.64930799450052490 ) ) ;
#29582=DIRECTION ( 'NONE',  ( 0.2250569586005206069, -0.7848668881104323702, 0.5773502691896226224 ) ) ;
#29598=CARTESIAN_POINT ( 'NONE',  ( -40.06561427811386267, 7.496110634155836117, 60.44930799450051495 ) ) ;
#29602=CARTESIAN_POINT ( 'NONE',  ( -40.12425944110432852, 6.890664497466326921, 39.53069180094396984 ) ) ;
#29604=CARTESIAN_POINT ( 'NONE',  ( -42.59697395963048194, 14.54042610638008526, 37.04930799450052348 ) ) ;
#29606=VECTOR ( 'NONE', #15432, 1000.000000000000000 ) ;
#29609=CIRCLE ( 'NONE', #15445, 0.09999999999999795164 ) ;
#29618=DIRECTION ( 'NONE',  ( 0.2756373558169971649, -0.9612616959383194493, 0.000000000000000000 ) ) ;
#29621=EDGE_CURVE ( 'NONE', #13895, #1905, #596, .T. ) ;
#29624=VERTEX_POINT ( 'NONE', #5873 ) ;
#29626=ORIENTED_EDGE ( 'NONE', *, *, #8234, .T. ) ;
#29644=ORIENTED_EDGE ( 'NONE', *, *, #21783, .T. ) ;
#29645=CIRCLE ( 'NONE', #2906, 1.199999999999999734 ) ;
#29647=AXIS2_PLACEMENT_3D ( 'NONE', #1436, #8995, #6692 ) ;
#29654=B_SPLINE_CURVE_WITH_KNOTS ( 'NONE', 3,
 ( #30884, #15939, #1155, #11183, #21167, #5774, #31206, #18703 ),
 .UNSPECIFIED., .F., .F.,
 ( 4, 2, 2, 4 ),
 ( 0.000000000000000000, 4.692856542812975473E-05, 7.039284814219625840E-05, 9.385713085626276207E-05 ),
 .UNSPECIFIED. ) ;
#29664=VERTEX_POINT ( 'NONE', #16342 ) ;
#29668=VECTOR ( 'NONE', #12489, 1000.000000000000000 ) ;
#29669=CARTESIAN_POINT ( 'NONE',  ( -39.50554051497144314, 7.696103224718195968, 32.14930799450051779 ) ) ;
#29671=EDGE_LOOP ( 'NONE', ( #1615, #13040, #15861, #11740 ) ) ;
#29673=CARTESIAN_POINT ( 'NONE',  ( -41.08785830660042393, 9.277514380576530328, 35.49072935073782986 ) ) ;
#29674=DIRECTION ( 'NONE',  ( -1.188208965918165239E-16, -1.880121038077813132E-16, -1.000000000000000000 ) ) ;
#29686=CYLINDRICAL_SURFACE ( 'NONE', #14803, 0.9031915329475500576 ) ;
#29692=ADVANCED_FACE ( 'NONE', ( #4199 ), #27965, .T. ) ;
#29694=VERTEX_POINT ( 'NONE', #11908 ) ;
#29695=AXIS2_PLACEMENT_3D ( 'NONE', #9322, #23931, #31659 ) ;
#29703=DIRECTION ( 'NONE',  ( 0.8746197071393926326, -0.4848096202463430537, -8.676864087101709653E-18 ) ) ;
#29704=DIRECTION ( 'NONE',  ( -2.779292025043186357E-18, 1.288349127009862211E-17, -1.000000000000000000 ) ) ;
#29706=ORIENTED_EDGE ( 'NONE', *, *, #24466, .T. ) ;
#29708=DIRECTION ( 'NONE',  ( -0.8746197071393926326, 0.4848096202463430537, 8.676864087101709653E-18 ) ) ;
#29710=FACE_OUTER_BOUND ( 'NONE', #12635, .T. ) ;
#29711=DIRECTION ( 'NONE',  ( 0.8746197071393926326, -0.4848096202463430537, -8.676864087101709653E-18 ) ) ;
#29725=CARTESIAN_POINT ( 'NONE',  ( -43.95628906790246759, -0.1269931775117038586, 61.94930799450052206 ) ) ;
#29731=PLANE ( 'NONE',  #2862 ) ;
#29734=VERTEX_POINT ( 'NONE', #17481 ) ;
#29735=PLANE ( 'NONE',  #30130 ) ;
#29740=CIRCLE ( 'NONE', #17690, 0.8999999999999983569 ) ;
#29742=CARTESIAN_POINT ( 'NONE',  ( -42.37913764077812573, 15.23192269303852875, 35.64930799450052490 ) ) ;
#29751=CARTESIAN_POINT ( 'NONE',  ( -41.07560527903737579, 9.385057823277966449, 34.64930799450051779 ) ) ;
#29753=ORIENTED_EDGE ( 'NONE', *, *, #17254, .T. ) ;
#29762=ORIENTED_EDGE ( 'NONE', *, *, #20757, .F. ) ;
#29764=CARTESIAN_POINT ( 'NONE',  ( -40.11027759654395197, 6.823245743731469304, 39.47270689035109115 ) ) ;
#29766=CARTESIAN_POINT ( 'NONE',  ( -40.18454328187963398, 7.548069831825862330, 60.44930799450051495 ) ) ;
#29784=CARTESIAN_POINT ( 'NONE',  ( -40.84548646114599535, 8.466718295361152613, 34.60485935866290674 ) ) ;
#29785=ORIENTED_EDGE ( 'NONE', *, *, #15044, .F. ) ;
#29788=( BOUNDED_CURVE ( )  B_SPLINE_CURVE ( 3, ( #20451, #28174, #912, #5859 ),
 .UNSPECIFIED., .F., .F. ) 
 B_SPLINE_CURVE_WITH_KNOTS ( ( 4, 4 ),
 ( 4.712388980384698556, 5.497787143782109531 ),
 .UNSPECIFIED. ) 
 CURVE ( )  GEOMETRIC_REPRESENTATION_ITEM ( )  RATIONAL_B_SPLINE_CURVE ( ( 1.000000000000000000, 0.9492530216741960070, 0.9492530216741960070, 1.000000000000000000 ) ) 
 REPRESENTATION_ITEM ( '' )  );
#29790=CARTESIAN_POINT ( 'NONE',  ( -41.56459318755936749, 7.281738416154046156, 60.54930799450051637 ) ) ;
#29798=AXIS2_PLACEMENT_3D ( 'NONE', #29742, #7585, #25139 ) ;
#29799=LINE ( 'NONE', #25030, #6884 ) ;
#29802=CYLINDRICAL_SURFACE ( 'NONE', #27445, 0.9031915329475500576 ) ;
#29822=ORIENTED_EDGE ( 'NONE', *, *, #12262, .T. ) ;
#29830=ORIENTED_EDGE ( 'NONE', *, *, #17900, .T. ) ;
#29831=DIRECTION ( 'NONE',  ( 0.8746197071393925215, -0.4848096202463429982, -8.676864087101708112E-18 ) ) ;
#29837=CARTESIAN_POINT ( 'NONE',  ( -40.69193635511749108, 9.347952559758585522, 39.44930799450052206 ) ) ;
#29838=AXIS2_PLACEMENT_3D ( 'NONE', #19946, #29977, #17493 ) ;
#29839=DIRECTION ( 'NONE',  ( -1.188208965918165239E-16, -1.880121038077813132E-16, -1.000000000000000000 ) ) ;
#29846=CARTESIAN_POINT ( 'NONE',  ( -40.23967075304302909, 7.740322171013528596, 53.80788663826320573 ) ) ;
#29848=EDGE_LOOP ( 'NONE', ( #6127, #8171, #18169, #21511 ) ) ;
#29855=ORIENTED_EDGE ( 'NONE', *, *, #589, .F. ) ;
#29856=PLANE ( 'NONE',  #22521 ) ;
#29864=EDGE_CURVE ( 'NONE', #31848, #27545, #1643, .T. ) ;
#29865=AXIS2_PLACEMENT_3D ( 'NONE', #27053, #32150, #7365 ) ;
#29867=CIRCLE ( 'NONE', #24088, 0.1000000000000008660 ) ;
#29873=EDGE_LOOP ( 'NONE', ( #28685, #32163, #14130, #32002 ) ) ;
#29875=EDGE_CURVE ( 'NONE', #16357, #9876, #24206, .T. ) ;
#29879=CARTESIAN_POINT ( 'NONE',  ( -40.23847960489091236, 6.935107575317837281, 34.54930799450052348 ) ) ;
#29885=VECTOR ( 'NONE', #9602, 1000.000000000000000 ) ;
#29892=CARTESIAN_POINT ( 'NONE',  ( -40.99173213700658636, 9.305078116158229662, 39.54930799450052348 ) ) ;
#29895=AXIS2_PLACEMENT_3D ( 'NONE', #27896, #25585, #20500 ) ;
#29900=AXIS2_PLACEMENT_3D ( 'NONE', #29068, #6589, #18560 ) ;
#29903=ADVANCED_FACE ( 'NONE', ( #11076 ), #17391, .T. ) ;
#29908=EDGE_CURVE ( 'NONE', #9365, #9700, #3514, .T. ) ;
#29922=CIRCLE ( 'NONE', #25180, 0.1000000000000018235 ) ;
#29927=CARTESIAN_POINT ( 'NONE',  ( -40.02540636251514172, 2.839176264122877047, 57.04930799450051637 ) ) ;
#29936=CARTESIAN_POINT ( 'NONE',  ( -40.16409007829387434, 6.927803014773068924, 39.54930799450049506 ) ) ;
#29938=AXIS2_PLACEMENT_3D ( 'NONE', #24081, #19312, #14086 ) ;
#29950=DIRECTION ( 'NONE',  ( -0.9612616959383200044, -0.2756373558169954996, 1.660411357259285896E-16 ) ) ;
#29951=CARTESIAN_POINT ( 'NONE',  ( -40.32034427004700916, 8.384459687302960873, 54.44930799450051495 ) ) ;
#29955=CARTESIAN_POINT ( 'NONE',  ( -40.78689554741473700, 8.436943771353742960, 34.55838508629864947 ) ) ;
#29956=EDGE_LOOP ( 'NONE', ( #311, #1379, #32188, #3948 ) ) ;
#29961=ORIENTED_EDGE ( 'NONE', *, *, #20609, .F. ) ;
#29963=DIRECTION ( 'NONE',  ( 0.4848096202463645921, 0.8746197071393805311, 0.000000000000000000 ) ) ;
#29964=FACE_OUTER_BOUND ( 'NONE', #2576, .T. ) ;
#29971=CARTESIAN_POINT ( 'NONE',  ( -42.37913764077812573, 15.23192269303853053, 38.44930799450052206 ) ) ;
#29977=DIRECTION ( 'NONE',  ( -0.4848096202463430537, -0.8746197071393926326, -9.920727850371700117E-18 ) ) ;
#29980=AXIS2_PLACEMENT_3D ( 'NONE', #20504, #23132, #12652 ) ;
#29984=ORIENTED_EDGE ( 'NONE', *, *, #24798, .F. ) ;
#29985=ORIENTED_EDGE ( 'NONE', *, *, #15966, .F. ) ;
#29987=ADVANCED_FACE ( 'NONE', ( #20749 ), #19499, .T. ) ;
#29996=ORIENTED_EDGE ( 'NONE', *, *, #30400, .T. ) ;
#29999=AXIS2_PLACEMENT_3D ( 'NONE', #2220, #25513, #12565 ) ;
#30000=ORIENTED_EDGE ( 'NONE', *, *, #17817, .T. ) ;
#30001=CYLINDRICAL_SURFACE ( 'NONE', #32078, 0.1000000000000006301 ) ;
#30002=CARTESIAN_POINT ( 'NONE',  ( -40.65487266620045403, 9.475231293617264683, 39.54930799450052348 ) ) ;
#30005=DIRECTION ( 'NONE',  ( -2.779292025043186357E-18, 1.288349127009862211E-17, -1.000000000000000000 ) ) ;
#30008=DIRECTION ( 'NONE',  ( -0.8746197071393926326, 0.4848096202463430537, 8.676864087101709653E-18 ) ) ;
#30010=ORIENTED_EDGE ( 'NONE', *, *, #25684, .T. ) ;
#30012=ORIENTED_EDGE ( 'NONE', *, *, #26162, .F. ) ;
#30014=CARTESIAN_POINT ( 'NONE',  ( -40.05987053574653345, 7.506472619680472746, 39.54930799450052348 ) ) ;
#30017=VERTEX_POINT ( 'NONE', #1693 ) ;
#30018=LINE ( 'NONE', #17531, #9409 ) ;
#30026=CIRCLE ( 'NONE', #23198, 0.1000000000000008243 ) ;
#30035=EDGE_CURVE ( 'NONE', #19824, #3250, #15831, .T. ) ;
#30040=ORIENTED_EDGE ( 'NONE', *, *, #12683, .F. ) ;
#30044=CARTESIAN_POINT ( 'NONE',  ( -40.61178118339597631, 9.038025460530262123, 57.04930799450051637 ) ) ;
#30045=DIRECTION ( 'NONE',  ( -2.779292025043186357E-18, 1.288349127009862211E-17, -1.000000000000000000 ) ) ;
#30049=DIRECTION ( 'NONE',  ( 0.2756373558169947779, -0.9612616959383200044, 0.000000000000000000 ) ) ;
#30053=VERTEX_POINT ( 'NONE', #3832 ) ;
#30055=VECTOR ( 'NONE', #3896, 1000.000000000000000 ) ;
#30062=EDGE_CURVE ( 'NONE', #30210, #7068, #1666, .T. ) ;
#30071=SPHERICAL_SURFACE ( 'NONE', #22975, 0.1000000000000000056 ) ;
#30079=CYLINDRICAL_SURFACE ( 'NONE', #13308, 0.1000000000000010325 ) ;
#30085=FACE_OUTER_BOUND ( 'NONE', #14548, .T. ) ;
#30096=CARTESIAN_POINT ( 'NONE',  ( -40.16503835899720087, 7.510440877657823755, 38.80028690913362510 ) ) ;
#30104=EDGE_CURVE ( 'NONE', #10889, #286, #29466, .T. ) ;
#30107=EDGE_CURVE ( 'NONE', #21817, #13209, #4686, .T. ) ;
#30110=EDGE_CURVE ( 'NONE', #20495, #29138, #28412, .T. ) ;
#30112=CARTESIAN_POINT ( 'NONE',  ( -42.59587854516874472, -0.7667456371672795035, 61.94930799450052206 ) ) ;
#30117=ORIENTED_EDGE ( 'NONE', *, *, #24553, .T. ) ;
#30120=TOROIDAL_SURFACE ( 'NONE', #1255, 1.299999999999999822, 0.1000000000000000056 ) ;
#30121=CARTESIAN_POINT ( 'NONE',  ( -43.38408989745150990, 1.111547985471240452, 60.44930799450051495 ) ) ;
#30123=CARTESIAN_POINT ( 'NONE',  ( -40.69573679811334443, 6.786506765454743295, 39.45085645659242601 ) ) ;
#30124=ORIENTED_EDGE ( 'NONE', *, *, #27873, .F. ) ;
#30130=AXIS2_PLACEMENT_3D ( 'NONE', #29409, #3971, #1668 ) ;
#30134=CARTESIAN_POINT ( 'NONE',  ( -42.22138300640814634, 14.68176690255379491, 37.04930799450052348 ) ) ;
#30138=EDGE_CURVE ( 'NONE', #9841, #9952, #12373, .T. ) ;
#30141=CARTESIAN_POINT ( 'NONE',  ( -40.02540636251514172, 2.839176264122877047, 55.04930799450051637 ) ) ;
#30143=ADVANCED_FACE ( 'NONE', ( #10071 ), #17604, .F. ) ;
#30146=CIRCLE ( 'NONE', #1826, 1.003191532947548925 ) ;
#30148=AXIS2_PLACEMENT_3D ( 'NONE', #5690, #21092, #15693 ) ;
#30153=ORIENTED_EDGE ( 'NONE', *, *, #17853, .T. ) ;
#30156=DIRECTION ( 'NONE',  ( -0.9612616959383204485, -0.2756373558169933347, 1.660411357259282692E-16 ) ) ;
#30157=CARTESIAN_POINT ( 'NONE',  ( -40.46271621608484281, 3.081581074246049212, 57.04930799450051637 ) ) ;
#30161=EDGE_LOOP ( 'NONE', ( #13423, #27711, #3179, #18148 ) ) ;
#30167=CARTESIAN_POINT ( 'NONE',  ( -40.32034427004700916, 8.384459687302960873, 59.54930799450050927 ) ) ;
#30172=CARTESIAN_POINT ( 'NONE',  ( -40.05987053574653345, 7.506472619680471858, 35.39279590939684539 ) ) ;
#30179=CARTESIAN_POINT ( 'NONE',  ( -42.59587854516874472, -0.7667456371672803916, 32.14930799450051779 ) ) ;
#30181=EDGE_LOOP ( 'NONE', ( #6319, #26730, #9797, #19541, #4512, #31303 ) ) ;
#30182=DIRECTION ( 'NONE',  ( 0.8746197071393858602, -0.4848096202463547666, 0.000000000000000000 ) ) ;
#30188=AXIS2_PLACEMENT_3D ( 'NONE', #5010, #25666, #12561 ) ;
#30192=DIRECTION ( 'NONE',  ( 0.8746197071393926326, -0.4848096202463430537, -8.676864087101709653E-18 ) ) ;
#30194=VERTEX_POINT ( 'NONE', #211 ) ;
#30206=VERTEX_POINT ( 'NONE', #12034 ) ;
#30207=DIRECTION ( 'NONE',  ( 0.9612616959383221138, 0.2756373558169876170, 0.000000000000000000 ) ) ;
#30208=DIRECTION ( 'NONE',  ( 0.000000000000000000, 0.000000000000000000, 1.000000000000000000 ) ) ;
#30210=VERTEX_POINT ( 'NONE', #22360 ) ;
#30213=CARTESIAN_POINT ( 'NONE',  ( -42.36153388572594736, 13.68895619636815653, 59.44930799450051495 ) ) ;
#30225=DIRECTION ( 'NONE',  ( -0.8746197071393805311, 0.4848096202463645921, 1.277302113040265530E-17 ) ) ;
#30226=CARTESIAN_POINT ( 'NONE',  ( -41.94956971822180947, 3.905757428664828890, 48.34930799450052064 ) ) ;
#30232=AXIS2_PLACEMENT_3D ( 'NONE', #22151, #20183, #30207 ) ;
#30233=CARTESIAN_POINT ( 'NONE',  ( -36.51523247376623971, 9.273102258352469818, 57.04930799450051637 ) ) ;
#30236=CARTESIAN_POINT ( 'NONE',  ( -40.60330327974817521, 7.565477138576668814, 60.21714911875709220 ) ) ;
#30240=DIRECTION ( 'NONE',  ( 0.1949050434465267045, -0.6797146636928664831, -0.7071067811865482389 ) ) ;
#30246=LINE ( 'NONE', #22514, #29284 ) ;
#30247=DIRECTION ( 'NONE',  ( 0.4848096202463636484, 0.8746197071393810862, 0.000000000000000000 ) ) ;
#30252=DIRECTION ( 'NONE',  ( -0.8746197071393840838, 0.4848096202463581528, 0.000000000000000000 ) ) ;
#30254=ORIENTED_EDGE ( 'NONE', *, *, #13229, .F. ) ;
#30261=ADVANCED_FACE ( 'NONE', ( #25159 ), #24726, .T. ) ;
#30267=DIRECTION ( 'NONE',  ( 0.4848096202463429982, 0.8746197071393925215, 9.920727850371698576E-18 ) ) ;
#30271=CARTESIAN_POINT ( 'NONE',  ( -40.76990606341588830, 8.436069916073961394, 34.55282792453324703 ) ) ;
#30272=ORIENTED_EDGE ( 'NONE', *, *, #23456, .T. ) ;
#30277=DIRECTION ( 'NONE',  ( -0.4848096202463429982, -0.8746197071393925215, -9.920727850371698576E-18 ) ) ;
#30279=ADVANCED_FACE ( 'NONE', ( #11465 ), #19512, .T. ) ;
#30284=DIRECTION ( 'NONE',  ( -0.9612616959383194493, -0.2756373558169972759, -8.795445018804905742E-19 ) ) ;
#30285=CARTESIAN_POINT ( 'NONE',  ( -40.76967387488526384, 8.530668925462080665, 39.44930799450052206 ) ) ;
#30293=CARTESIAN_POINT ( 'NONE',  ( -42.47434154250543514, 4.196643200812633978, 37.04930799450052348 ) ) ;
#30299=ORIENTED_EDGE ( 'NONE', *, *, #8744, .F. ) ;
#30300=VECTOR ( 'NONE', #13140, 999.9999999999998863 ) ;
#30301=AXIS2_PLACEMENT_3D ( 'NONE', #5036, #15043, #12261 ) ;
#30304=EDGE_CURVE ( 'NONE', #23287, #22939, #22660, .T. ) ;
#30305=CARTESIAN_POINT ( 'NONE',  ( -41.01929587258828747, 9.401204285752058354, 34.64930799450051779 ) ) ;
#30312=DIRECTION ( 'NONE',  ( -0.8746197071393926326, 0.4848096202463430537, 8.676864087101709653E-18 ) ) ;
#30319=CARTESIAN_POINT ( 'NONE',  ( -43.86882709718853590, -0.1754741395363378920, 32.14930799450051779 ) ) ;
#30325=CARTESIAN_POINT ( 'NONE',  ( -41.56459318755936749, 7.281738416154046156, 53.64930799450051779 ) ) ;
#30329=CARTESIAN_POINT ( 'NONE',  ( -36.30817626167056744, 11.56595247146531946, 37.04930799450052348 ) ) ;
#30330=EDGE_LOOP ( 'NONE', ( #29830, #28794, #26277, #11833 ) ) ;
#30343=EDGE_LOOP ( 'NONE', ( #28834, #14981, #31001 ) ) ;
#30346=AXIS2_PLACEMENT_3D ( 'NONE', #1588, #4541, #31955 ) ;
#30351=LINE ( 'NONE', #10169, #791 ) ;
#30356=DIRECTION ( 'NONE',  ( 0.000000000000000000, 0.000000000000000000, 1.000000000000000000 ) ) ;
#30363=DIRECTION ( 'NONE',  ( 0.9612616959383207815, 0.2756373558169926685, 8.795445018804289444E-19 ) ) ;
#30364=CARTESIAN_POINT ( 'NONE',  ( -42.26497471389478733, 14.66834543456874940, 60.54930799450051637 ) ) ;
#30372=CARTESIAN_POINT ( 'NONE',  ( -43.37834615508418068, 1.121909970995875971, 34.54930799450052348 ) ) ;
#30373=CARTESIAN_POINT ( 'NONE',  ( -42.73182147790732444, -0.8057266458565844891, 61.94930799450052206 ) ) ;
#30375=AXIS2_PLACEMENT_3D ( 'NONE', #13230, #25680, #8132 ) ;
#30382=DIRECTION ( 'NONE',  ( -7.588956326749211550E-18, 4.206627182996912454E-18, -1.000000000000000000 ) ) ;
#30383=DIRECTION ( 'NONE',  ( -0.4848096202463430537, -0.8746197071393926326, -9.920727850371701658E-18 ) ) ;
#30386=DIRECTION ( 'NONE',  ( 0.4848096202463673676, 0.8746197071393789768, 0.000000000000000000 ) ) ;
#30387=CYLINDRICAL_SURFACE ( 'NONE', #3907, 0.1000000000000018235 ) ;
#30394=LINE ( 'NONE', #20695, #3397 ) ;
#30396=ADVANCED_FACE ( 'NONE', ( #14584 ), #29686, .F. ) ;
#30400=EDGE_CURVE ( 'NONE', #21242, #27995, #9500, .T. ) ;
#30404=ORIENTED_EDGE ( 'NONE', *, *, #18518, .T. ) ;
#30411=DIRECTION ( 'NONE',  ( -0.9612616959383204485, -0.2756373558169933347, 1.660411357259282692E-16 ) ) ;
#30416=CARTESIAN_POINT ( 'NONE',  ( -40.01196617103988018, 7.363926680072800046, 38.86384274482242063 ) ) ;
#30425=VECTOR ( 'NONE', #4140, 1000.000000000000114 ) ;
#30433=CARTESIAN_POINT ( 'NONE',  ( -40.02540636251514172, 2.839176264122877047, 55.14930799450051779 ) ) ;
#30434=CARTESIAN_POINT ( 'NONE',  ( -41.01929587258828036, 9.401204285752060130, 38.64930799450052490 ) ) ;
#30436=AXIS2_PLACEMENT_3D ( 'NONE', #19043, #28744, #23501 ) ;
#30442=LINE ( 'NONE', #5333, #14678 ) ;
#30453=CARTESIAN_POINT ( 'NONE',  ( -40.49360782792987834, 7.147293204394356891, 38.94271047082367687 ) ) ;
#30457=DIRECTION ( 'NONE',  ( -0.4848096202463431648, -0.8746197071393924105, 0.000000000000000000 ) ) ;
#30460=AXIS2_PLACEMENT_3D ( 'NONE', #14902, #29839, #24910 ) ;
#30466=ORIENTED_EDGE ( 'NONE', *, *, #9865, .T. ) ;
#30468=AXIS2_PLACEMENT_3D ( 'NONE', #1855, #9406, #16940 ) ;
#30469=EDGE_LOOP ( 'NONE', ( #5011, #27423 ) ) ;
#30473=DIRECTION ( 'NONE',  ( -0.7141240004913222972, 0.3958453973320028019, -0.5773502691896303940 ) ) ;
#30490=AXIS2_PLACEMENT_3D ( 'NONE', #9489, #6864, #31968 ) ;
#30491=EDGE_LOOP ( 'NONE', ( #4166, #249 ) ) ;
#30497=CARTESIAN_POINT ( 'NONE',  ( -40.01185171578377719, 7.339011093366132776, 35.33835236764744536 ) ) ;
#30499=ORIENTED_EDGE ( 'NONE', *, *, #13205, .T. ) ;
#30508=( GEOMETRIC_REPRESENTATION_CONTEXT ( 3 ) GLOBAL_UNCERTAINTY_ASSIGNED_CONTEXT ( ( #23907 ) ) GLOBAL_UNIT_ASSIGNED_CONTEXT ( ( #18947, #1555, #1726 ) ) REPRESENTATION_CONTEXT ( 'NONE', 'WORKASPACE' ) );
#30516=AXIS2_PLACEMENT_3D ( 'NONE', #4193, #21256, #9115 ) ;
#30524=ORIENTED_EDGE ( 'NONE', *, *, #27262, .F. ) ;
#30529=DIRECTION ( 'NONE',  ( -0.2756373558169942228, 0.9612616959383203374, 0.000000000000000000 ) ) ;
#30535=CARTESIAN_POINT ( 'NONE',  ( -40.60251150970604073, 6.748447833883063574, 53.54930799450051637 ) ) ;
#30537=CARTESIAN_POINT ( 'NONE',  ( -40.28779227465695811, 2.984619150196779813, 57.04930799450051637 ) ) ;
#30539=EDGE_CURVE ( 'NONE', #19419, #12604, #28440, .T. ) ;
#30540=ORIENTED_EDGE ( 'NONE', *, *, #25354, .F. ) ;
#30542=DIRECTION ( 'NONE',  ( -0.9612616959383198934, -0.2756373558169956106, 0.000000000000000000 ) ) ;
#30543=EDGE_CURVE ( 'NONE', #24828, #16797, #25808, .T. ) ;
#30547=EDGE_CURVE ( 'NONE', #18622, #21242, #32116, .T. ) ;
#30553=CARTESIAN_POINT ( 'NONE',  ( -39.67555847965937943, 2.645252416024337361, 48.34930799450052064 ) ) ;
#30557=CARTESIAN_POINT ( 'NONE',  ( -42.85109120870324517, 14.58887732880157273, 55.18058063134417779 ) ) ;
#30560=CARTESIAN_POINT ( 'NONE',  ( -40.34207605779958072, 7.502898035225042506, 60.54930799450051637 ) ) ;
#30561=CARTESIAN_POINT ( 'NONE',  ( -40.06561427811386267, 7.496110634155836117, 53.64930799450051779 ) ) ;
#30563=LINE ( 'NONE', #30724, #27390 ) ;
#30566=AXIS2_PLACEMENT_3D ( 'NONE', #4393, #11625, #1925 ) ;
#30568=CARTESIAN_POINT ( 'NONE',  ( -39.59300248568538194, 7.744584186742828891, 62.04930799450052348 ) ) ;
#30572=VERTEX_POINT ( 'NONE', #12788 ) ;
#30574=DIRECTION ( 'NONE',  ( -0.2756373558169954441, 0.9612616959383198934, -1.479773560108263204E-16 ) ) ;
#30576=EDGE_LOOP ( 'NONE', ( #18539, #1792, #16579, #29407 ) ) ;
#30588=ADVANCED_FACE ( 'NONE', ( #136 ), #7850, .F. ) ;
#30600=ORIENTED_EDGE ( 'NONE', *, *, #2850, .F. ) ;
#30605=CARTESIAN_POINT ( 'NONE',  ( -37.68353499307994525, 12.01442086639228712, 60.54930799450051637 ) ) ;
#30608=DIRECTION ( 'NONE',  ( -0.3958453973320076313, -0.7141240004913228523, 0.5773502691896265082 ) ) ;
#30609=DIRECTION ( 'NONE',  ( 0.4848096202463424986, 0.8746197071393928546, -2.220446049250312834E-16 ) ) ;
#30616=CARTESIAN_POINT ( 'NONE',  ( -40.59298576501943501, 7.024321269945732027, 38.94336021962444505 ) ) ;
#30618=EDGE_LOOP ( 'NONE', ( #28431, #22461, #16727, #26493 ) ) ;
#30619=FACE_OUTER_BOUND ( 'NONE', #29253, .T. ) ;
#30620=FACE_OUTER_BOUND ( 'NONE', #30671, .T. ) ;
#30625=LINE ( 'NONE', #8140, #10971 ) ;
#30627=ORIENTED_EDGE ( 'NONE', *, *, #9160, .F. ) ;
#30632=ADVANCED_FACE ( 'NONE', ( #24926, #22771 ), #292, .F. ) ;
#30637=VERTEX_POINT ( 'NONE', #30179 ) ;
#30642=FACE_OUTER_BOUND ( 'NONE', #17523, .T. ) ;
#30648=CARTESIAN_POINT ( 'NONE',  ( -42.28301147118430237, 15.25948642862022986, 35.64930799450052490 ) ) ;
#30656=CARTESIAN_POINT ( 'NONE',  ( -40.70323106273447422, 6.774493230553032319, 34.57503839362117759 ) ) ;
#30661=FACE_BOUND ( 'NONE', #6069, .T. ) ;
#30665=CARTESIAN_POINT ( 'NONE',  ( -42.33363892739273382, 14.73725438281773847, 55.13459228725880479 ) ) ;
#30671=EDGE_LOOP ( 'NONE', ( #28522, #20370, #27322, #26965 ) ) ;
#30686=ORIENTED_EDGE ( 'NONE', *, *, #27282, .T. ) ;
#30693=DIRECTION ( 'NONE',  ( 0.2756373558170105986, -0.9612616959383156745, 0.000000000000000000 ) ) ;
#30701=EDGE_LOOP ( 'NONE', ( #16503, #25233, #24856 ) ) ;
#30703=CARTESIAN_POINT ( 'NONE',  ( -40.50726676868416121, 7.559560304694834088, 53.83429597860652649 ) ) ;
#30708=AXIS2_PLACEMENT_3D ( 'NONE', #20891, #30919, #11530 ) ;
#30709=EDGE_LOOP ( 'NONE', ( #4078, #14849, #21748 ) ) ;
#30713=CARTESIAN_POINT ( 'NONE',  ( -40.05987053574653345, 7.506472619680472746, 39.54930799450052348 ) ) ;
#30719=EDGE_CURVE ( 'NONE', #29624, #23397, #10960, .T. ) ;
#30724=CARTESIAN_POINT ( 'NONE',  ( -40.14651252454546437, 6.746025643617127088, 39.54930799450052348 ) ) ;
#30729=SURFACE_STYLE_USAGE ( .BOTH. , #20702 ) ;
#30737=EDGE_CURVE ( 'NONE', #30980, #5512, #31300, .T. ) ;
#30739=VERTEX_POINT ( 'NONE', #28667 ) ;
#30741=CARTESIAN_POINT ( 'NONE',  ( -40.13646513110854386, 7.213257191581853078, 38.95955396713193863 ) ) ;
#30749=DIRECTION ( 'NONE',  ( 0.8746197071393925215, -0.4848096202463429982, -8.676864087101708112E-18 ) ) ;
#30754=SPHERICAL_SURFACE ( 'NONE', #22962, 0.1000000000000000056 ) ;
#30757=AXIS2_PLACEMENT_3D ( 'NONE', #19520, #27408, #14936 ) ;
#30760=DIRECTION ( 'NONE',  ( -0.8746197071393810862, 0.4848096202463637039, 8.676864087101942305E-18 ) ) ;
#30765=CARTESIAN_POINT ( 'NONE',  ( -42.38263560350583248, 14.61917486843862868, 60.54930799450051637 ) ) ;
#30766=DIRECTION ( 'NONE',  ( 0.2756373558169947779, -0.9612616959383200044, 0.000000000000000000 ) ) ;
#30767=ADVANCED_FACE ( 'NONE', ( #18797, #30661 ), #16187, .T. ) ;
#30768=LINE ( 'NONE', #25355, #13162 ) ;
#30769=ORIENTED_EDGE ( 'NONE', *, *, #11600, .T. ) ;
#30770=FACE_OUTER_BOUND ( 'NONE', #15569, .T. ) ;
#30775=DIRECTION ( 'NONE',  ( 0.7848668881104262640, 0.2250569586005336520, 0.5773502691896258421 ) ) ;
#30780=DIRECTION ( 'NONE',  ( 0.000000000000000000, 0.000000000000000000, 1.000000000000000000 ) ) ;
#30788=ORIENTED_EDGE ( 'NONE', *, *, #32245, .F. ) ;
#30792=PLANE ( 'NONE',  #15438 ) ;
#30793=LINE ( 'NONE', #7994, #15846 ) ;
#30795=DIRECTION ( 'NONE',  ( 0.4848096202463673676, 0.8746197071393789768, 0.000000000000000000 ) ) ;
#30799=FACE_OUTER_BOUND ( 'NONE', #13250, .T. ) ;
#30803=ADVANCED_FACE ( 'NONE', ( #25887 ), #930, .T. ) ;
#30808=EDGE_CURVE ( 'NONE', #23798, #7845, #26686, .T. ) ;
#30814=ADVANCED_FACE ( 'NONE', ( #4039 ), #2063, .F. ) ;
#30823=CIRCLE ( 'NONE', #8772, 0.1000000000000008243 ) ;
#30828=VECTOR ( 'NONE', #7953, 1000.000000000000000 ) ;
#30834=CARTESIAN_POINT ( 'NONE',  ( -40.73091736380679606, 9.483895492497154578, 34.64930799450051779 ) ) ;
#30837=ORIENTED_EDGE ( 'NONE', *, *, #25760, .T. ) ;
#30839=ORIENTED_EDGE ( 'NONE', *, *, #18376, .F. ) ;
#30846=EDGE_CURVE ( 'NONE', #1803, #9995, #16916, .T. ) ;
#30850=EDGE_CURVE ( 'NONE', #12604, #23684, #14226, .T. ) ;
#30859=CARTESIAN_POINT ( 'NONE',  ( -40.70508238852949745, 9.491303552449114278, 35.44930799450052206 ) ) ;
#30865=VECTOR ( 'NONE', #27740, 1000.000000000000227 ) ;
#30866=ORIENTED_EDGE ( 'NONE', *, *, #4758, .T. ) ;
#30867=FACE_OUTER_BOUND ( 'NONE', #3830, .T. ) ;
#30872=VECTOR ( 'NONE', #26112, 1000.000000000000114 ) ;
#30873=ORIENTED_EDGE ( 'NONE', *, *, #2214, .F. ) ;
#30875=DIRECTION ( 'NONE',  ( -0.2756373558169974980, 0.9612616959383194493, 1.315048337272770743E-17 ) ) ;
#30878=CARTESIAN_POINT ( 'NONE',  ( -43.72819403793993587, 1.315833819094414769, 39.54930799450052348 ) ) ;
#30880=FACE_OUTER_BOUND ( 'NONE', #10628, .T. ) ;
#30883=DIRECTION ( 'NONE',  ( -0.4848096202463429427, -0.8746197071393925215, 4.053240046925389072E-19 ) ) ;
#30884=CARTESIAN_POINT ( 'NONE',  ( -40.64500813507293486, 6.819128862114091305, 34.57932936825760351 ) ) ;
#30888=VERTEX_POINT ( 'NONE', #31941 ) ;
#30889=CYLINDRICAL_SURFACE ( 'NONE', #28633, 0.1000000000000008243 ) ;
#30900=LINE ( 'NONE', #15629, #2819 ) ;
#30906=APPLICATION_CONTEXT ( 'automotive_design' ) ;
#30908=AXIS2_PLACEMENT_3D ( 'NONE', #24397, #31791, #1425 ) ;
#30916=AXIS2_PLACEMENT_3D ( 'NONE', #32063, #21374, #4323 ) ;
#30919=DIRECTION ( 'NONE',  ( 1.188208965918164993E-16, 1.880121038077812639E-16, 1.000000000000000000 ) ) ;
#30929=CARTESIAN_POINT ( 'NONE',  ( -40.10917099319649282, 6.845611892227013051, 34.60381041995846374 ) ) ;
#30937=CARTESIAN_POINT ( 'NONE',  ( -41.50386623137114839, 10.69791363055605515, 57.28220823191252720 ) ) ;
#30952=VECTOR ( 'NONE', #23014, 1000.000000000000000 ) ;
#30953=EDGE_CURVE ( 'NONE', #28083, #7551, #10648, .T. ) ;
#30954=CARTESIAN_POINT ( 'NONE',  ( -40.70335362822509495, 9.387769322903325886, 39.54930799450052348 ) ) ;
#30959=CARTESIAN_POINT ( 'NONE',  ( -40.76967387488526384, 8.530668925462080665, 39.44930799450052206 ) ) ;
#30970=ORIENTED_EDGE ( 'NONE', *, *, #10581, .T. ) ;
#30972=CARTESIAN_POINT ( 'NONE',  ( -41.77464577679393187, 3.808795504615559047, 32.14930799450051779 ) ) ;
#30977=VECTOR ( 'NONE', #10020, 1000.000000000000114 ) ;
#30978=DIRECTION ( 'NONE',  ( 0.4848096202463627602, 0.8746197071393815303, 0.000000000000000000 ) ) ;
#30979=CARTESIAN_POINT ( 'NONE',  ( -40.49379808738692788, 7.146223304870686022, 35.15525948572338422 ) ) ;
#30980=VERTEX_POINT ( 'NONE', #17489 ) ;
#30982=DIRECTION ( 'NONE',  ( -0.9612616959383183390, -0.2756373558170014948, -8.795445018805493151E-19 ) ) ;
#30983=CIRCLE ( 'NONE', #551, 0.1000000000000004774 ) ;
#30993=CIRCLE ( 'NONE', #16823, 0.09999999999999795164 ) ;
#30997=DIRECTION ( 'NONE',  ( -0.8746197071393810862, 0.4848096202463637039, 8.676864087101942305E-18 ) ) ;
#31001=ORIENTED_EDGE ( 'NONE', *, *, #21474, .F. ) ;
#31002=ORIENTED_EDGE ( 'NONE', *, *, #13645, .F. ) ;
#31004=AXIS2_PLACEMENT_3D ( 'NONE', #22213, #19425, #29453 ) ;
#31013=PLANE ( 'NONE',  #4006 ) ;
#31026=ADVANCED_FACE ( 'NONE', ( #17316 ), #12747, .T. ) ;
#31029=ORIENTED_EDGE ( 'NONE', *, *, #12386, .F. ) ;
#31031=CARTESIAN_POINT ( 'NONE',  ( -39.00632496464983490, 3.646315102566973998, 47.04930799450051637 ) ) ;
#31036=AXIS2_PLACEMENT_3D ( 'NONE', #17957, #25829, #15823 ) ;
#31042=PLANE ( 'NONE',  #899 ) ;
#31050=FACE_OUTER_BOUND ( 'NONE', #17651, .T. ) ;
#31058=ORIENTED_EDGE ( 'NONE', *, *, #23975, .F. ) ;
#31059=CARTESIAN_POINT ( 'NONE',  ( -43.29662792673756400, 1.063067023446606196, 53.64930799450051779 ) ) ;
#31069=ADVANCED_FACE ( 'NONE', ( #15035 ), #19777, .F. ) ;
#31074=DIRECTION ( 'NONE',  ( 7.588956326749211550E-18, -4.206627182996911684E-18, 1.000000000000000000 ) ) ;
#31075=VECTOR ( 'NONE', #2963, 1000.000000000000114 ) ;
#31089=FACE_OUTER_BOUND ( 'NONE', #27895, .T. ) ;
#31092=CARTESIAN_POINT ( 'NONE',  ( -42.38687957179149635, 4.148162238788000167, 39.04930799450052348 ) ) ;
#31093=VERTEX_POINT ( 'NONE', #20912 ) ;
#31094=DIRECTION ( 'NONE',  ( 1.188208965918165239E-16, 1.880121038077813132E-16, 1.000000000000000000 ) ) ;
#31095=CARTESIAN_POINT ( 'NONE',  ( -40.55202315603386864, 7.223587105649683870, 38.76578233797366835 ) ) ;
#31098=DIRECTION ( 'NONE',  ( 0.9612616959383221138, 0.2756373558169876170, 0.000000000000000000 ) ) ;
#31112=CIRCLE ( 'NONE', #31625, 0.09999999999999836797 ) ;
#31119=EDGE_LOOP ( 'NONE', ( #25253, #5875, #2587, #15708 ) ) ;
#31127=ORIENTED_EDGE ( 'NONE', *, *, #22067, .F. ) ;
#31128=DIRECTION ( 'NONE',  ( 0.4848096202463645921, 0.8746197071393805311, 0.000000000000000000 ) ) ;
#31133=CARTESIAN_POINT ( 'NONE',  ( -40.11286833322908052, 2.887657226147511302, 57.04930799450051637 ) ) ;
#31134=CARTESIAN_POINT ( 'NONE',  ( -40.65487266620045403, 9.475231293617264683, 39.43717596014455040 ) ) ;
#31140=CARTESIAN_POINT ( 'NONE',  ( -40.57495275781082711, 7.492308784443611813, 35.33000499469285671 ) ) ;
#31142=DIRECTION ( 'NONE',  ( 0.000000000000000000, 0.000000000000000000, 1.000000000000000000 ) ) ;
#31153=CARTESIAN_POINT ( 'NONE',  ( -43.64073206722599707, 1.267352857069779626, 34.64930799450052490 ) ) ;
#31154=VERTEX_POINT ( 'NONE', #28476 ) ;
#31163=PLANE ( 'NONE',  #7359 ) ;
#31164=DIRECTION ( 'NONE',  ( 0.2603858710390620779, -0.9080734476337356531, 0.3280271511107128446 ) ) ;
#31169=CIRCLE ( 'NONE', #13873, 0.09999999999999795164 ) ;
#31172=PLANE ( 'NONE',  #29695 ) ;
#31175=DIRECTION ( 'NONE',  ( 0.000000000000000000, 0.000000000000000000, 1.000000000000000000 ) ) ;
#31178=AXIS2_PLACEMENT_3D ( 'NONE', #19382, #24148, #9221 ) ;
#31184=ORIENTED_EDGE ( 'NONE', *, *, #28166, .F. ) ;
#31188=AXIS2_PLACEMENT_3D ( 'NONE', #21651, #6724, #16718 ) ;
#31206=CARTESIAN_POINT ( 'NONE',  ( -40.69616936570353971, 6.785751122969994498, 34.64127309652835152 ) ) ;
#31211=EDGE_CURVE ( 'NONE', #8513, #17105, #22040, .T. ) ;
#31216=EDGE_CURVE ( 'NONE', #29624, #2645, #16395, .T. ) ;
#31217=ORIENTED_EDGE ( 'NONE', *, *, #24865, .F. ) ;
#31231=LINE ( 'NONE', #862, #29255 ) ;
#31232=CARTESIAN_POINT ( 'NONE',  ( -43.73393778030726509, 1.305471833569777695, 60.54930799450051637 ) ) ;
#31236=CARTESIAN_POINT ( 'NONE',  ( -41.04804154345566758, 9.288931653684134204, 34.54930799450051637 ) ) ;
#31238=DIRECTION ( 'NONE',  ( 0.4832773644131139190, 0.8718554444429506001, -0.07944226231106060743 ) ) ;
#31242=CARTESIAN_POINT ( 'NONE',  ( -40.60330327974818232, 7.565477138576674143, 53.88146687024394055 ) ) ;
#31245=CARTESIAN_POINT ( 'NONE',  ( -40.57832940339291383, 7.446916344587776848, 60.29072935073781991 ) ) ;
#31250=CARTESIAN_POINT ( 'NONE',  ( -40.11096502192368263, 6.858424625636979854, 34.59247500421662380 ) ) ;
#31265=CIRCLE ( 'NONE', #6606, 1.624998423334082620 ) ;
#31274=EDGE_CURVE ( 'NONE', #2185, #26286, #21120, .T. ) ;
#31276=CARTESIAN_POINT ( 'NONE',  ( -40.61704948737776277, 6.826301864398534036, 34.55791711734467953 ) ) ;
#31277=ORIENTED_EDGE ( 'NONE', *, *, #17859, .T. ) ;
#31294=CARTESIAN_POINT ( 'NONE',  ( -40.70098307446937014, 6.778209214779045588, 34.68768967974548190 ) ) ;
#31300=LINE ( 'NONE', #3236, #25825 ) ;
#31303=ORIENTED_EDGE ( 'NONE', *, *, #22654, .T. ) ;
#31305=VECTOR ( 'NONE', #22433, 1000.000000000000114 ) ;
#31307=VERTEX_POINT ( 'NONE', #12541 ) ;
#31308=CARTESIAN_POINT ( 'NONE',  ( -39.59300248568538194, 7.744584186742828891, 61.94930799450052206 ) ) ;
#31311=CARTESIAN_POINT ( 'NONE',  ( -41.23380787120766655, 11.23768311167744294, 37.04930799450052348 ) ) ;
#31312=EDGE_CURVE ( 'NONE', #16068, #28989, #218, .T. ) ;
#31314=( BOUNDED_CURVE ( )  B_SPLINE_CURVE ( 3, ( #18201, #6226, #25765, #23625 ),
 .UNSPECIFIED., .F., .F. ) 
 B_SPLINE_CURVE_WITH_KNOTS ( ( 4, 4 ),
 ( 0.6077475352746632975, 1.139624073389847503 ),
 .UNSPECIFIED. ) 
 CURVE ( )  GEOMETRIC_REPRESENTATION_ITEM ( )  RATIONAL_B_SPLINE_CURVE ( ( 1.000000000000000000, 0.9765642231641280535, 0.9765642231641280535, 1.000000000000000000 ) ) 
 REPRESENTATION_ITEM ( '' )  );
#31315=CARTESIAN_POINT ( 'NONE',  ( -42.73182147790732444, -0.8057266458565844891, 61.94930799450052206 ) ) ;
#31320=CARTESIAN_POINT ( 'NONE',  ( -40.02540636251514172, 2.839176264122877047, 55.04930799450051637 ) ) ;
#31323=CARTESIAN_POINT ( 'NONE',  ( -40.68283709840997631, 6.807248601136921984, 39.30095348056342885 ) ) ;
#31324=CARTESIAN_POINT ( 'NONE',  ( -40.52510752649232728, 7.677764709599122384, 34.54930799450052348 ) ) ;
#31328=ORIENTED_EDGE ( 'NONE', *, *, #4706, .T. ) ;
#31329=DIRECTION ( 'NONE',  ( -2.779292025043186357E-18, 1.288349127009862211E-17, -1.000000000000000000 ) ) ;
#31335=CARTESIAN_POINT ( 'NONE',  ( -40.99628586177130529, 8.927770518203464789, 56.04611646155296256 ) ) ;
#31349=CYLINDRICAL_SURFACE ( 'NONE', #17058, 0.09999999999999945044 ) ;
#31353=EDGE_LOOP ( 'NONE', ( #16368, #16392, #16409, #13128 ) ) ;
#31358=CARTESIAN_POINT ( 'NONE',  ( -40.11729073372970333, 6.802967823440400963, 39.44930799450052206 ) ) ;
#31359=EDGE_LOOP ( 'NONE', ( #17535, #3348, #31669, #19984, #16875 ) ) ;
#31360=CARTESIAN_POINT ( 'NONE',  ( -41.41619974353107381, 10.78537257809431615, 36.23067884439899444 ) ) ;
#31365=DIRECTION ( 'NONE',  ( 0.2756373558170082672, -0.9612616959383162296, -6.938893903907184201E-14 ) ) ;
#31367=ORIENTED_EDGE ( 'NONE', *, *, #931, .F. ) ;
#31375=CARTESIAN_POINT ( 'NONE',  ( -40.51045226066063520, 7.589116544599141534, 60.22001867261916885 ) ) ;
#31378=CONICAL_SURFACE ( 'NONE', #29282, 1.003191532947550701, 0.7853981633974447263 ) ;
#31380=CARTESIAN_POINT ( 'NONE',  ( -40.99469220063296859, 10.73619040060270002, 57.17865484131924347 ) ) ;
#31392=EDGE_CURVE ( 'NONE', #21311, #26286, #4380, .T. ) ;
#31393=DIRECTION ( 'NONE',  ( -0.8746197071393877476, 0.4848096202463514359, 0.000000000000000000 ) ) ;
#31395=EDGE_CURVE ( 'NONE', #2133, #3392, #7453, .T. ) ;
#31396=CARTESIAN_POINT ( 'NONE',  ( -42.48178708409979265, 14.60617548783703690, 60.54930799450051637 ) ) ;
#31404=ORIENTED_EDGE ( 'NONE', *, *, #18843, .F. ) ;
#31405=DIRECTION ( 'NONE',  ( 0.2756373558169958327, -0.9612616959383198934, 0.000000000000000000 ) ) ;
#31409=AXIS2_PLACEMENT_3D ( 'NONE', #16386, #21461, #15910 ) ;
#31412=CYLINDRICAL_SURFACE ( 'NONE', #15577, 0.1000000000000007272 ) ;
#31417=CARTESIAN_POINT ( 'NONE',  ( -40.02540636251513462, 2.839176264122873050, 35.84930799450052064 ) ) ;
#31424=EDGE_CURVE ( 'NONE', #23543, #22288, #17280, .T. ) ;
#31436=DIRECTION ( 'NONE',  ( 0.000000000000000000, 1.517883041479704827E-15, -1.000000000000000000 ) ) ;
#31447=DIRECTION ( 'NONE',  ( 0.4848096202463405002, 0.8746197071393938538, 0.000000000000000000 ) ) ;
#31448=AXIS2_PLACEMENT_3D ( 'NONE', #9439, #4672, #9925 ) ;
#31449=ORIENTED_EDGE ( 'NONE', *, *, #26386, .F. ) ;
#31456=CARTESIAN_POINT ( 'NONE',  ( -40.07989290236490376, 6.890692649785586710, 34.91305977274481620 ) ) ;
#31461=CARTESIAN_POINT ( 'NONE',  ( -41.94956971822180947, 3.905757428664829334, 45.14930799450051779 ) ) ;
#31462=ORIENTED_EDGE ( 'NONE', *, *, #1926, .T. ) ;
#31463=ORIENTED_EDGE ( 'NONE', *, *, #9160, .T. ) ;
#31467=ORIENTED_EDGE ( 'NONE', *, *, #18523, .F. ) ;
#31470=EDGE_CURVE ( 'NONE', #18870, #23253, #30900, .T. ) ;
#31478=AXIS2_PLACEMENT_3D ( 'NONE', #20675, #15274, #656 ) ;
#31479=ORIENTED_EDGE ( 'NONE', *, *, #1777, .T. ) ;
#31483=ORIENTED_EDGE ( 'NONE', *, *, #4706, .F. ) ;
#31484=DIRECTION ( 'NONE',  ( 2.779292025043186357E-18, -1.288349127009862211E-17, 1.000000000000000000 ) ) ;
#31486=CARTESIAN_POINT ( 'NONE',  ( -40.56019413908494187, 7.186695055020557277, 38.80167063144872230 ) ) ;
#31490=CARTESIAN_POINT ( 'NONE',  ( -41.40774006177731081, 10.72547736613775626, 57.28220823191252720 ) ) ;
#31491=CARTESIAN_POINT ( 'NONE',  ( -40.46271621608484281, 3.081581074246048768, 38.54930799450052348 ) ) ;
#31497=CARTESIAN_POINT ( 'NONE',  ( -39.59792565122570096, 7.943629834091020747, 34.54930799450052348 ) ) ;
#31499=DIRECTION ( 'NONE',  ( -7.588956326749211550E-18, 4.206627182996911684E-18, -1.000000000000000000 ) ) ;
#31501=ORIENTED_EDGE ( 'NONE', *, *, #842, .T. ) ;
#31502=DIRECTION ( 'NONE',  ( -0.8746197071393926326, 0.4848096202463430537, 8.676864087101709653E-18 ) ) ;
#31510=ORIENTED_EDGE ( 'NONE', *, *, #23456, .F. ) ;
#31511=AXIS2_PLACEMENT_3D ( 'NONE', #2332, #29582, #14158 ) ;
#31518=LINE ( 'NONE', #13793, #18849 ) ;
#31519=AXIS2_PLACEMENT_3D ( 'NONE', #32460, #19972, #2033 ) ;
#31531=EDGE_CURVE ( 'NONE', #30980, #23798, #26040, .T. ) ;
#31532=CIRCLE ( 'NONE', #27851, 0.1000000000000028644 ) ;
#31534=ORIENTED_EDGE ( 'NONE', *, *, #16072, .F. ) ;
#31535=ORIENTED_EDGE ( 'NONE', *, *, #933, .T. ) ;
#31537=DIRECTION ( 'NONE',  ( 0.8746197071393926326, -0.4848096202463430537, -8.676864087101709653E-18 ) ) ;
#31542=ORIENTED_EDGE ( 'NONE', *, *, #1932, .T. ) ;
#31553=FACE_OUTER_BOUND ( 'NONE', #5679, .T. ) ;
#31556=ORIENTED_EDGE ( 'NONE', *, *, #16887, .F. ) ;
#31559=CIRCLE ( 'NONE', #16347, 1.899999999999999023 ) ;
#31564=LINE ( 'NONE', #9070, #8417 ) ;
#31579=DIRECTION ( 'NONE',  ( -0.4848096202463774151, -0.8746197071393733147, 0.000000000000000000 ) ) ;
#31581=DIRECTION ( 'NONE',  ( -0.2756373558169932236, 0.9612616959383205595, -1.479773560108267395E-16 ) ) ;
#31583=FACE_OUTER_BOUND ( 'NONE', #16554, .T. ) ;
#31584=EDGE_CURVE ( 'NONE', #18455, #19824, #6748, .T. ) ;
#31585=DIRECTION ( 'NONE',  ( 0.9612616959383313286, 0.2756373558169555871, 0.000000000000000000 ) ) ;
#31591=VECTOR ( 'NONE', #24289, 1000.000000000000000 ) ;
#31592=CIRCLE ( 'NONE', #9047, 0.09999999999999845124 ) ;
#31593=VECTOR ( 'NONE', #19637, 1000.000000000000114 ) ;
#31594=AXIS2_PLACEMENT_3D ( 'NONE', #4527, #21591, #9458 ) ;
#31598=EDGE_LOOP ( 'NONE', ( #6007, #24903, #30600, #4026 ) ) ;
#31602=CARTESIAN_POINT ( 'NONE',  ( -41.63422246745999189, 11.51531537899137447, 57.04930799450051637 ) ) ;
#31604=FACE_OUTER_BOUND ( 'NONE', #9945, .T. ) ;
#31607=ORIENTED_EDGE ( 'NONE', *, *, #9759, .F. ) ;
#31610=DIRECTION ( 'NONE',  ( 0.000000000000000000, 0.000000000000000000, 1.000000000000000000 ) ) ;
#31619=CARTESIAN_POINT ( 'NONE',  ( -42.38474149870877028, 15.25146566812707505, 38.54930799450052348 ) ) ;
#31623=EDGE_CURVE ( 'NONE', #17347, #2789, #31860, .T. ) ;
#31625=AXIS2_PLACEMENT_3D ( 'NONE', #21456, #18828, #13609 ) ;
#31627=EDGE_CURVE ( 'NONE', #4349, #5375, #11355, .T. ) ;
#31634=ORIENTED_EDGE ( 'NONE', *, *, #28648, .T. ) ;
#31635=DIRECTION ( 'NONE',  ( -0.9612616959383200044, -0.2756373558169954996, 1.660411357259285896E-16 ) ) ;
#31646=EDGE_LOOP ( 'NONE', ( #495, #16936, #24929, #12371 ) ) ;
#31647=CARTESIAN_POINT ( 'NONE',  ( -40.48129536610376533, 8.613360132207176889, 39.44930799450052206 ) ) ;
#31652=CARTESIAN_POINT ( 'NONE',  ( -40.61337426079425228, 6.957937756952573771, 39.01901553589728167 ) ) ;
#31654=CARTESIAN_POINT ( 'NONE',  ( -40.52669582637187773, 7.652910973922034010, 60.15421819779514578 ) ) ;
#31658=ORIENTED_EDGE ( 'NONE', *, *, #29081, .T. ) ;
#31659=DIRECTION ( 'NONE',  ( -0.3958453973320084640, -0.7141240004913232964, 0.5773502691896251759 ) ) ;
#31664=ORIENTED_EDGE ( 'NONE', *, *, #8023, .F. ) ;
#31669=ORIENTED_EDGE ( 'NONE', *, *, #10821, .F. ) ;
#31670=ORIENTED_EDGE ( 'NONE', *, *, #8586, .F. ) ;
#31672=FACE_BOUND ( 'NONE', #2847, .T. ) ;
#31673=DIRECTION ( 'NONE',  ( -0.3958453973319808195, -0.7141240004913296247, -0.5773502691896363892 ) ) ;
#31678=CARTESIAN_POINT ( 'NONE',  ( -40.05987053574653345, 7.506472619680471858, 34.64930799450051779 ) ) ;
#31691=ORIENTED_EDGE ( 'NONE', *, *, #10669, .T. ) ;
#31694=DIRECTION ( 'NONE',  ( 2.779292025043186357E-18, -1.288349127009862211E-17, 1.000000000000000000 ) ) ;
#31695=DIRECTION ( 'NONE',  ( 0.8746197071393926326, -0.4848096202463430537, -8.676864087101709653E-18 ) ) ;
#31696=ORIENTED_EDGE ( 'NONE', *, *, #13621, .F. ) ;
#31702=EDGE_CURVE ( 'NONE', #15339, #18438, #28039, .T. ) ;
#31704=AXIS2_PLACEMENT_3D ( 'NONE', #17744, #4628, #4796 ) ;
#31709=PLANE ( 'NONE',  #1289 ) ;
#31711=LINE ( 'NONE', #4616, #2865 ) ;
#31714=ORIENTED_EDGE ( 'NONE', *, *, #19565, .T. ) ;
#31716=DIRECTION ( 'NONE',  ( 1.188208965918165239E-16, 1.880121038077813132E-16, 1.000000000000000000 ) ) ;
#31717=DIRECTION ( 'NONE',  ( 0.2756373558169931126, -0.9612616959383206705, 1.479773560108267642E-16 ) ) ;
#31718=ADVANCED_FACE ( 'NONE', ( #12169 ), #2477, .T. ) ;
#31723=CYLINDRICAL_SURFACE ( 'NONE', #20987, 1.199999999999999734 ) ;
#31724=AXIS2_PLACEMENT_3D ( 'NONE', #14770, #29703, #19513 ) ;
#31727=VERTEX_POINT ( 'NONE', #9866 ) ;
#31738=CARTESIAN_POINT ( 'NONE',  ( -40.11286833322908052, 2.887657226147509970, 55.84930799450052064 ) ) ;
#31739=VERTEX_POINT ( 'NONE', #21996 ) ;
#31746=CARTESIAN_POINT ( 'NONE',  ( -40.59290689585611744, 7.518854022824533523, 60.12740069859619751 ) ) ;
#31750=CARTESIAN_POINT ( 'NONE',  ( -42.37913764077812573, 15.23192269303852875, 38.44930799450052206 ) ) ;
#31758=ORIENTED_EDGE ( 'NONE', *, *, #22831, .F. ) ;
#31762=DIRECTION ( 'NONE',  ( 0.8746197071393926326, -0.4848096202463430537, -8.676864087101709653E-18 ) ) ;
#31767=DIRECTION ( 'NONE',  ( -0.2756373558170034377, 0.9612616959383176729, -3.701728707981190596E-16 ) ) ;
#31770=CARTESIAN_POINT ( 'NONE',  ( -40.12057988072736947, 7.355395738388389226, 35.24232147887364874 ) ) ;
#31774=ORIENTED_EDGE ( 'NONE', *, *, #18415, .T. ) ;
#31789=DIRECTION ( 'NONE',  ( -0.8746197071393926326, 0.4848096202463430537, 8.676864087101709653E-18 ) ) ;
#31791=DIRECTION ( 'NONE',  ( -0.8746197071393790878, 0.4848096202463673676, 1.277302113040196197E-17 ) ) ;
#31792=ADVANCED_FACE ( 'NONE', ( #12004 ), #22485, .F. ) ;
#31795=EDGE_CURVE ( 'NONE', #5664, #21721, #27094, .T. ) ;
#31806=CARTESIAN_POINT ( 'NONE',  ( -40.68765130478452363, 6.801118111650202636, 39.35160066530853840 ) ) ;
#31809=CARTESIAN_POINT ( 'NONE',  ( -43.42682711710880739, 1.034448000281938285, 39.54930799450052348 ) ) ;
#31813=PLANE ( 'NONE',  #18216 ) ;
#31814=DIRECTION ( 'NONE',  ( 0.2756373558169947779, -0.9612616959383200044, 0.000000000000000000 ) ) ;
#31817=ORIENTED_EDGE ( 'NONE', *, *, #3033, .F. ) ;
#31818=ORIENTED_EDGE ( 'NONE', *, *, #550, .F. ) ;
#31819=CARTESIAN_POINT ( 'NONE',  ( -42.47434154250543514, 4.196643200812633978, 38.94930799450052206 ) ) ;
#31823=ADVANCED_FACE ( 'NONE', ( #7729 ), #29731, .F. ) ;
#31825=DIRECTION ( 'NONE',  ( 2.779292025043186357E-18, -1.288349127009862211E-17, 1.000000000000000000 ) ) ;
#31831=DIRECTION ( 'NONE',  ( 0.9612616959383200044, 0.2756373558169954996, -1.660411357259285896E-16 ) ) ;
#31834=SPHERICAL_SURFACE ( 'NONE', #6538, 0.1000000000000000056 ) ;
#31848=VERTEX_POINT ( 'NONE', #13145 ) ;
#31851=FACE_OUTER_BOUND ( 'NONE', #2901, .T. ) ;
#31853=DIRECTION ( 'NONE',  ( -0.6797146636928645957, -0.1949050434465350867, 0.7071067811865476838 ) ) ;
#31854=ORIENTED_EDGE ( 'NONE', *, *, #27838, .F. ) ;
#31860=LINE ( 'NONE', #29405, #10694 ) ;
#31861=EDGE_CURVE ( 'NONE', #23543, #18622, #15280, .T. ) ;
#31863=ADVANCED_FACE ( 'NONE', ( #18051 ), #261, .T. ) ;
#31864=AXIS2_PLACEMENT_3D ( 'NONE', #31308, #8812, #6356 ) ;
#31865=EDGE_LOOP ( 'NONE', ( #26776, #16416, #22821, #9105, #29376 ) ) ;
#31871=VECTOR ( 'NONE', #4464, 1000.000000000000227 ) ;
#31874=DIRECTION ( 'NONE',  ( 1.188208965918165239E-16, 1.880121038077813132E-16, 1.000000000000000000 ) ) ;
#31876=DIRECTION ( 'NONE',  ( -0.8746197071393926326, 0.4848096202463430537, 8.676864087101709653E-18 ) ) ;
#31878=DIRECTION ( 'NONE',  ( 0.000000000000000000, 0.000000000000000000, -1.000000000000000000 ) ) ;
#31898=CARTESIAN_POINT ( 'NONE',  ( -40.11553135844171436, 6.871094863070439374, 39.51608551794754476 ) ) ;
#31902=TOROIDAL_SURFACE ( 'NONE', #11464, 0.8999999999999995781, 0.1000000000000000056 ) ;
#31903=CARTESIAN_POINT ( 'NONE',  ( -36.76418579970419387, 10.14130568307076352, 57.95249952744806166 ) ) ;
#31906=EDGE_LOOP ( 'NONE', ( #5202, #6647, #29762 ) ) ;
#31911=FACE_OUTER_BOUND ( 'NONE', #28548, .T. ) ;
#31914=ORIENTED_EDGE ( 'NONE', *, *, #9719, .F. ) ;
#31923=DIRECTION ( 'NONE',  ( -0.4848096202463430537, -0.8746197071393926326, -9.920727850371700117E-18 ) ) ;
#31926=LINE ( 'NONE', #17134, #8675 ) ;
#31941=CARTESIAN_POINT ( 'NONE',  ( -42.68334051588269062, -0.7182646751426463583, 32.04930799450052348 ) ) ;
#31945=VECTOR ( 'NONE', #16224, 1000.000000000000000 ) ;
#31946=ORIENTED_EDGE ( 'NONE', *, *, #4991, .F. ) ;
#31949=CARTESIAN_POINT ( 'NONE',  ( -41.93344242462055149, 13.82826554927148166, 54.56265170360538264 ) ) ;
#31952=ORIENTED_EDGE ( 'NONE', *, *, #26307, .T. ) ;
#31954=CARTESIAN_POINT ( 'NONE',  ( -40.11286833322907341, 2.887657226147507306, 37.04930799450052348 ) ) ;
#31955=DIRECTION ( 'NONE',  ( 0.4848096202463673121, 0.8746197071393789768, 0.000000000000000000 ) ) ;
#31965=CIRCLE ( 'NONE', #25153, 0.1000000000000016709 ) ;
#31966=VECTOR ( 'NONE', #28475, 1000.000000000000227 ) ;
#31968=DIRECTION ( 'NONE',  ( 0.7141240004913684825, -0.3958453973319465691, 0.5773502691896116312 ) ) ;
#31975=CARTESIAN_POINT ( 'NONE',  ( -41.02113223168485234, 7.230835263863472306, 39.44930799450052206 ) ) ;
#31976=CIRCLE ( 'NONE', #2069, 0.09999999999999792388 ) ;
#31981=ORIENTED_EDGE ( 'NONE', *, *, #3204, .F. ) ;
#31984=AXIS2_PLACEMENT_3D ( 'NONE', #1843, #19224, #6611 ) ;
#31987=EDGE_CURVE ( 'NONE', #13785, #8280, #28016, .T. ) ;
#31995=CARTESIAN_POINT ( 'NONE',  ( -40.11286833322907341, 2.887657226147507306, 35.74930799450051921 ) ) ;
#32001=VERTEX_POINT ( 'NONE', #30648 ) ;
#32002=ORIENTED_EDGE ( 'NONE', *, *, #32216, .F. ) ;
#32004=VECTOR ( 'NONE', #2257, 1000.000000000000000 ) ;
#32009=DIRECTION ( 'NONE',  ( -0.2756373558170082672, 0.9612616959383162296, 0.000000000000000000 ) ) ;
#32013=CARTESIAN_POINT ( 'NONE',  ( -40.70484894842233103, 8.274204744976163539, 59.44930799450051495 ) ) ;
#32014=CARTESIAN_POINT ( 'NONE',  ( -40.05987053574653345, 7.506472619680471858, 35.64930799450052490 ) ) ;
#32016=DIRECTION ( 'NONE',  ( -2.779292025043186357E-18, 1.288349127009862211E-17, -1.000000000000000000 ) ) ;
#32024=CARTESIAN_POINT ( 'NONE',  ( -40.60722745863126448, 9.415333058485025219, 39.40788663826321425 ) ) ;
#32026=DIRECTION ( 'NONE',  ( -0.8746197071393858602, 0.4848096202463547666, 0.000000000000000000 ) ) ;
#32027=ADVANCED_FACE ( 'NONE', ( #8637 ), #8159, .T. ) ;
#32030=EDGE_CURVE ( 'NONE', #4736, #5569, #12311, .T. ) ;
#32033=DIRECTION ( 'NONE',  ( 0.3428121700606640565, 0.6184495258776567805, -0.7071067811865473507 ) ) ;
#32034=CYLINDRICAL_SURFACE ( 'NONE', #31178, 0.1000000000000010325 ) ;
#32045=DIRECTION ( 'NONE',  ( -0.8746197071393858602, 0.4848096202463547666, 0.000000000000000000 ) ) ;
#32048=LINE ( 'NONE', #22679, #21487 ) ;
#32050=CARTESIAN_POINT ( 'NONE',  ( -40.61650700234910971, 6.826799243660863326, 39.53667871757248520 ) ) ;
#32052=ORIENTED_EDGE ( 'NONE', *, *, #9225, .F. ) ;
#32057=LINE ( 'NONE', #19229, #27705 ) ;
#32060=ORIENTED_EDGE ( 'NONE', *, *, #1703, .T. ) ;
#32063=CARTESIAN_POINT ( 'NONE',  ( -40.18454328187963398, 7.548069831825862330, 60.29072935073781991 ) ) ;
#32064=ORIENTED_EDGE ( 'NONE', *, *, #17891, .T. ) ;
#32065=ORIENTED_EDGE ( 'NONE', *, *, #13867, .F. ) ;
#32066=DIRECTION ( 'NONE',  ( 0.8746197071393926326, -0.4848096202463430537, -8.676864087101709653E-18 ) ) ;
#32071=ORIENTED_EDGE ( 'NONE', *, *, #16476, .T. ) ;
#32074=VERTEX_POINT ( 'NONE', #23082 ) ;
#32076=ADVANCED_FACE ( 'NONE', ( #30799 ), #21188, .T. ) ;
#32078=AXIS2_PLACEMENT_3D ( 'NONE', #19803, #7515, #32299 ) ;
#32079=EDGE_LOOP ( 'NONE', ( #11687, #20733, #9012, #24591, #28661, #12537, #25074, #10522 ) ) ;
#32081=DIRECTION ( 'NONE',  ( -7.588956326749211550E-18, 4.206627182996912454E-18, -1.000000000000000000 ) ) ;
#32084=ORIENTED_EDGE ( 'NONE', *, *, #3337, .F. ) ;
#32086=ORIENTED_EDGE ( 'NONE', *, *, #123, .T. ) ;
#32088=AXIS2_PLACEMENT_3D ( 'NONE', #17962, #20906, #7971 ) ;
#32089=( BOUNDED_CURVE ( )  B_SPLINE_CURVE ( 3, ( #7910, #22829, #28092, #3121 ),
 .UNSPECIFIED., .F., .F. ) 
 B_SPLINE_CURVE_WITH_KNOTS ( ( 4, 4 ),
 ( 5.497787143782102426, 6.283185307179586232 ),
 .UNSPECIFIED. ) 
 CURVE ( )  GEOMETRIC_REPRESENTATION_ITEM ( )  RATIONAL_B_SPLINE_CURVE ( ( 1.000000000000000000, 0.9492530216741865701, 0.9492530216741865701, 1.000000000000000000 ) ) 
 REPRESENTATION_ITEM ( '' )  );
#32090=DIRECTION ( 'NONE',  ( -0.2756373558169945559, 0.9612616959383202264, 0.000000000000000000 ) ) ;
#32094=CARTESIAN_POINT ( 'NONE',  ( -40.28779227465695811, 2.984619150196779813, 57.04930799450051637 ) ) ;
#32099=CARTESIAN_POINT ( 'NONE',  ( -40.57832940339291383, 7.446916344587776848, 53.80788663826320573 ) ) ;
#32105=FACE_OUTER_BOUND ( 'NONE', #11174, .T. ) ;
#32106=VERTEX_POINT ( 'NONE', #23562 ) ;
#32112=ORIENTED_EDGE ( 'NONE', *, *, #22217, .T. ) ;
#32116=CIRCLE ( 'NONE', #27383, 0.9031915329475502796 ) ;
#32125=DIRECTION ( 'NONE',  ( -0.8746197071393840838, 0.4848096202463581528, 0.000000000000000000 ) ) ;
#32132=CARTESIAN_POINT ( 'NONE',  ( -40.47970302497626705, 7.463434137431151250, 53.64930799450051779 ) ) ;
#32133=EDGE_CURVE ( 'NONE', #12291, #13584, #2378, .T. ) ;
#32136=CARTESIAN_POINT ( 'NONE',  ( -37.58300281841709989, 16.01180101885526597, 36.00717268343339583 ) ) ;
#32138=CARTESIAN_POINT ( 'NONE',  ( -40.18454328187963398, 7.548069831825862330, 60.29072935073781991 ) ) ;
#32141=VECTOR ( 'NONE', #6990, 1000.000000000000227 ) ;
#32142=VECTOR ( 'NONE', #17182, 1000.000000000000000 ) ;
#32144=CARTESIAN_POINT ( 'NONE',  ( -41.94956971822180947, 3.905757428664830222, 48.24930799450051211 ) ) ;
#32148=FACE_OUTER_BOUND ( 'NONE', #14477, .T. ) ;
#32150=DIRECTION ( 'NONE',  ( 0.9612616959383188942, 0.2756373558169995519, -1.660411357259292306E-16 ) ) ;
#32151=ORIENTED_EDGE ( 'NONE', *, *, #11756, .T. ) ;
#32152=EDGE_LOOP ( 'NONE', ( #31714, #28006, #6991, #153 ) ) ;
#32153=CARTESIAN_POINT ( 'NONE',  ( -42.37913764077812573, 15.23192269303852875, 35.64930799450052490 ) ) ;
#32159=VECTOR ( 'NONE', #22276, 1000.000000000000000 ) ;
#32161=DIRECTION ( 'NONE',  ( 0.3428121700606640565, 0.6184495258776567805, -0.7071067811865474617 ) ) ;
#32163=ORIENTED_EDGE ( 'NONE', *, *, #14763, .T. ) ;
#32164=CARTESIAN_POINT ( 'NONE',  ( -41.34584395867850048, 11.59800658573647247, 57.04930799450051637 ) ) ;
#32169=ORIENTED_EDGE ( 'NONE', *, *, #22096, .T. ) ;
#32172=ORIENTED_EDGE ( 'NONE', *, *, #7846, .F. ) ;
#32175=CARTESIAN_POINT ( 'NONE',  ( -40.68496126738437368, 6.805971067583526768, 34.76999393395801974 ) ) ;
#32179=CARTESIAN_POINT ( 'NONE',  ( -36.38930206846553261, 9.511667899829566508, 54.44930799450051495 ) ) ;
#32184=DIRECTION ( 'NONE',  ( -0.9612616959383206705, -0.2756373558169934457, 1.660411357259282938E-16 ) ) ;
#32185=CARTESIAN_POINT ( 'NONE',  ( -40.18454328187963398, 7.548069831825862330, 60.54930799450051637 ) ) ;
#32188=ORIENTED_EDGE ( 'NONE', *, *, #8767, .F. ) ;
#32194=DIRECTION ( 'NONE',  ( 0.1949050434465247061, -0.6797146636928672603, 0.7071067811865480168 ) ) ;
#32196=AXIS2_PLACEMENT_3D ( 'NONE', #26618, #14156, #24156 ) ;
#32199=LINE ( 'NONE', #9715, #15039 ) ;
#32201=CARTESIAN_POINT ( 'NONE',  ( -40.70484894842233103, 8.274204744976163539, 54.54930799450051637 ) ) ;
#32205=CARTESIAN_POINT ( 'NONE',  ( -43.69495677161796010, 1.169528900831203311, 53.64930799450051779 ) ) ;
#32210=DIRECTION ( 'NONE',  ( -0.8746197071393890798, 0.4848096202463489934, 8.676864087101777446E-18 ) ) ;
#32216=EDGE_CURVE ( 'NONE', #23287, #13496, #24924, .T. ) ;
#32223=CARTESIAN_POINT ( 'NONE',  ( -40.38645765092156381, 8.586711236632284638, 34.59301614167199546 ) ) ;
#32225=DIRECTION ( 'NONE',  ( -2.779292025043186357E-18, 1.288349127009862211E-17, -1.000000000000000000 ) ) ;
#32231=ORIENTED_EDGE ( 'NONE', *, *, #26111, .T. ) ;
#32232=VERTEX_POINT ( 'NONE', #12360 ) ;
#32241=CARTESIAN_POINT ( 'NONE',  ( -40.08841711228579641, 7.575633567407562552, 60.44930799450051495 ) ) ;
#32245=EDGE_CURVE ( 'NONE', #18805, #1639, #9885, .T. ) ;
#32252=ORIENTED_EDGE ( 'NONE', *, *, #9040, .F. ) ;
#32259=ADVANCED_FACE ( 'NONE', ( #24208 ), #14528, .F. ) ;
#32262=DIRECTION ( 'NONE',  ( 0.000000000000000000, 0.000000000000000000, -1.000000000000000000 ) ) ;
#32267=ORIENTED_EDGE ( 'NONE', *, *, #1929, .T. ) ;
#32283=DIRECTION ( 'NONE',  ( 1.188208965918165239E-16, 1.880121038077813132E-16, 1.000000000000000000 ) ) ;
#32289=CARTESIAN_POINT ( 'NONE',  ( -36.37788479535792163, 9.471851136684824368, 54.54930799450051637 ) ) ;
#32294=ORIENTED_EDGE ( 'NONE', *, *, #23110, .F. ) ;
#32298=EDGE_LOOP ( 'NONE', ( #12754, #24431, #2723, #885 ) ) ;
#32299=DIRECTION ( 'NONE',  ( 0.2756373558170082672, -0.9612616959383162296, 0.000000000000000000 ) ) ;
#32300=LINE ( 'NONE', #30002, #32004 ) ;
#32306=DIRECTION ( 'NONE',  ( 0.000000000000000000, 0.000000000000000000, -1.000000000000000000 ) ) ;
#32313=CARTESIAN_POINT ( 'NONE',  ( -42.38687957179150345, 4.148162238788004608, 58.24930799450051921 ) ) ;
#32314=VERTEX_POINT ( 'NONE', #1722 ) ;
#32315=EDGE_CURVE ( 'NONE', #2732, #29138, #4674, .T. ) ;
#32330=DIRECTION ( 'NONE',  ( 0.4848096202463461624, 0.8746197071393907452, 9.920727850371670843E-18 ) ) ;
#32334=ORIENTED_EDGE ( 'NONE', *, *, #28799, .F. ) ;
#32346=CIRCLE ( 'NONE', #4024, 0.1000000000000018235 ) ;
#32348=DIRECTION ( 'NONE',  ( 0.8746197071393926326, -0.4848096202463430537, -8.676864087101709653E-18 ) ) ;
#32358=VERTEX_POINT ( 'NONE', #4352 ) ;
#32359=EDGE_CURVE ( 'NONE', #2697, #27609, #6917, .T. ) ;
#32360=ORIENTED_EDGE ( 'NONE', *, *, #13867, .T. ) ;
#32368=FACE_OUTER_BOUND ( 'NONE', #26350, .T. ) ;
#32371=CARTESIAN_POINT ( 'NONE',  ( -40.51565501380215295, 9.065589196111961456, 57.04930799450051637 ) ) ;
#32372=DIRECTION ( 'NONE',  ( -0.1540342867254180514, 0.6907746437949934259, 0.7064728091037132396 ) ) ;
#32387=ORIENTED_EDGE ( 'NONE', *, *, #26569, .F. ) ;
#32389=LINE ( 'NONE', #9904, #23603 ) ;
#32396=CIRCLE ( 'NONE', #2517, 1.300000000000002487 ) ;
#32400=ORIENTED_EDGE ( 'NONE', *, *, #26202, .T. ) ;
#32404=CARTESIAN_POINT ( 'NONE',  ( -40.51045226066063520, 7.589116544599140646, 53.87859731638185679 ) ) ;
#32407=CARTESIAN_POINT ( 'NONE',  ( -40.14060284811700541, 7.788019651925919717, 34.54930799450052348 ) ) ;
#32411=ORIENTED_EDGE ( 'NONE', *, *, #1968, .T. ) ;
#32418=CARTESIAN_POINT ( 'NONE',  ( -40.09211399732166115, 9.667069410243957606, 34.64930799450051779 ) ) ;
#32424=AXIS2_PLACEMENT_3D ( 'NONE', #12183, #15291, #24815 ) ;
#32427=DIRECTION ( 'NONE',  ( -0.9612616959383200044, -0.2756373558169954996, 1.660411357259285896E-16 ) ) ;
#32430=EDGE_CURVE ( 'NONE', #22442, #8660, #10418, .T. ) ;
#32439=CIRCLE ( 'NONE', #16155, 0.09999999999999795164 ) ;
#32440=ADVANCED_FACE ( 'NONE', ( #8116 ), #25427, .T. ) ;
#32444=EDGE_CURVE ( 'NONE', #22288, #7112, #1872, .T. ) ;
#32448=ORIENTED_EDGE ( 'NONE', *, *, #6836, .T. ) ;
#32449=DIRECTION ( 'NONE',  ( 0.6184495258776571136, -0.3428121700606572286, 0.7071067811865504593 ) ) ;
#32452=FACE_OUTER_BOUND ( 'NONE', #22363, .T. ) ;
#32460=CARTESIAN_POINT ( 'NONE',  ( -41.52218637998915085, 11.15499190493234671, 37.04930799450052348 ) ) ;
#32461=VECTOR ( 'NONE', #5027, 1000.000000000000114 ) ;
#32466=DIRECTION ( 'NONE',  ( -0.8746197071393926326, 0.4848096202463430537, 8.676864087101709653E-18 ) ) ;
#32470=CARTESIAN_POINT ( 'NONE',  ( -40.28136326135769707, 8.248516754564388265, 54.59072935073782418 ) ) ;
#32475=DIRECTION ( 'NONE',  ( 0.8746197071393926326, -0.4848096202463430537, -8.676864087101709653E-18 ) ) ;
#32479=ORIENTED_EDGE ( 'NONE', *, *, #4567, .F. ) ;
#32487=ORIENTED_EDGE ( 'NONE', *, *, #16517, .T. ) ;
#32490=CARTESIAN_POINT ( 'NONE',  ( -40.80097511801616150, 8.246641009394465982, 54.54930799450051637 ) ) ;
#32492=EDGE_CURVE ( 'NONE', #19917, #23906, #15021, .T. ) ;
#32523=COLOUR_RGB('Sky Blue',0.24,0.69,0.87);
#32524=FILL_AREA_STYLE_COLOUR('',#32523);
#32525=FILL_AREA_STYLE('',(#32524));
#32526=SURFACE_STYLE_FILL_AREA(#32525);
#32527=SURFACE_SIDE_STYLE('',(#32526));
#32528=SURFACE_STYLE_USAGE(.BOTH.,#32527);
#32529=PRESENTATION_STYLE_ASSIGNMENT((#32528));
ENDSEC;
END-ISO-10303-21;
